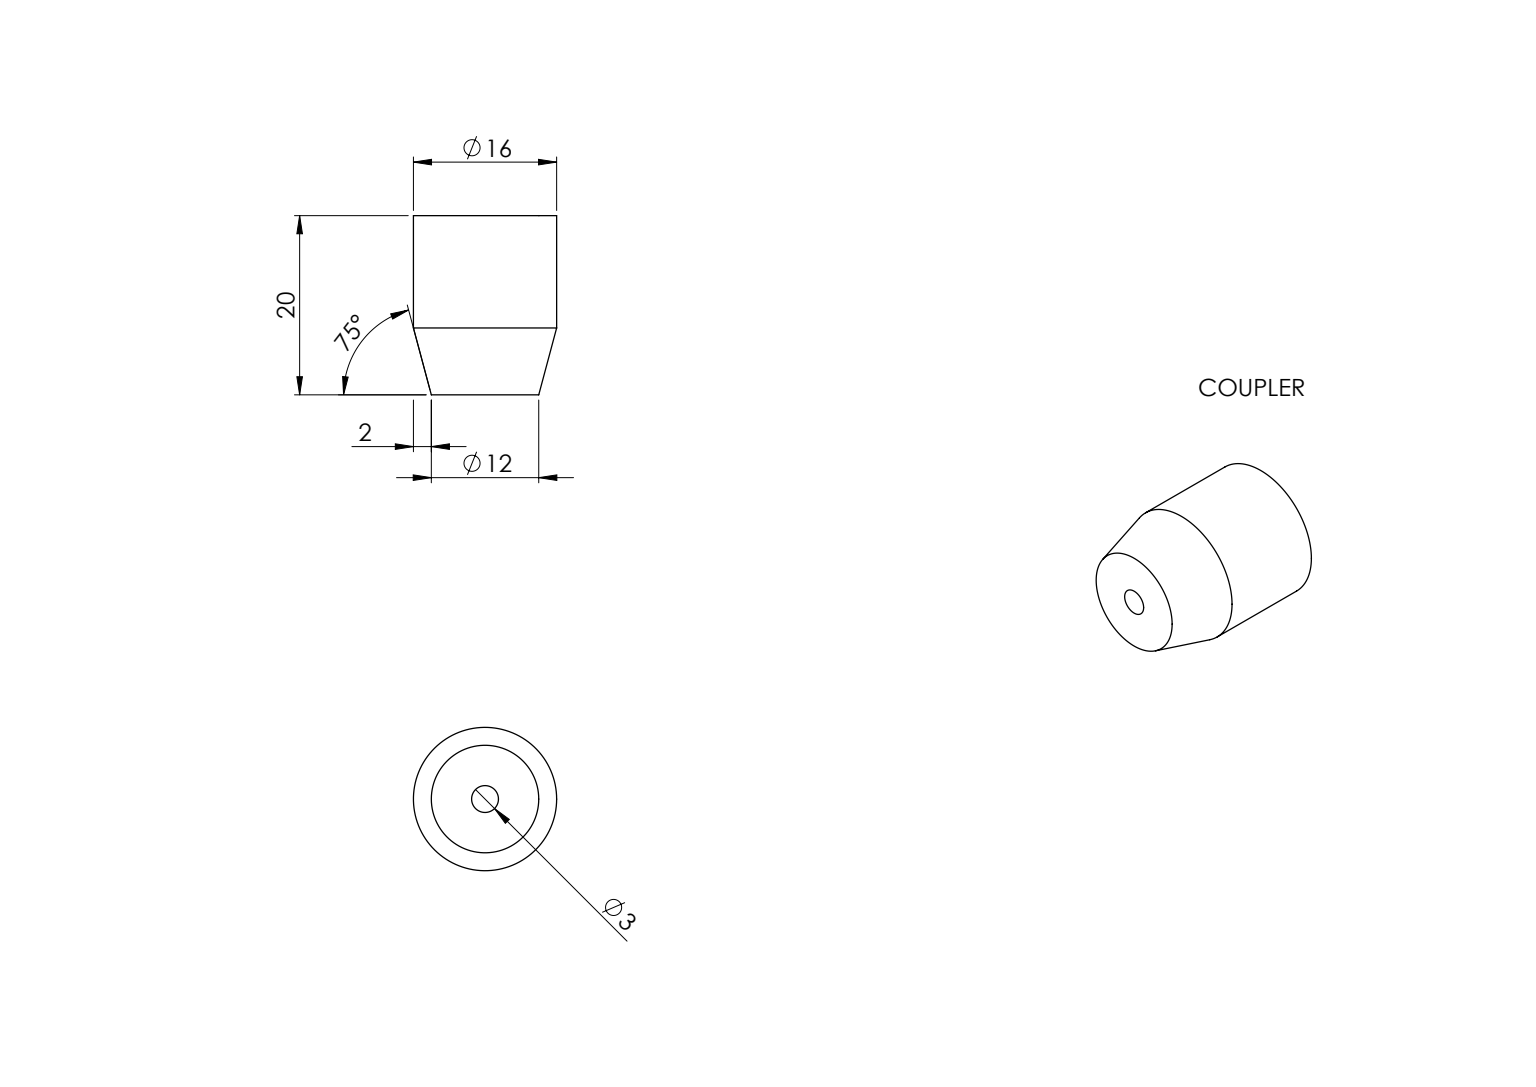
ISO-10303-21;
HEADER;
FILE_DESCRIPTION (('STEP AP214'),
    '1' );
FILE_NAME ('coupler.step',
    '2026-10-31T03:36:27',
    ( '' ),
    ( '' ),
    'SwSTEP 2.0',
    'SolidWorks 2026',
    '' );
FILE_SCHEMA (( 'AUTOMOTIVE_DESIGN' ));
ENDSEC;

DATA;
#7=CARTESIAN_POINT ( 'NONE',  ( 10.56230152254411081, 0.000000000000000000, -0.3374999987710014526 ) ) ;
#8=DIRECTION ( 'NONE',  ( -1.000000000000000000, 0.000000000000000000, 0.000000000000000000 ) ) ;
#18=CARTESIAN_POINT ( 'NONE',  ( 19.68408634441911786, -5.407089921784861808, -9.046874999385529748 ) ) ;
#22=CARTESIAN_POINT ( 'NONE',  ( 13.44051670066911619, -5.407089921784865361, -3.721874999385532679 ) ) ;
#34=CARTESIAN_POINT ( 'NONE',  ( 16.56230152254410726, 0.000000000000000000, -10.00000000000000000 ) ) ;
#40=CARTESIAN_POINT ( 'NONE',  ( 13.56230152254411792, -5.196152422706638241, -4.875000000000101252 ) ) ;
#43=LINE ( 'NONE', #12559, #36906 ) ;
#57=CARTESIAN_POINT ( 'NONE',  ( 13.44051670066911441, -5.407089921784865361, -1.021874999385524729 ) ) ;
#68=CARTESIAN_POINT ( 'NONE',  ( 10.56230152254517307, 3.464101615138364565, -6.224999998771024501 ) ) ;
#79=EDGE_CURVE ( 'NONE', #19909, #6556, #23186, .T. ) ;
#81=CARTESIAN_POINT ( 'NONE',  ( 10.56230152254410726, 0.000000000000000000, -4.387499998770999277 ) ) ;
#94=CARTESIAN_POINT ( 'NONE',  ( 10.31873187879411269, 0.000000000000000000, -10.04062499938554431 ) ) ;
#97=CARTESIAN_POINT ( 'NONE',  ( 11.28998163430637725, -3.344369132205555317, -9.999999999999998224 ) ) ;
#108=CARTESIAN_POINT ( 'NONE',  ( 22.80587116629411781, -3.604726614523235284, -3.553124999385526728 ) ) ;
#125=CARTESIAN_POINT ( 'NONE',  ( 16.56230152254410726, 0.000000000000000000, -10.00000000000000000 ) ) ;
#128=EDGE_CURVE ( 'NONE', #11418, #35635, #36670, .T. ) ;
#135=ADVANCED_FACE ( 'NONE', ( #36144 ), #26701, .T. ) ;
#136=EDGE_LOOP ( 'NONE', ( #21590, #33549, #31769, #19071 ) ) ;
#142=CARTESIAN_POINT ( 'NONE',  ( 13.44051670066910908, 5.407089921784862696, -9.721874999385510918 ) ) ;
#155=LINE ( 'NONE', #26123, #10199 ) ;
#162=ORIENTED_EDGE ( 'NONE', *, *, #30521, .T. ) ;
#172=CARTESIAN_POINT ( 'NONE',  ( 19.68408634441911076, 5.407089921784857367, -4.790624999385539873 ) ) ;
#179=CARTESIAN_POINT ( 'NONE',  ( 10.56230152254411259, 3.464101615137752166, -4.874999998771025744 ) ) ;
#195=EDGE_CURVE ( 'NONE', #23387, #15078, #25492, .T. ) ;
#201=SHAPE_REPRESENTATION ( 'coupler', ( #17215 ), #24466 ) ;
#205=VERTEX_POINT ( 'NONE', #8495 ) ;
#208=CARTESIAN_POINT ( 'NONE',  ( 16.56230152254411436, 7.209453229046482114, -8.859374999385529748 ) ) ;
#213=CARTESIAN_POINT ( 'NONE',  ( 19.68408634441912142, -5.407089921784861808, -3.646874999385540939 ) ) ;
#222=EDGE_LOOP ( 'NONE', ( #9327, #12339, #21719, #21080 ) ) ;
#231=CARTESIAN_POINT ( 'NONE',  ( 10.56230152254410726, 0.000000000000000000, -3.600000000000047606 ) ) ;
#247=CARTESIAN_POINT ( 'NONE',  ( 19.68408634441911076, 5.407089921784862696, -2.146874999385511629 ) ) ;
#279=CARTESIAN_POINT ( 'NONE',  ( 22.80587116629410716, 7.646167579472015790E-16, -9.365624999385563143 ) ) ;
#285=DIRECTION ( 'NONE',  ( 1.000000000000000000, 0.000000000000000000, 0.000000000000000000 ) ) ;
#292=CARTESIAN_POINT ( 'NONE',  ( 10.31873187879411269, 3.604726614523236616, -4.228124999385536320 ) ) ;
#313=AXIS2_PLACEMENT_3D ( 'NONE', #22514, #37081, #34061 ) ;
#319=EDGE_LOOP ( 'NONE', ( #2535, #440, #17456, #4187 ) ) ;
#326=CARTESIAN_POINT ( 'NONE',  ( 13.44051670066911264, -5.407089921784865361, -10.02187499938553294 ) ) ;
#328=CARTESIAN_POINT ( 'NONE',  ( 13.44051670066911441, 5.407089921784856479, -2.915624999385552307 ) ) ;
#342=CARTESIAN_POINT ( 'NONE',  ( 10.56230152254331323, 3.464101615137297419, -9.037500000000031619 ) ) ;
#359=CARTESIAN_POINT ( 'NONE',  ( 22.80587116629411071, 3.604726614523238837, -5.728124999385511451 ) ) ;
#364=CARTESIAN_POINT ( 'NONE',  ( 10.56230152254410726, 0.000000000000000000, -4.387499998770999277 ) ) ;
#383=CARTESIAN_POINT ( 'NONE',  ( 22.56230152254385501, 3.464101615137912926, -7.837500000000038547 ) ) ;
#386=CARTESIAN_POINT ( 'NONE',  ( 22.56230152254410370, 0.000000000000000000, -10.00000000000000000 ) ) ;
#389=ORIENTED_EDGE ( 'NONE', *, *, #10539, .F. ) ;
#395=ORIENTED_EDGE ( 'NONE', *, *, #6389, .F. ) ;
#396=CARTESIAN_POINT ( 'NONE',  ( 10.31873187879411269, 3.604726614523240613, -4.284374999385516247 ) ) ;
#415=CARTESIAN_POINT ( 'NONE',  ( 16.56230152254411081, 6.928203230275514990, -3.712500000000020339 ) ) ;
#418=CARTESIAN_POINT ( 'NONE',  ( 10.56230152254458865, 3.464101615138028389, -5.324999998771027698 ) ) ;
#434=CARTESIAN_POINT ( 'NONE',  ( 10.31873187879410736, 3.604726614523240613, -1.584374999385509630 ) ) ;
#440=ORIENTED_EDGE ( 'NONE', *, *, #16671, .T. ) ;
#453=LINE ( 'NONE', #37417, #32490 ) ;
#457=CARTESIAN_POINT ( 'NONE',  ( 10.56230152254384080, 3.464101615137603396, -9.937499999999992895 ) ) ;
#464=DIRECTION ( 'NONE',  ( 0.000000000000000000, 0.000000000000000000, 1.000000000000000000 ) ) ;
#465=CARTESIAN_POINT ( 'NONE',  ( 10.31873187879411091, -3.604726614523240613, -8.653124999385532590 ) ) ;
#478=CARTESIAN_POINT ( 'NONE',  ( 10.31873187879411091, -3.604726614523240613, -5.053124999385533833 ) ) ;
#495=DIRECTION ( 'NONE',  ( 1.000000000000000000, 0.000000000000000000, 0.000000000000000000 ) ) ;
#501=CARTESIAN_POINT ( 'NONE',  ( 22.56230152254543597, 3.464101615136989665, -4.574999998771033916 ) ) ;
#510=CARTESIAN_POINT ( 'NONE',  ( 13.44051670066911441, -5.407089921784859143, -1.865624999385528948 ) ) ;
#514=DIRECTION ( 'NONE',  ( 1.000000000000000000, 0.000000000000000000, -0.000000000000000000 ) ) ;
#524=FACE_OUTER_BOUND ( 'NONE', #7081, .T. ) ;
#537=( BOUNDED_CURVE ( )  B_SPLINE_CURVE ( 2, ( #9361, #68, #20936, #11634, #17898, #12007, #35307 ),
 .UNSPECIFIED., .F., .F. ) 
 B_SPLINE_CURVE_WITH_KNOTS ( ( 3, 2, 2, 3 ),
 ( 0.5652173913043500031, 0.5724637681159433500, 0.5797101449275368079, 0.5869565217391301548 ),
 .UNSPECIFIED. ) 
 CURVE ( )  GEOMETRIC_REPRESENTATION_ITEM ( )  RATIONAL_B_SPLINE_CURVE ( ( 0.9999999999999589217, 0.8660254037844797859, 1.000000000000000000, 0.8660254037844387076, 1.000000000000000000, 0.8660254037844448138, 0.9999999999999938938 ) ) 
 REPRESENTATION_ITEM ( '' )  );
#541=CARTESIAN_POINT ( 'NONE',  ( 10.31873187879411269, -3.604726614523240613, -4.603124999385506122 ) ) ;
#546=CARTESIAN_POINT ( 'NONE',  ( 13.56230152254410548, 5.196152422706630247, -5.812499998771008869 ) ) ;
#568=CARTESIAN_POINT ( 'NONE',  ( 22.80587116629411071, 3.604726614523238837, -0.7781249993855585689 ) ) ;
#571=ORIENTED_EDGE ( 'NONE', *, *, #36630, .T. ) ;
#578=CARTESIAN_POINT ( 'NONE',  ( 22.80587116629412492, 3.604726614523243278, -3.984374999385507987 ) ) ;
#579=EDGE_LOOP ( 'NONE', ( #18982, #34697, #20451, #16198 ) ) ;
#598=CARTESIAN_POINT ( 'NONE',  ( 13.56230152254411614, -5.196152422706638241, -5.775000000000085620 ) ) ;
#602=LINE ( 'NONE', #31703, #10891 ) ;
#606=CARTESIAN_POINT ( 'NONE',  ( 22.56625951594015689, -0.6522502533381772105, -10.00000000000000000 ) ) ;
#616=CARTESIAN_POINT ( 'NONE',  ( 19.68408634441911431, 5.407089921784862696, -0.7968749993855217539 ) ) ;
#639=CARTESIAN_POINT ( 'NONE',  ( 19.56230152254412147, 5.196152422706637353, -0.6000000000000171863 ) ) ;
#650=CARTESIAN_POINT ( 'NONE',  ( 10.31873187879411091, -3.604726614523240613, -9.553124999385522287 ) ) ;
#657=ORIENTED_EDGE ( 'NONE', *, *, #10356, .T. ) ;
#661=CARTESIAN_POINT ( 'NONE',  ( 13.44051670066911619, -5.407089921784859143, -5.015624999385570604 ) ) ;
#667=ORIENTED_EDGE ( 'NONE', *, *, #34152, .T. ) ;
#698=CARTESIAN_POINT ( 'NONE',  ( 19.68408634441910721, -5.407089921784855591, -1.790624999385564964 ) ) ;
#727=CARTESIAN_POINT ( 'NONE',  ( 22.80587116629410716, 7.646167579472015790E-16, -5.765624999385543958 ) ) ;
#735=CARTESIAN_POINT ( 'NONE',  ( 16.56230152254410726, -6.928203230275506996, -5.624999998770996434 ) ) ;
#740=CARTESIAN_POINT ( 'NONE',  ( 19.68408634441911786, -5.407089921784861808, -4.996874999385530813 ) ) ;
#742=CARTESIAN_POINT ( 'NONE',  ( 22.56230152254410015, 7.347880794884117764E-16, -7.312499998771010645 ) ) ;
#754=CARTESIAN_POINT ( 'NONE',  ( 16.56230152254411436, -6.928203230275514990, -4.837499999999994138 ) ) ;
#756=CARTESIAN_POINT ( 'NONE',  ( 22.56230152254500254, 3.464101615137234358, -5.924999998771016685 ) ) ;
#771=CARTESIAN_POINT ( 'NONE',  ( 10.31873187879410736, -3.604726614523244610, -3.309374999385498395 ) ) ;
#791=CARTESIAN_POINT ( 'NONE',  ( 13.56230152254410726, 5.196152422706636465, -6.375000000000019540 ) ) ;
#792=ORIENTED_EDGE ( 'NONE', *, *, #29984, .F. ) ;
#800=CARTESIAN_POINT ( 'NONE',  ( 10.56230152254594756, 3.464101615138813095, -1.274999998771018772 ) ) ;
#808=CARTESIAN_POINT ( 'NONE',  ( 22.80587116629411781, -3.604726614523238837, -4.509374999385530103 ) ) ;
#822=CARTESIAN_POINT ( 'NONE',  ( 19.68408634441910365, -5.407089921784855591, -0.8906249993855530622 ) ) ;
#831=CARTESIAN_POINT ( 'NONE',  ( 16.56230152254411436, 6.928203230275506996, -0.8999999987709939031 ) ) ;
#837=CARTESIAN_POINT ( 'NONE',  ( 21.95617849068234761, 3.814046910745170660, -9.967423460872726793 ) ) ;
#841=( BOUNDED_CURVE ( )  B_SPLINE_CURVE ( 2, ( #13122, #26953, #12745, #33021, #24313, #35856, #23936 ),
 .UNSPECIFIED., .F., .F. ) 
 B_SPLINE_CURVE_WITH_KNOTS ( ( 3, 2, 2, 3 ),
 ( 0.5434782608695670758, 0.5507246376811614219, 0.5579710144927557680, 0.5652173913043500031 ),
 .UNSPECIFIED. ) 
 CURVE ( )  GEOMETRIC_REPRESENTATION_ITEM ( )  RATIONAL_B_SPLINE_CURVE ( ( 0.9999999999999651390, 0.8660254037844735686, 1.000000000000000000, 0.8660254037844387076, 1.000000000000000000, 0.8660254037843976294, 1.000000000000041078 ) ) 
 REPRESENTATION_ITEM ( '' )  );
#853=DIRECTION ( 'NONE',  ( 0.000000000000000000, 0.000000000000000000, 1.000000000000000000 ) ) ;
#854=CARTESIAN_POINT ( 'NONE',  ( 13.44051670066911086, 5.407089921784856479, -6.965624999385521932 ) ) ;
#856=LINE ( 'NONE', #4264, #19603 ) ;
#861=ORIENTED_EDGE ( 'NONE', *, *, #9647, .T. ) ;
#863=DIRECTION ( 'NONE',  ( 0.000000000000000000, 0.000000000000000000, 1.000000000000000000 ) ) ;
#868=CARTESIAN_POINT ( 'NONE',  ( 10.56230152254410726, 0.000000000000000000, -5.850000000000049383 ) ) ;
#890=CARTESIAN_POINT ( 'NONE',  ( 13.44051670066911264, -5.407089921784859143, -2.765624999385540850 ) ) ;
#901=CARTESIAN_POINT ( 'NONE',  ( 10.56230152254374310, -3.464101615137546109, -6.712500000000007461 ) ) ;
#912=EDGE_LOOP ( 'NONE', ( #20316, #5565, #15559, #5000 ) ) ;
#923=CARTESIAN_POINT ( 'NONE',  ( 13.44051670066911086, 5.407089921784856479, -4.715624999385548577 ) ) ;
#929=CARTESIAN_POINT ( 'NONE',  ( 16.56230152254411081, -6.928203230275506996, -5.174999998771001586 ) ) ;
#932=AXIS2_PLACEMENT_3D ( 'NONE', #8550, #25977, #8 ) ;
#933=CARTESIAN_POINT ( 'NONE',  ( 16.56230152254411436, 7.209453229046482114, -4.809374999385505944 ) ) ;
#945=CARTESIAN_POINT ( 'NONE',  ( 10.56230152254410726, 0.000000000000000000, -7.650000000000045652 ) ) ;
#960=CARTESIAN_POINT ( 'NONE',  ( 22.80587116629411426, 7.646167579472024665E-16, -6.721874999385535787 ) ) ;
#968=CARTESIAN_POINT ( 'NONE',  ( 22.56230152254411792, 7.347880794884125653E-16, -5.625000000000018652 ) ) ;
#975=AXIS2_PLACEMENT_3D ( 'NONE', #33240, #22432, #7279 ) ;
#979=CARTESIAN_POINT ( 'NONE',  ( 22.56230152254412502, -3.464101615137755275, -7.012500000000041922 ) ) ;
#983=CARTESIAN_POINT ( 'NONE',  ( 22.56230152254410726, 7.347880794884117764E-16, -9.562499998771039955 ) ) ;
#988=CARTESIAN_POINT ( 'NONE',  ( 22.39561461052787195, -1.640876061562029031, -9.999999999999998224 ) ) ;
#990=DIRECTION ( 'NONE',  ( 1.000000000000000000, 0.000000000000000000, 0.000000000000000000 ) ) ;
#996=CARTESIAN_POINT ( 'NONE',  ( 19.68408634441912142, -5.407089921784861808, -2.746874999385529037 ) ) ;
#1037=ORIENTED_EDGE ( 'NONE', *, *, #23070, .T. ) ;
#1041=CARTESIAN_POINT ( 'NONE',  ( 22.80587116629411071, 3.604726614523238837, -6.178124999385540050 ) ) ;
#1049=CARTESIAN_POINT ( 'NONE',  ( 16.56230152254411436, -6.928203230275514990, -3.937500000000034639 ) ) ;
#1055=CARTESIAN_POINT ( 'NONE',  ( 13.56230152254410370, 5.196152422706630247, -4.912499998770996967 ) ) ;
#1079=CARTESIAN_POINT ( 'NONE',  ( 22.80587116629410716, 7.646167579472015790E-16, -3.965624999385547689 ) ) ;
#1088=ORIENTED_EDGE ( 'NONE', *, *, #15863, .T. ) ;
#1111=CARTESIAN_POINT ( 'NONE',  ( 19.68408634441910721, -5.407089921784855591, -8.090624999385564564 ) ) ;
#1118=CARTESIAN_POINT ( 'NONE',  ( 10.56230152254411614, -3.464101615137757051, -6.149999998770987020 ) ) ;
#1119=CARTESIAN_POINT ( 'NONE',  ( 10.56230152254410903, 7.347880794884117764E-16, -10.00000000000000000 ) ) ;
#1121=CARTESIAN_POINT ( 'NONE',  ( 10.31873187879410736, 0.000000000000000000, -3.346874999385518468 ) ) ;
#1134=CARTESIAN_POINT ( 'NONE',  ( 10.56230152254490484, 3.464101615138212242, -5.774999998771026988 ) ) ;
#1149=CARTESIAN_POINT ( 'NONE',  ( 16.56230152254411792, -7.209453229046482114, -5.484374999385515537 ) ) ;
#1154=EDGE_CURVE ( 'NONE', #28711, #31946, #29357, .T. ) ;
#1169=CARTESIAN_POINT ( 'NONE',  ( 22.56230152254411792, 7.347880794884125653E-16, -7.425000000000042455 ) ) ;
#1184=CARTESIAN_POINT ( 'NONE',  ( 19.68408634441910721, 5.407089921784862696, -3.046874999385523530 ) ) ;
#1201=CARTESIAN_POINT ( 'NONE',  ( 22.56230152254410370, 7.347880794884117764E-16, -1.012499998771038134 ) ) ;
#1213=CARTESIAN_POINT ( 'NONE',  ( 22.56230152254411792, 7.347880794884125653E-16, -2.475000000000060485 ) ) ;
#1225=CARTESIAN_POINT ( 'NONE',  ( 13.44051670066911619, -5.407089921784859143, -6.815624999385539340 ) ) ;
#1250=ADVANCED_FACE ( 'NONE', ( #23225 ), #9190, .F. ) ;
#1263=CARTESIAN_POINT ( 'NONE',  ( 22.80587116629410716, 7.646167579472015790E-16, -4.415624999385525662 ) ) ;
#1265=CARTESIAN_POINT ( 'NONE',  ( 16.56230152254410726, 0.000000000000000000, 10.00000000000000000 ) ) ;
#1272=CARTESIAN_POINT ( 'NONE',  ( 16.56230152254410726, 0.000000000000000000, 10.00000000000000000 ) ) ;
#1287=CARTESIAN_POINT ( 'NONE',  ( 22.56230152254410726, 7.347880794884117764E-16, -9.112499998771033560 ) ) ;
#1288=EDGE_CURVE ( 'NONE', #21775, #13344, #22888, .T. ) ;
#1296=CARTESIAN_POINT ( 'NONE',  ( 19.68408634441910721, 5.407089921784857367, -8.390624999385531524 ) ) ;
#1297=( BOUNDED_CURVE ( )  B_SPLINE_CURVE ( 2, ( #36397, #25222, #16702, #28423, #36212, #7793, #8169 ),
 .UNSPECIFIED., .F., .F. ) 
 B_SPLINE_CURVE_WITH_KNOTS ( ( 3, 2, 2, 3 ),
 ( 0.2173913043478289675, 0.2246376811594223422, 0.2318840579710157446, 0.2391304347826091192 ),
 .UNSPECIFIED. ) 
 CURVE ( )  GEOMETRIC_REPRESENTATION_ITEM ( )  RATIONAL_B_SPLINE_CURVE ( ( 0.9999999999999465983, 0.8660254037844921093, 1.000000000000000000, 0.8660254037844387076, 1.000000000000000000, 0.8660254037844310471, 1.000000000000007772 ) ) 
 REPRESENTATION_ITEM ( '' )  );
#1301=CIRCLE ( 'NONE', #23716, 5.999999999999998224 ) ;
#1303=CARTESIAN_POINT ( 'NONE',  ( 22.56230152254410015, 7.347880794884117764E-16, -7.762499998770988618 ) ) ;
#1308=CARTESIAN_POINT ( 'NONE',  ( 22.80587116629411781, -3.604726614523238837, -4.509374999385530103 ) ) ;
#1327=CARTESIAN_POINT ( 'NONE',  ( 16.56230152254410726, -7.209453229046475009, -3.178124999385525395 ) ) ;
#1339=CARTESIAN_POINT ( 'NONE',  ( 16.56230152254411081, 7.209453229046482114, -5.709374999385496530 ) ) ;
#1340=VERTEX_POINT ( 'NONE', #32484 ) ;
#1346=( NAMED_UNIT ( * ) SI_UNIT ( $, .STERADIAN. ) SOLID_ANGLE_UNIT ( ) );
#1361=CARTESIAN_POINT ( 'NONE',  ( 16.56230152254411436, -6.928203230275514990, -7.987500000000027356 ) ) ;
#1363=ORIENTED_EDGE ( 'NONE', *, *, #4409, .T. ) ;
#1378=CARTESIAN_POINT ( 'NONE',  ( 19.68408634441911431, 5.407089921784862696, -4.846874999385547333 ) ) ;
#1392=CARTESIAN_POINT ( 'NONE',  ( 16.56230152254410726, 0.000000000000000000, 0.000000000000000000 ) ) ;
#1399=CARTESIAN_POINT ( 'NONE',  ( 13.56230152254410903, 5.196152422706636465, -0.5250000000000532019 ) ) ;
#1404=CARTESIAN_POINT ( 'NONE',  ( 16.56230152254411081, 6.928203230275506996, -8.549999998770985599 ) ) ;
#1415=CARTESIAN_POINT ( 'NONE',  ( 10.31873187879411091, 0.000000000000000000, -7.340624999385508609 ) ) ;
#1455=CARTESIAN_POINT ( 'NONE',  ( 16.56230152254411081, 7.209453229046475009, -3.403124999385538807 ) ) ;
#1457=LINE ( 'NONE', #35951, #26756 ) ;
#1460=CARTESIAN_POINT ( 'NONE',  ( 15.26155779561005232, -6.106572496351636126, -10.00000000000000000 ) ) ;
#1486=CARTESIAN_POINT ( 'NONE',  ( 10.31873187879411091, 3.604726614523236616, -7.828124999385534188 ) ) ;
#1491=CARTESIAN_POINT ( 'NONE',  ( 22.56230152254410370, 7.347880794884117764E-16, -8.662499998771028942 ) ) ;
#1494=CARTESIAN_POINT ( 'NONE',  ( 22.80587116629412847, -3.604726614523238837, -5.409374999385520688 ) ) ;
#1522=ORIENTED_EDGE ( 'NONE', *, *, #16803, .T. ) ;
#1523=CARTESIAN_POINT ( 'NONE',  ( 13.44051670066910908, 5.407089921784862696, -7.021874999385530280 ) ) ;
#1527=CARTESIAN_POINT ( 'NONE',  ( 19.68408634441910721, 5.407089921784857367, -1.190624999385520022 ) ) ;
#1532=CARTESIAN_POINT ( 'NONE',  ( 19.56230152254411081, -5.196152422706629359, -9.637499998771032139 ) ) ;
#1536=CARTESIAN_POINT ( 'NONE',  ( 10.56230152254410903, 0.000000000000000000, -1.237499998771041110 ) ) ;
#1537=ORIENTED_EDGE ( 'NONE', *, *, #3843, .T. ) ;
#1546=CARTESIAN_POINT ( 'NONE',  ( 13.56230152254411792, -5.196152422706638241, -9.375000000000078160 ) ) ;
#1561=CARTESIAN_POINT ( 'NONE',  ( 10.31873187879410736, 0.000000000000000000, -5.596874999385520688 ) ) ;
#1588=CARTESIAN_POINT ( 'NONE',  ( 16.56230152254411436, 6.928203230275514990, -3.262500000000057021 ) ) ;
#1606=CARTESIAN_POINT ( 'NONE',  ( 10.31873187879410736, 0.000000000000000000, -6.890624999385530636 ) ) ;
#1608=CARTESIAN_POINT ( 'NONE',  ( 13.56230152254411259, -5.196152422706632912, -2.512499998771011711 ) ) ;
#1613=ORIENTED_EDGE ( 'NONE', *, *, #16584, .F. ) ;
#1625=DIRECTION ( 'NONE',  ( 0.000000000000000000, 0.000000000000000000, 1.000000000000000000 ) ) ;
#1645=CARTESIAN_POINT ( 'NONE',  ( 13.44051670066911086, 5.407089921784856479, -4.715624999385548577 ) ) ;
#1649=CARTESIAN_POINT ( 'NONE',  ( 19.68408634441911786, -5.407089921784861808, -9.496874999385534366 ) ) ;
#1654=CARTESIAN_POINT ( 'NONE',  ( 10.31873187879410381, 3.604726614523240613, -0.2343749993854903346 ) ) ;
#1656=ORIENTED_EDGE ( 'NONE', *, *, #14505, .T. ) ;
#1661=DIRECTION ( 'NONE',  ( 1.000000000000000000, 0.000000000000000000, 0.000000000000000000 ) ) ;
#1675=CARTESIAN_POINT ( 'NONE',  ( 19.68408634441910721, -5.407089921784855591, -8.990624999385548932 ) ) ;
#1680=CARTESIAN_POINT ( 'NONE',  ( 22.56230152254409660, 3.464101615137755275, -9.074999998770975296 ) ) ;
#1683=CARTESIAN_POINT ( 'NONE',  ( 13.44051670066911264, -5.407089921784865361, -5.521874999385528504 ) ) ;
#1696=CARTESIAN_POINT ( 'NONE',  ( 22.56230152254410726, 7.347880794884117764E-16, -9.112499998771033560 ) ) ;
#1708=CARTESIAN_POINT ( 'NONE',  ( 22.56230152254403265, -3.464101615137814338, -0.2625000000000441980 ) ) ;
#1712=CARTESIAN_POINT ( 'NONE',  ( 13.44051670066911086, 5.407089921784862696, -5.671874999385540406 ) ) ;
#1721=( NAMED_UNIT ( * ) PLANE_ANGLE_UNIT ( ) SI_UNIT ( $, .RADIAN. ) );
#1722=CARTESIAN_POINT ( 'NONE',  ( 22.56230152254410015, 7.347880794884117764E-16, -2.812499998771006204 ) ) ;
#1725=CARTESIAN_POINT ( 'NONE',  ( 22.56230152254410015, 3.464101615137755275, -0.5249999987710241012 ) ) ;
#1729=CARTESIAN_POINT ( 'NONE',  ( 10.56230152254411081, 0.000000000000000000, -4.837499998771033205 ) ) ;
#1733=CARTESIAN_POINT ( 'NONE',  ( 19.56230152254412147, -5.196152422706635576, -9.300000000000057554 ) ) ;
#1752=CARTESIAN_POINT ( 'NONE',  ( 13.44051670066910908, 5.407089921784862696, -7.021874999385530280 ) ) ;
#1756=EDGE_LOOP ( 'NONE', ( #2378, #1797, #29965, #24577 ) ) ;
#1775=CARTESIAN_POINT ( 'NONE',  ( 10.56230152254411614, -3.464101615137761048, -1.312500000000054401 ) ) ;
#1783=DIRECTION ( 'NONE',  ( 0.000000000000000000, 0.000000000000000000, 1.000000000000000000 ) ) ;
#1793=CARTESIAN_POINT ( 'NONE',  ( 19.68408634441910721, 5.407089921784857367, -8.390624999385531524 ) ) ;
#1797=ORIENTED_EDGE ( 'NONE', *, *, #17252, .T. ) ;
#1829=CARTESIAN_POINT ( 'NONE',  ( 10.31873187879411091, -3.604726614523240613, -5.053124999385533833 ) ) ;
#1839=CARTESIAN_POINT ( 'NONE',  ( 13.44051670066910908, 5.407089921784862696, -2.071874999385547866 ) ) ;
#1847=EDGE_CURVE ( 'NONE', #16024, #17042, #30597, .T. ) ;
#1860=CARTESIAN_POINT ( 'NONE',  ( 13.44051670066911264, 5.407089921784856479, -8.315624999385541116 ) ) ;
#1865=CARTESIAN_POINT ( 'NONE',  ( 22.56230152254410015, 7.347880794884117764E-16, -8.212499998771022547 ) ) ;
#1866=( BOUNDED_CURVE ( )  B_SPLINE_CURVE ( 2, ( #29614, #800, #33026, #3650, #4213, #18453, #15219 ),
 .UNSPECIFIED., .F., .F. ) 
 B_SPLINE_CURVE_WITH_KNOTS ( ( 3, 2, 2, 3 ),
 ( 0.08695652173913427652, 0.09420289855072766505, 0.1014492753623210397, 0.1086956521739144144 ),
 .UNSPECIFIED. ) 
 CURVE ( )  GEOMETRIC_REPRESENTATION_ITEM ( )  RATIONAL_B_SPLINE_CURVE ( ( 0.9999999999999289457, 0.8660254037845097619, 1.000000000000000000, 0.8660254037844387076, 1.000000000000000000, 0.8660254037844132835, 1.000000000000025313 ) ) 
 REPRESENTATION_ITEM ( '' )  );
#1870=CARTESIAN_POINT ( 'NONE',  ( 13.44051670066911264, -5.407089921784865361, -5.971874999385562433 ) ) ;
#1874=CYLINDRICAL_SURFACE ( 'NONE', #4361, 1.500000000000001332 ) ;
#1877=DIRECTION ( 'NONE',  ( 0.000000000000000000, 0.000000000000000000, 1.000000000000000000 ) ) ;
#1899=CARTESIAN_POINT ( 'NONE',  ( 22.80587116629412492, -3.604726614523238837, -7.659374999385499372 ) ) ;
#1900=ORIENTED_EDGE ( 'NONE', *, *, #29749, .F. ) ;
#1910=CARTESIAN_POINT ( 'NONE',  ( 16.56230152254411436, 6.928203230275506996, -0.4499999987709982219 ) ) ;
#1917=CARTESIAN_POINT ( 'NONE',  ( 22.56230152254412147, -3.464101615137755275, -9.712500000000016342 ) ) ;
#1924=CYLINDRICAL_SURFACE ( 'NONE', #15961, 5.999999999999998224 ) ;
#1934=CARTESIAN_POINT ( 'NONE',  ( 19.68408634441911431, -5.407089921784861808, -6.346874999385549110 ) ) ;
#1939=CARTESIAN_POINT ( 'NONE',  ( 19.68408634441911431, -5.407089921784861808, -0.4968749993855270386 ) ) ;
#1943=PRODUCT_CONTEXT ( 'NONE', #19027, 'mechanical' ) ;
#1958=CARTESIAN_POINT ( 'NONE',  ( 13.56230152254410726, 5.196152422706636465, -1.875000000000043299 ) ) ;
#1971=ORIENTED_EDGE ( 'NONE', *, *, #25981, .F. ) ;
#1972=CARTESIAN_POINT ( 'NONE',  ( 22.56230152254492438, -3.464101615137295642, -7.012500000000033040 ) ) ;
#1976=CARTESIAN_POINT ( 'NONE',  ( 13.44051670066911619, -5.407089921784859143, -9.515624999385547511 ) ) ;
#1986=DIRECTION ( 'NONE',  ( 0.000000000000000000, 0.000000000000000000, 1.000000000000000000 ) ) ;
#2009=DIRECTION ( 'NONE',  ( 0.000000000000000000, 0.000000000000000000, 1.000000000000000000 ) ) ;
#2014=CARTESIAN_POINT ( 'NONE',  ( 22.80587116629410360, 7.646167579472015790E-16, -7.115624999385533833 ) ) ;
#2020=CARTESIAN_POINT ( 'NONE',  ( 10.56230152254410548, 0.000000000000000000, -6.750000000000061284 ) ) ;
#2022=CARTESIAN_POINT ( 'NONE',  ( 22.80587116629411426, 7.646167579472024665E-16, -1.771874999385525395 ) ) ;
#2029=CARTESIAN_POINT ( 'NONE',  ( 19.68408634441910365, -5.407089921784855591, -0.8906249993855530622 ) ) ;
#2046=CARTESIAN_POINT ( 'NONE',  ( 16.56230152254411436, -7.209453229046475009, -9.928124999385525840 ) ) ;
#2053=CARTESIAN_POINT ( 'NONE',  ( 22.56230152254409660, 3.464101615137755275, -9.524999998771003007 ) ) ;
#2057=CARTESIAN_POINT ( 'NONE',  ( 10.31873187879411091, 3.604726614523240613, -9.684374999385527261 ) ) ;
#2058=CARTESIAN_POINT ( 'NONE',  ( 22.80587116629411781, -3.604726614523238837, -7.209374999385536498 ) ) ;
#2074=CARTESIAN_POINT ( 'NONE',  ( 10.56230152254410903, 0.000000000000000000, -2.250000000000057732 ) ) ;
#2083=CYLINDRICAL_SURFACE ( 'NONE', #16524, 5.999999999999998224 ) ;
#2089=CARTESIAN_POINT ( 'NONE',  ( 22.80587116629411781, -3.604726614523238837, -8.109374999385527971 ) ) ;
#2099=CARTESIAN_POINT ( 'NONE',  ( 13.56230152254410548, 5.196152422706630247, -1.312499998771005094 ) ) ;
#2102=CARTESIAN_POINT ( 'NONE',  ( 16.56230152254411081, -6.928203230275514990, -8.887500000000020606 ) ) ;
#2106=CARTESIAN_POINT ( 'NONE',  ( 13.56230152254410548, 5.196152422706636465, -9.975000000000012079 ) ) ;
#2121=CARTESIAN_POINT ( 'NONE',  ( 16.56230152254411436, 7.209453229046482114, -5.259374999385500793 ) ) ;
#2127=CARTESIAN_POINT ( 'NONE',  ( 22.80587116629411781, 7.646167579472024665E-16, -0.4218749993855352987 ) ) ;
#2128=CARTESIAN_POINT ( 'NONE',  ( 10.56230152254410903, 0.000000000000000000, -5.737499998771017573 ) ) ;
#2144=CARTESIAN_POINT ( 'NONE',  ( 10.56230152254410726, 0.000000000000000000, -1.350000000000045608 ) ) ;
#2161=CARTESIAN_POINT ( 'NONE',  ( 19.68408634441910721, -5.407089921784855591, -9.440624999385555327 ) ) ;
#2165=EDGE_CURVE ( 'NONE', #205, #18251, #37105, .T. ) ;
#2168=ORIENTED_EDGE ( 'NONE', *, *, #25401, .F. ) ;
#2171=CARTESIAN_POINT ( 'NONE',  ( 22.56230152254410726, 7.347880794884117764E-16, -3.262499998771012599 ) ) ;
#2198=CARTESIAN_POINT ( 'NONE',  ( 19.68408634441910721, 5.407089921784857367, -5.690624999385579308 ) ) ;
#2207=CARTESIAN_POINT ( 'NONE',  ( 10.31873187879410736, -3.604726614523244610, -1.509374999385515670 ) ) ;
#2209=VERTEX_POINT ( 'NONE', #32966 ) ;
#2213=CARTESIAN_POINT ( 'NONE',  ( 16.56230152254411436, 7.209453229046475009, -2.053124999385520066 ) ) ;
#2218=EDGE_LOOP ( 'NONE', ( #26929, #14715, #15035, #29987 ) ) ;
#2232=CARTESIAN_POINT ( 'NONE',  ( 22.80587116629410716, 7.646167579472015790E-16, -9.365624999385563143 ) ) ;
#2238=CARTESIAN_POINT ( 'NONE',  ( 10.56230152254411259, -3.464101615137757051, -10.19999999877101082 ) ) ;
#2241=CARTESIAN_POINT ( 'NONE',  ( 10.31873187879411091, -3.604726614523244610, -9.609374999385535077 ) ) ;
#2242=CARTESIAN_POINT ( 'NONE',  ( 16.56230152254411436, -7.209453229046482114, -5.934374999385510385 ) ) ;
#2248=CYLINDRICAL_SURFACE ( 'NONE', #20898, 8.000000000000000000 ) ;
#2272=CARTESIAN_POINT ( 'NONE',  ( 22.80587116629412137, 7.646167579472024665E-16, -8.521874999385502747 ) ) ;
#2276=CARTESIAN_POINT ( 'NONE',  ( 13.44051670066911264, -5.407089921784859143, -2.765624999385540850 ) ) ;
#2282=CARTESIAN_POINT ( 'NONE',  ( 10.56230152254410903, 3.464101615137752166, -1.274999998770995679 ) ) ;
#2292=CARTESIAN_POINT ( 'NONE',  ( 19.68408634441910721, 5.407089921784857367, -0.2906249993855358760 ) ) ;
#2293=CYLINDRICAL_SURFACE ( 'NONE', #36650, 5.999999999999998224 ) ;
#2303=CARTESIAN_POINT ( 'NONE',  ( 22.56230152254390475, 3.464101615137881840, -3.787500000000044942 ) ) ;
#2311=CARTESIAN_POINT ( 'NONE',  ( 16.56230152254411436, 7.209453229046482114, -7.059374999385483740 ) ) ;
#2315=( BOUNDED_CURVE ( )  B_SPLINE_CURVE ( 2, ( #26791, #15432, #23962, #30909, #22012, #33566, #6519, #33750, #10623, #36582, #13286, #10250, #36206, #3671, #7417, #18988, #13100, #16511, #26981, #4562, #822, #35505, #16137, #19368, #22202, #24842, #28058, #15241, #1527, #32665, #13473, #36393, #25025, #7790, #6706, #10439, #24655, #18278, #7603, #30727, #16323, #18094, #29635, #9552, #29822, #28420, #3017, #17250, #20096, #37499, #16884, #26139, #34488, #36950, #25584, #11551, #22568, #10812, #31825, #31097, #22384, #8348, #5306, #23124, #33934, #37320, #7975, #22942, #16698, #31278, #2276, #20285, #11370, #8530, #14586, #34668, #8713, #25957, #2641, #37137, #11182, #28791, #28976, #5119, #19740, #2460, #5860, #31642, #28246, #19549, #34115, #19920, #5670, #2828, #28604, #13853, #14400, #25400, #10997, #17438, #8166, #14034, #14218, #22755, #34304, #31459, #25768, #5482, #17066, #23873, #26893, #20657, #26510, #21226, #15339, #29731, #15147, #35604, #32389, #541, #11923, #14963, #923, #23490, #172, #32766, #20473, #11739, #12492, #6429, #35041, #24059, #18190, #3765, #9650, #35412, #35227, #32012, #12107, #6802, #3202, #18003, #29546, #32204, #18377, #29927, #3955, #15530, #23309, #359, #727, #14778, #21038, #9276, #34855, #8895, #23680, #20848, #6043, #3584, #17629, #26697, #12299, #9462, #29159, #26322, #32575, #9088, #6239, #6615, #17816, #29354, #3394, #24433, #24617, #7193, #7743, #24799, #7006, #13249, #7561, #19327, #36538, #30864, #27270, #16282, #21972, #36164, #19136, #30118, #10581, #15910, #18576, #22160, #33704, #33335, #18946, #36350, #21600, #10019, #21784, #10395, #10210, #4889, #27086, #1486, #13060, #12678, #7375, #24977, #21412, #33149, #1111, #4148, #24248, #33517, #18764, #4703, #1860, #35792, #1296, #30684, #35983, #30500, #30306, #9834, #27830, #15720, #13429, #32954, #4521, #12867, #4330, #27458, #16095, #27648, #1675, #25542, #28013, #5440, #31781, #8669, #28561, #36728, #25728, #17022, #2232, #19695, #2418, #28382, #37094, #37281, #13812, #13991, #2602, #22898, #34625, #10767, #25359, #34073, #11510, #2046, #22339, #13625, #36904 ),
 .UNSPECIFIED., .F., .F. ) 
 B_SPLINE_CURVE_WITH_KNOTS ( ( 3, 2, 2, 2, 2, 2, 2, 2, 2, 2, 2, 2, 2, 2, 2, 2, 2, 2, 2, 2, 2, 2, 2, 2, 2, 2, 2, 2, 2, 2, 2, 2, 2, 2, 2, 2, 2, 2, 2, 2, 2, 2, 2, 2, 2, 2, 2, 2, 2, 2, 2, 2, 2, 2, 2, 2, 2, 2, 2, 2, 2, 2, 2, 2, 2, 2, 2, 2, 2, 2, 2, 2, 2, 2, 2, 2, 2, 2, 2, 2, 2, 2, 2, 2, 2, 2, 2, 2, 2, 2, 2, 2, 2, 2, 2, 2, 2, 2, 2, 2, 2, 2, 2, 2, 2, 2, 2, 2, 2, 2, 2, 2, 2, 2, 2, 2, 2, 2, 2, 2, 2, 2, 2, 2, 2, 2, 2, 2, 2, 2, 2, 2, 3 ),
 ( 0.000000000000000000, 0.007499808116169960973, 0.01499961623233992195, 0.02249942434850988118, 0.02999923246467984389, 0.03749904058084980313, 0.04499884869701976237, 0.05249865681318972854, 0.05999846492935968778, 0.06749827304552964702, 0.07499808116169960626, 0.08249788927786955162, 0.08999769739403952473, 0.09749750551020949785, 0.1049973136263794571, 0.1124971217425494163, 0.1199969298587193756, 0.1274967379748893348, 0.1349965460910592940, 0.1424963542072292533, 0.1499961623233992125, 0.1574959704395691995, 0.1649957785557391032, 0.1724955866719090902, 0.1799953947880790495, 0.1874952029042490087, 0.1949950110204189957, 0.2024948191365889549, 0.2099946272527589142, 0.2174944353689288457, 0.2249942434850988326, 0.2324940516012687641, 0.2399938597174387511, 0.2474936678336087381, 0.2549934759497786696, 0.2624932840659486288, 0.2699930921821185881, 0.2774929002982886028, 0.2849927084144585065, 0.2924925165306284103, 0.2999923246467984250, 0.3074921327629683843, 0.3149919408791383990, 0.3224917489953083582, 0.3299915571114782065, 0.3374913652276482212, 0.3449911733438181805, 0.3524909814599881952, 0.3599907895761580989, 0.3674905976923280582, 0.3749904058084980174, 0.3824902139246679766, 0.3899900220408379914, 0.3974898301570078951, 0.4049896382731779099, 0.4124894463893478136, 0.4199892545055178283, 0.4274890626216877321, 0.4349888707378576913, 0.4424886788540277061, 0.4499884869701976653, 0.4574882950863676245, 0.4649881032025375283, 0.4724879113187074875, 0.4799877194348775022, 0.4874875275510474615, 0.4949873356672174762, 0.5024871437833873244, 0.5099869518995573392, 0.5174867600157272429, 0.5249865681318972577, 0.5324863762480671614, 0.5399861843642371761, 0.5474859924804070799, 0.5549858005965772056, 0.5624856087127469983, 0.5699854168289170131, 0.5774852249450870278, 0.5849850330612568206, 0.5924848411774269463, 0.5999846492935968501, 0.6074844574097668648, 0.6149842655259367685, 0.6224840736421066723, 0.6299838817582767980, 0.6374836898744465907, 0.6449834979906167165, 0.6524833061067866202, 0.6599831142229564129, 0.6674829223391265387, 0.6749827304552964424, 0.6824825385714665682, 0.6899823466876363609, 0.6974821548038062646, 0.7049819629199763904, 0.7124817710361461831, 0.7199815791523161979, 0.7274813872684862126, 0.7349811953846561163, 0.7424810035008261311, 0.7499808116169960348, 0.7574806197331660496, 0.7649804278493359533, 0.7724802359655059680, 0.7799800440816759828, 0.7874798521978458865, 0.7949796603140157902, 0.8024794684301858050, 0.8099792765463558197, 0.8174790846625257235, 0.8249788927786956272, 0.8324787008948656419, 0.8399785090110356567, 0.8474783171272055604, 0.8549781252433754641, 0.8624779333595454789, 0.8699777414757153826, 0.8774775495918853974, 0.8849773577080554121, 0.8924771658242253158, 0.8999769739403953306, 0.9074767820565652343, 0.9149765901727352491, 0.9224763982889051528, 0.9299762064050750565, 0.9374760145212451823, 0.9449758226374149750, 0.9524756307535849897, 0.9599754388697550045, 0.9674752469859249082, 0.9749750551020949230, 0.9824748632182648267, 0.9859330816693211430 ),
 .UNSPECIFIED. ) 
 CURVE ( )  GEOMETRIC_REPRESENTATION_ITEM ( )  RATIONAL_B_SPLINE_CURVE ( ( 1.000000000000000000, 0.8660254037844387076, 1.000000000000000000, 0.8660254037844387076, 1.000000000000000000, 0.8660254037844387076, 1.000000000000000000, 0.8660254037844387076, 1.000000000000000000, 0.8660254037844387076, 1.000000000000000000, 0.8660254037844387076, 1.000000000000000000, 0.8660254037844387076, 1.000000000000000000, 0.8660254037844387076, 1.000000000000000000, 0.8660254037844387076, 1.000000000000000000, 0.8660254037844387076, 1.000000000000000000, 0.8660254037844387076, 1.000000000000000000, 0.8660254037844387076, 1.000000000000000000, 0.8660254037844387076, 1.000000000000000000, 0.8660254037844387076, 1.000000000000000000, 0.8660254037844387076, 1.000000000000000000, 0.8660254037844387076, 1.000000000000000000, 0.8660254037844387076, 1.000000000000000000, 0.8660254037844387076, 1.000000000000000000, 0.8660254037844387076, 1.000000000000000000, 0.8660254037844387076, 1.000000000000000000, 0.8660254037844387076, 1.000000000000000000, 0.8660254037844387076, 1.000000000000000000, 0.8660254037844387076, 1.000000000000000000, 0.8660254037844387076, 1.000000000000000000, 0.8660254037844387076, 1.000000000000000000, 0.8660254037844387076, 1.000000000000000000, 0.8660254037844387076, 1.000000000000000000, 0.8660254037844387076, 1.000000000000000000, 0.8660254037844387076, 1.000000000000000000, 0.8660254037844387076, 1.000000000000000000, 0.8660254037844387076, 1.000000000000000000, 0.8660254037844387076, 1.000000000000000000, 0.8660254037844387076, 1.000000000000000000, 0.8660254037844387076, 1.000000000000000000, 0.8660254037844387076, 1.000000000000000000, 0.8660254037844387076, 1.000000000000000000, 0.8660254037844387076, 1.000000000000000000, 0.8660254037844387076, 1.000000000000000000, 0.8660254037844387076, 1.000000000000000000, 0.8660254037844387076, 1.000000000000000000, 0.8660254037844387076, 1.000000000000000000, 0.8660254037844387076, 1.000000000000000000, 0.8660254037844387076, 1.000000000000000000, 0.8660254037844387076, 1.000000000000000000, 0.8660254037844387076, 1.000000000000000000, 0.8660254037844387076, 1.000000000000000000, 0.8660254037844387076, 1.000000000000000000, 0.8660254037844387076, 1.000000000000000000, 0.8660254037844387076, 1.000000000000000000, 0.8660254037844387076, 1.000000000000000000, 0.8660254037844387076, 1.000000000000000000, 0.8660254037844387076, 1.000000000000000000, 0.8660254037844387076, 1.000000000000000000, 0.8660254037844387076, 1.000000000000000000, 0.8660254037844387076, 1.000000000000000000, 0.8660254037844387076, 1.000000000000000000, 0.8660254037844387076, 1.000000000000000000, 0.8660254037844387076, 1.000000000000000000, 0.8660254037844387076, 1.000000000000000000, 0.8660254037844387076, 1.000000000000000000, 0.8660254037844387076, 1.000000000000000000, 0.8660254037844387076, 1.000000000000000000, 0.8660254037844387076, 1.000000000000000000, 0.8660254037844387076, 1.000000000000000000, 0.8660254037844387076, 1.000000000000000000, 0.8660254037844387076, 1.000000000000000000, 0.8660254037844387076, 1.000000000000000000, 0.8660254037844387076, 1.000000000000000000, 0.8660254037844387076, 1.000000000000000000, 0.8660254037844387076, 1.000000000000000000, 0.8660254037844387076, 1.000000000000000000, 0.8660254037844387076, 1.000000000000000000, 0.8660254037844387076, 1.000000000000000000, 0.8660254037844387076, 1.000000000000000000, 0.8660254037844387076, 1.000000000000000000, 0.8660254037844387076, 1.000000000000000000, 0.8660254037844387076, 1.000000000000000000, 0.8660254037844387076, 1.000000000000000000, 0.8660254037844387076, 1.000000000000000000, 0.8660254037844387076, 1.000000000000000000, 0.8660254037844387076, 1.000000000000000000, 0.8660254037844387076, 1.000000000000000000, 0.8660254037844387076, 1.000000000000000000, 0.8660254037844387076, 1.000000000000000000, 0.8660254037844387076, 1.000000000000000000, 0.8660254037844387076, 1.000000000000000000, 0.8660254037844387076, 1.000000000000000000, 0.8660254037844387076, 1.000000000000000000, 0.8660254037844387076, 1.000000000000000000, 0.8660254037844387076, 1.000000000000000000, 0.8660254037844387076, 1.000000000000000000, 0.8660254037844387076, 1.000000000000000000, 0.8660254037844387076, 1.000000000000000000, 0.8660254037844387076, 1.000000000000000000, 0.8660254037844387076, 1.000000000000000000, 0.8660254037844387076, 1.000000000000000000, 0.8660254037844387076, 1.000000000000000000, 0.8660254037844387076, 1.000000000000000000, 0.8660254037844387076, 1.000000000000000000, 0.8660254037844387076, 1.000000000000000000, 0.8660254037844387076, 1.000000000000000000, 0.8660254037844387076, 1.000000000000000000, 0.8660254037844387076, 1.000000000000000000, 0.8660254037844387076, 1.000000000000000000, 0.8660254037844387076, 1.000000000000000000, 0.8660254037844387076, 1.000000000000000000, 0.8660254037844387076, 1.000000000000000000, 0.8660254037844387076, 1.000000000000000000, 0.8660254037844387076, 1.000000000000000000, 0.8660254037844387076, 1.000000000000000000, 0.8660254037844387076, 1.000000000000000000, 0.8660254037844387076, 1.000000000000000000, 0.8660254037844387076, 1.000000000000000000, 0.8660254037844387076, 1.000000000000000000, 0.8660254037844387076, 1.000000000000000000, 0.8660254037844387076, 1.000000000000000000, 0.8660254037844387076, 1.000000000000000000, 0.8660254037844387076, 1.000000000000000000, 0.8660254037844387076, 1.000000000000000000, 0.8660254037844387076, 1.000000000000000000, 0.8660254037844387076, 1.000000000000000000, 0.8660254037844387076, 1.000000000000000000, 0.8660254037844387076, 1.000000000000000000, 0.8660254037844387076, 1.000000000000000000, 0.8660254037844387076, 1.000000000000000000, 0.8660254037844387076, 1.000000000000000000, 0.8660254037844387076, 1.000000000000000000, 0.8660254037844387076, 1.000000000000000000, 0.8660254037844387076, 1.000000000000000000, 0.8660254037844387076, 1.000000000000000000, 0.8660254037844387076, 1.000000000000000000, 0.9382232967258800072, 0.9334180070662969619 ) ) 
 REPRESENTATION_ITEM ( '' )  );
#2318=CARTESIAN_POINT ( 'NONE',  ( 10.31873187879410914, 0.000000000000000000, -2.446874999385534544 ) ) ;
#2324=CYLINDRICAL_SURFACE ( 'NONE', #23074, 8.000000000000000000 ) ;
#2336=CARTESIAN_POINT ( 'NONE',  ( 19.56230152254411792, 5.196152422706637353, -1.950000000000035039 ) ) ;
#2344=FACE_OUTER_BOUND ( 'NONE', #9960, .T. ) ;
#2353=CARTESIAN_POINT ( 'NONE',  ( 10.31873187879411091, -3.604726614523240613, -10.00312499938551802 ) ) ;
#2362=CARTESIAN_POINT ( 'NONE',  ( 10.56230152254410726, 0.000000000000000000, -0.9000000000000396572 ) ) ;
#2378=ORIENTED_EDGE ( 'NONE', *, *, #13301, .T. ) ;
#2386=CARTESIAN_POINT ( 'NONE',  ( 16.56230152254411081, 7.209453229046475009, -6.553124999385508964 ) ) ;
#2388=FACE_OUTER_BOUND ( 'NONE', #26406, .T. ) ;
#2395=CARTESIAN_POINT ( 'NONE',  ( 22.80587116629411781, 7.646167579472024665E-16, -0.8718749993855412495 ) ) ;
#2400=CARTESIAN_POINT ( 'NONE',  ( 22.80587116629410360, 7.646167579472015790E-16, -2.615624999385557370 ) ) ;
#2418=CARTESIAN_POINT ( 'NONE',  ( 19.68408634441910721, -5.407089921784855591, -9.440624999385555327 ) ) ;
#2428=CARTESIAN_POINT ( 'NONE',  ( 22.80587116629411071, 3.604726614523243278, -9.384374999385521221 ) ) ;
#2435=CARTESIAN_POINT ( 'NONE',  ( 19.56230152254410370, 5.196152422706631135, -3.637499998771026810 ) ) ;
#2436=VERTEX_POINT ( 'NONE', #9755 ) ;
#2457=CARTESIAN_POINT ( 'NONE',  ( 22.80587116629411426, 7.646167579472024665E-16, -7.621874999385519267 ) ) ;
#2460=CARTESIAN_POINT ( 'NONE',  ( 10.31873187879411091, 3.604726614523236616, -3.328124999385545291 ) ) ;
#2467=CARTESIAN_POINT ( 'NONE',  ( 19.56230152254410370, 5.196152422706631135, -3.637499998771026810 ) ) ;
#2471=CARTESIAN_POINT ( 'NONE',  ( 22.56230152254412147, 7.347880794884125653E-16, -8.775000000000032330 ) ) ;
#2477=CARTESIAN_POINT ( 'NONE',  ( 16.56230152254411081, -7.209453229046475009, -2.278124999385533478 ) ) ;
#2492=CARTESIAN_POINT ( 'NONE',  ( 22.80587116629411781, -3.604726614523238837, -8.109374999385527971 ) ) ;
#2497=CARTESIAN_POINT ( 'NONE',  ( 10.31873187879410203, 3.604726614523240613, -1.134374999385481697 ) ) ;
#2510=ORIENTED_EDGE ( 'NONE', *, *, #29857, .F. ) ;
#2520=CARTESIAN_POINT ( 'NONE',  ( 22.56230152254412502, -3.464101615137755275, -5.662500000000022737 ) ) ;
#2522=ORIENTED_EDGE ( 'NONE', *, *, #21319, .F. ) ;
#2535=ORIENTED_EDGE ( 'NONE', *, *, #13434, .T. ) ;
#2540=CARTESIAN_POINT ( 'NONE',  ( 13.44051670066911086, 5.407089921784856479, -9.215624999385523708 ) ) ;
#2542=CARTESIAN_POINT ( 'NONE',  ( 22.56230152254410370, 0.000000000000000000, -10.00000000000000000 ) ) ;
#2545=ORIENTED_EDGE ( 'NONE', *, *, #19779, .F. ) ;
#2549=CARTESIAN_POINT ( 'NONE',  ( 19.56230152254412502, -5.196152422706635576, -4.350000000000076028 ) ) ;
#2561=CARTESIAN_POINT ( 'NONE',  ( 19.56230152254411436, -5.196152422706629359, -4.237499998771044218 ) ) ;
#2568=CARTESIAN_POINT ( 'NONE',  ( 16.56230152254410726, 0.000000000000000000, -10.00000000000000000 ) ) ;
#2572=CARTESIAN_POINT ( 'NONE',  ( 22.80587116629410360, 7.646167579472015790E-16, -6.665624999385527438 ) ) ;
#2582=ORIENTED_EDGE ( 'NONE', *, *, #17982, .F. ) ;
#2586=CARTESIAN_POINT ( 'NONE',  ( 13.44051670066911441, 5.407089921784856479, -2.915624999385552307 ) ) ;
#2599=DIRECTION ( 'NONE',  ( 0.000000000000000000, 0.000000000000000000, 1.000000000000000000 ) ) ;
#2602=CARTESIAN_POINT ( 'NONE',  ( 13.44051670066911086, 5.407089921784856479, -9.665624999385530103 ) ) ;
#2611=CARTESIAN_POINT ( 'NONE',  ( 24.19849202207515404, 7.686353184319911769, -10.30110366105550135 ) ) ;
#2612=CARTESIAN_POINT ( 'NONE',  ( 16.56230152254411436, 7.209453229046482114, -9.759374999385554972 ) ) ;
#2615=CARTESIAN_POINT ( 'NONE',  ( 22.56230152254410370, 7.347880794884117764E-16, -1.012499998771038134 ) ) ;
#2633=CARTESIAN_POINT ( 'NONE',  ( 19.56230152254412502, -5.196152422706635576, -2.100000000000074252 ) ) ;
#2641=CARTESIAN_POINT ( 'NONE',  ( 22.80587116629410716, 7.646167579472015790E-16, -3.065624999385535787 ) ) ;
#2647=CARTESIAN_POINT ( 'NONE',  ( 16.56230152254410726, 6.928203230275506996, -3.599999998771000520 ) ) ;
#2657=CARTESIAN_POINT ( 'NONE',  ( 16.56230152254411436, 7.209453229046475009, -2.503124999385547778 ) ) ;
#2661=MECHANICAL_DESIGN_GEOMETRIC_PRESENTATION_REPRESENTATION('',(#35945),#19635);
#2666=FACE_OUTER_BOUND ( 'NONE', #17186, .T. ) ;
#2677=CARTESIAN_POINT ( 'NONE',  ( 10.31873187879410736, 0.000000000000000000, -8.296874999385501326 ) ) ;
#2681=CARTESIAN_POINT ( 'NONE',  ( 10.31873187879410736, -3.604726614523244610, -1.509374999385515670 ) ) ;
#2693=CARTESIAN_POINT ( 'NONE',  ( 22.56230152254411792, 7.347880794884125653E-16, -4.725000000000035172 ) ) ;
#2699=CARTESIAN_POINT ( 'NONE',  ( 10.56230152254410548, 0.000000000000000000, -4.050000000000054001 ) ) ;
#2700=VERTEX_POINT ( 'NONE', #28299 ) ;
#2717=CARTESIAN_POINT ( 'NONE',  ( 22.80587116629411781, -3.604726614523238837, -0.9093749993854999270 ) ) ;
#2755=CARTESIAN_POINT ( 'NONE',  ( 19.68408634441910721, -5.407089921784855591, -9.440624999385555327 ) ) ;
#2764=ORIENTED_EDGE ( 'NONE', *, *, #13312, .F. ) ;
#2768=CARTESIAN_POINT ( 'NONE',  ( 13.44051670066911619, -5.407089921784859143, -5.465624999385548577 ) ) ;
#2780=ADVANCED_FACE ( 'NONE', ( #20488 ), #35241, .F. ) ;
#2800=CARTESIAN_POINT ( 'NONE',  ( 16.56230152254411436, 7.209453229046482114, -8.859374999385529748 ) ) ;
#2828=CARTESIAN_POINT ( 'NONE',  ( 16.56230152254411081, -7.209453229046475009, -3.628124999385553107 ) ) ;
#2834=CARTESIAN_POINT ( 'NONE',  ( 16.56230152254411081, -6.928203230275506996, -4.724999998771005849 ) ) ;
#2856=ORIENTED_EDGE ( 'NONE', *, *, #33700, .F. ) ;
#2860=CARTESIAN_POINT ( 'NONE',  ( 19.68408634441911786, -5.407089921784861808, -9.496874999385534366 ) ) ;
#2865=CARTESIAN_POINT ( 'NONE',  ( 22.80587116629411781, 3.604726614523243278, -3.084374999385516514 ) ) ;
#2868=EDGE_CURVE ( 'NONE', #19993, #12997, #5359, .T. ) ;
#2876=FACE_OUTER_BOUND ( 'NONE', #16775, .T. ) ;
#2883=CARTESIAN_POINT ( 'NONE',  ( 22.56230152254412147, 3.464101615137759271, -5.137500000000033928 ) ) ;
#2892=CARTESIAN_POINT ( 'NONE',  ( 16.56230152254410726, 0.000000000000000000, -10.00000000000000000 ) ) ;
#2904=CARTESIAN_POINT ( 'NONE',  ( 10.31873187879410914, 0.000000000000000000, -1.996874999385528371 ) ) ;
#2910=ORIENTED_EDGE ( 'NONE', *, *, #10356, .F. ) ;
#2940=CARTESIAN_POINT ( 'NONE',  ( 16.56230152254410726, -7.209453229046475009, -8.578124999385506655 ) ) ;
#2949=ORIENTED_EDGE ( 'NONE', *, *, #16877, .F. ) ;
#2953=CARTESIAN_POINT ( 'NONE',  ( 19.68408634441910721, -5.407089921784855591, -4.940624999385550886 ) ) ;
#2955=( BOUNDED_CURVE ( )  B_SPLINE_CURVE ( 2, ( #21166, #28596, #15279, #32514, #20981, #11545, #25761 ),
 .UNSPECIFIED., .F., .F. ) 
 B_SPLINE_CURVE_WITH_KNOTS ( ( 3, 2, 2, 3 ),
 ( 0.1521739130434802134, 0.1594202898550745040, 0.1666666666666688501, 0.1739130434782631685 ),
 .UNSPECIFIED. ) 
 CURVE ( )  GEOMETRIC_REPRESENTATION_ITEM ( )  RATIONAL_B_SPLINE_CURVE ( ( 0.9999999999999640288, 0.8660254037844746788, 1.000000000000000000, 0.8660254037844387076, 1.000000000000000000, 0.8660254037843960750, 1.000000000000042633 ) ) 
 REPRESENTATION_ITEM ( '' )  );
#2959=EDGE_LOOP ( 'NONE', ( #12802, #33780 ) ) ;
#2980=VERTEX_POINT ( 'NONE', #6817 ) ;
#2987=CARTESIAN_POINT ( 'NONE',  ( 16.56230152254411436, -7.209453229046482114, -9.534374999385541116 ) ) ;
#3017=CARTESIAN_POINT ( 'NONE',  ( 13.44051670066911441, -5.407089921784859143, -1.865624999385528948 ) ) ;
#3023=CARTESIAN_POINT ( 'NONE',  ( 19.56230152254411436, -5.196152422706629359, -4.687499998771022192 ) ) ;
#3035=ORIENTED_EDGE ( 'NONE', *, *, #24256, .T. ) ;
#3036=CARTESIAN_POINT ( 'NONE',  ( 22.56230152254278210, -3.464101615138517332, -4.649999998770996790 ) ) ;
#3044=ADVANCED_FACE ( 'NONE', ( #18589 ), #33162, .F. ) ;
#3049=VECTOR ( 'NONE', #10113, 1000.000000000000000 ) ;
#3051=CARTESIAN_POINT ( 'NONE',  ( 22.80587116629411781, -3.604726614523238837, -8.559374999385489957 ) ) ;
#3055=CARTESIAN_POINT ( 'NONE',  ( 22.80587116629412492, -3.604726614523238837, -3.159374999385510474 ) ) ;
#3073=CARTESIAN_POINT ( 'NONE',  ( 13.56230152254411969, -5.196152422706638241, -3.525000000000083844 ) ) ;
#3092=CARTESIAN_POINT ( 'NONE',  ( 19.68408634441911431, -5.407089921784861808, -0.9468749993855329894 ) ) ;
#3127=CARTESIAN_POINT ( 'NONE',  ( 16.56230152254411081, -7.209453229046475009, -8.128124999385510918 ) ) ;
#3128=CARTESIAN_POINT ( 'NONE',  ( 13.56230152254410726, 5.196152422706636465, -8.625000000000021316 ) ) ;
#3141=CARTESIAN_POINT ( 'NONE',  ( 19.68408634441910721, -5.407089921784855591, -4.490624999385572913 ) ) ;
#3157=DIRECTION ( 'NONE',  ( 0.000000000000000000, 0.000000000000000000, 1.000000000000000000 ) ) ;
#3171=CARTESIAN_POINT ( 'NONE',  ( 22.80587116629412847, 3.604726614523243278, -9.834374999385516958 ) ) ;
#3177=DIRECTION ( 'NONE',  ( 1.000000000000000000, 0.000000000000000000, 0.000000000000000000 ) ) ;
#3202=CARTESIAN_POINT ( 'NONE',  ( 19.68408634441910365, -5.407089921784855591, -5.390624999385557281 ) ) ;
#3203=EDGE_CURVE ( 'NONE', #9264, #35280, #34242, .T. ) ;
#3210=CARTESIAN_POINT ( 'NONE',  ( 19.56230152254410370, 5.196152422706631135, -4.087499998771032317 ) ) ;
#3217=DIRECTION ( 'NONE',  ( 1.000000000000000000, 0.000000000000000000, 0.000000000000000000 ) ) ;
#3219=DIRECTION ( 'NONE',  ( 1.000000000000000000, 0.000000000000000000, 0.000000000000000000 ) ) ;
#3223=ORIENTED_EDGE ( 'NONE', *, *, #14047, .F. ) ;
#3224=CARTESIAN_POINT ( 'NONE',  ( 16.56230152254411081, -6.928203230275506996, -4.724999998771005849 ) ) ;
#3238=CARTESIAN_POINT ( 'NONE',  ( 10.31873187879410558, 0.000000000000000000, -9.196874999385512339 ) ) ;
#3244=CARTESIAN_POINT ( 'NONE',  ( 13.44051670066911086, 5.407089921784862696, -3.871874999385516158 ) ) ;
#3263=CARTESIAN_POINT ( 'NONE',  ( 13.56230152254410548, 5.196152422706636465, -5.025000000000029665 ) ) ;
#3271=DIRECTION ( 'NONE',  ( 0.000000000000000000, 0.000000000000000000, 1.000000000000000000 ) ) ;
#3275=ORIENTED_EDGE ( 'NONE', *, *, #16803, .F. ) ;
#3279=CARTESIAN_POINT ( 'NONE',  ( 13.44051670066911086, -5.407089921784865361, -0.5718749993855187785 ) ) ;
#3286=ORIENTED_EDGE ( 'NONE', *, *, #8631, .F. ) ;
#3312=CARTESIAN_POINT ( 'NONE',  ( 22.80587116629410360, 7.646167579472015790E-16, -8.015624999385517313 ) ) ;
#3319=CARTESIAN_POINT ( 'NONE',  ( 16.56230152254410726, 0.000000000000000000, 2.535898384862258492 ) ) ;
#3326=CARTESIAN_POINT ( 'NONE',  ( 13.44051670066911619, -5.407089921784859143, -4.565624999385536675 ) ) ;
#3339=CARTESIAN_POINT ( 'NONE',  ( 16.56230152254410726, 0.000000000000000000, -10.00000000000000000 ) ) ;
#3341=CARTESIAN_POINT ( 'NONE',  ( 22.56230152254411792, 7.347880794884125653E-16, -0.2250000000000584865 ) ) ;
#3362=CARTESIAN_POINT ( 'NONE',  ( 22.80587116629410716, 7.646167579472015790E-16, -1.265624999385539518 ) ) ;
#3364=PLANE ( 'NONE',  #6170 ) ;
#3373=ADVANCED_FACE ( 'NONE', ( #22355 ), #1874, .F. ) ;
#3394=CARTESIAN_POINT ( 'NONE',  ( 19.68408634441910721, 5.407089921784857367, -6.590624999385563676 ) ) ;
#3399=CARTESIAN_POINT ( 'NONE',  ( 16.56230152254410726, 6.928203230275506996, -6.749999998770969789 ) ) ;
#3412=EDGE_LOOP ( 'NONE', ( #13119, #17010, #21267, #27489 ) ) ;
#3420=CARTESIAN_POINT ( 'NONE',  ( 19.68408634441910721, 5.407089921784857367, -0.2906249993855358760 ) ) ;
#3428=CARTESIAN_POINT ( 'NONE',  ( 19.56230152254412502, -5.196152422706635576, -1.200000000000062128 ) ) ;
#3430=CARTESIAN_POINT ( 'NONE',  ( 16.56230152254411436, -7.209453229046482114, -4.134374999385496352 ) ) ;
#3441=ORIENTED_EDGE ( 'NONE', *, *, #11948, .T. ) ;
#3448=CARTESIAN_POINT ( 'NONE',  ( 22.56230152254411436, 3.464101615137759271, -6.037500000000025402 ) ) ;
#3470=CARTESIAN_POINT ( 'NONE',  ( 19.68408634441912142, -5.407089921784861808, -1.396874999385538940 ) ) ;
#3498=VECTOR ( 'NONE', #5141, 1000.000000000000000 ) ;
#3501=CARTESIAN_POINT ( 'NONE',  ( 22.80587116629411071, -3.604726614523235284, -9.403124999385536142 ) ) ;
#3515=CARTESIAN_POINT ( 'NONE',  ( 22.80587116629411071, -3.604726614523235284, -5.353124999385542537 ) ) ;
#3521=ORIENTED_EDGE ( 'NONE', *, *, #18712, .T. ) ;
#3531=CARTESIAN_POINT ( 'NONE',  ( 16.56230152254410726, 0.000000000000000000, -10.00000000000000000 ) ) ;
#3555=CARTESIAN_POINT ( 'NONE',  ( 10.31873187879411091, 3.604726614523236616, -0.6281249993855065883 ) ) ;
#3567=UNCERTAINTY_MEASURE_WITH_UNIT (LENGTH_MEASURE( 1.000000000000000082E-05 ), #34263, 'distance_accuracy_value', 'NONE');
#3584=CARTESIAN_POINT ( 'NONE',  ( 16.56230152254411081, 7.209453229046475009, -6.103124999385545202 ) ) ;
#3591=CARTESIAN_POINT ( 'NONE',  ( 16.56230152254411081, 6.928203230275506996, -5.849999998771011178 ) ) ;
#3596=CARTESIAN_POINT ( 'NONE',  ( 22.80587116629412847, 3.604726614523243278, -4.884374999385531879 ) ) ;
#3616=ORIENTED_EDGE ( 'NONE', *, *, #4742, .F. ) ;
#3622=VERTEX_POINT ( 'NONE', #2615 ) ;
#3623=CARTESIAN_POINT ( 'NONE',  ( 13.44051670066910908, 5.407089921784862696, -4.321874999385522109 ) ) ;
#3634=ORIENTED_EDGE ( 'NONE', *, *, #27555, .T. ) ;
#3641=CARTESIAN_POINT ( 'NONE',  ( 10.56230152254410726, 0.000000000000000000, -5.850000000000049383 ) ) ;
#3642=ORIENTED_EDGE ( 'NONE', *, *, #9417, .T. ) ;
#3649=DIRECTION ( 'NONE',  ( 0.000000000000000000, 0.000000000000000000, 1.000000000000000000 ) ) ;
#3650=CARTESIAN_POINT ( 'NONE',  ( 16.56230152254411436, 6.928203230275506996, -1.349999998771021614 ) ) ;
#3654=ORIENTED_EDGE ( 'NONE', *, *, #12852, .T. ) ;
#3657=CARTESIAN_POINT ( 'NONE',  ( 16.56230152254411436, -7.209453229046482114, -4.134374999385496352 ) ) ;
#3669=EDGE_CURVE ( 'NONE', #3622, #7868, #13664, .T. ) ;
#3671=CARTESIAN_POINT ( 'NONE',  ( 10.31873187879411091, 3.604726614523236616, -0.6281249993855065883 ) ) ;
#3675=ADVANCED_FACE ( 'NONE', ( #17226, #34277 ), #3364, .T. ) ;
#3680=CARTESIAN_POINT ( 'NONE',  ( 22.56230152254322263, 3.464101615138280632, -0.6375000000000334843 ) ) ;
#3686=CYLINDRICAL_SURFACE ( 'NONE', #28947, 5.999999999999998224 ) ;
#3690=CARTESIAN_POINT ( 'NONE',  ( 16.56230152254410726, 0.000000000000000000, -10.00000000000000000 ) ) ;
#3702=CARTESIAN_POINT ( 'NONE',  ( 16.56230152254411081, 7.209453229046475009, -7.453124999385500438 ) ) ;
#3709=CARTESIAN_POINT ( 'NONE',  ( 22.56230152254411792, 7.347880794884125653E-16, -2.025000000000027001 ) ) ;
#3728=( BOUNDED_CURVE ( )  B_SPLINE_CURVE ( 2, ( #23495, #35044, #6244, #25587, #34307, #8351, #5484 ),
 .UNSPECIFIED., .F., .F. ) 
 B_SPLINE_CURVE_WITH_KNOTS ( ( 3, 2, 2, 3 ),
 ( 0.1086956521739144144, 0.1159420289855087466, 0.1231884057971030788, 0.1304347826086973972 ),
 .UNSPECIFIED. ) 
 CURVE ( )  GEOMETRIC_REPRESENTATION_ITEM ( )  RATIONAL_B_SPLINE_CURVE ( ( 0.9999999999999745759, 0.8660254037844641317, 1.000000000000000000, 0.8660254037844387076, 1.000000000000000000, 0.8660254037844064001, 1.000000000000032419 ) ) 
 REPRESENTATION_ITEM ( '' )  );
#3735=CARTESIAN_POINT ( 'NONE',  ( 19.68408634441910721, 5.407089921784857367, -2.090624999385559679 ) ) ;
#3738=DIRECTION ( 'NONE',  ( 0.000000000000000000, 0.000000000000000000, 1.000000000000000000 ) ) ;
#3751=( BOUNDED_CURVE ( )  B_SPLINE_CURVE ( 2, ( #28843, #8764, #5721, #34168, #14636, #17302, #19788 ),
 .UNSPECIFIED., .F., .F. ) 
 B_SPLINE_CURVE_WITH_KNOTS ( ( 3, 2, 2, 3 ),
 ( 0.1304347826086947326, 0.1376811594202889955, 0.1449275362318832860, 0.1521739130434775489 ),
 .UNSPECIFIED. ) 
 CURVE ( )  GEOMETRIC_REPRESENTATION_ITEM ( )  RATIONAL_B_SPLINE_CURVE ( ( 1.000000000000016875, 0.8660254037844218322, 1.000000000000000000, 0.8660254037844387076, 1.000000000000000000, 0.8660254037844520303, 0.9999999999999866773 ) ) 
 REPRESENTATION_ITEM ( '' )  );
#3765=CARTESIAN_POINT ( 'NONE',  ( 10.31873187879410736, 3.604726614523236616, -5.128124999385527794 ) ) ;
#3769=CYLINDRICAL_SURFACE ( 'NONE', #32755, 5.999999999999998224 ) ;
#3771=CARTESIAN_POINT ( 'NONE',  ( 22.56230152254411436, -3.464101615137751278, -5.099999998771006737 ) ) ;
#3776=CARTESIAN_POINT ( 'NONE',  ( 22.80587116629412847, 3.604726614523243278, -3.984374999385507987 ) ) ;
#3802=CARTESIAN_POINT ( 'NONE',  ( 13.56230152254410370, 5.196152422706630247, -8.062499998771011533 ) ) ;
#3803=ORIENTED_EDGE ( 'NONE', *, *, #2165, .T. ) ;
#3804=CARTESIAN_POINT ( 'NONE',  ( 22.80587116629411426, -3.604726614523238837, -6.309374999385513050 ) ) ;
#3824=CARTESIAN_POINT ( 'NONE',  ( 10.56230152254411081, 0.000000000000000000, -0.1687499993855146041 ) ) ;
#3826=CARTESIAN_POINT ( 'NONE',  ( 10.56230152254410726, 3.464101615137757051, -6.787500000000028955 ) ) ;
#3837=LINE ( 'NONE', #27341, #5454 ) ;
#3843=EDGE_CURVE ( 'NONE', #34832, #29417, #1457, .T. ) ;
#3844=CARTESIAN_POINT ( 'NONE',  ( 13.44051670066911619, -5.407089921784865361, -3.721874999385532679 ) ) ;
#3856=CARTESIAN_POINT ( 'NONE',  ( 22.56230152254410370, 0.000000000000000000, -10.00000000000000000 ) ) ;
#3869=DIRECTION ( 'NONE',  ( 0.000000000000000000, 0.000000000000000000, 1.000000000000000000 ) ) ;
#3872=CARTESIAN_POINT ( 'NONE',  ( 10.56230152254411259, -3.464101615137761048, -0.8625000000000265787 ) ) ;
#3886=STYLED_ITEM ( 'NONE', ( #27509 ), #20554 ) ;
#3888=ADVANCED_FACE ( 'NONE', ( #15880 ), #14352, .T. ) ;
#3890=CARTESIAN_POINT ( 'NONE',  ( 22.80587116629410716, 7.646167579472015790E-16, -5.765624999385543958 ) ) ;
#3899=CARTESIAN_POINT ( 'NONE',  ( 13.56230152254411792, -5.196152422706638241, -3.975000000000061817 ) ) ;
#3917=ORIENTED_EDGE ( 'NONE', *, *, #30423, .T. ) ;
#3924=CARTESIAN_POINT ( 'NONE',  ( 13.44051670066911264, 5.407089921784856479, -3.365624999385530280 ) ) ;
#3927=DIRECTION ( 'NONE',  ( -1.000000000000000000, 0.000000000000000000, 0.000000000000000000 ) ) ;
#3955=CARTESIAN_POINT ( 'NONE',  ( 13.44051670066911264, 5.407089921784856479, -5.615624999385532057 ) ) ;
#3962=CARTESIAN_POINT ( 'NONE',  ( 10.56230152254410726, 3.464101615137752166, -5.774999998771017218 ) ) ;
#3965=CARTESIAN_POINT ( 'NONE',  ( 22.80587116629412137, 7.646167579472024665E-16, -4.471874999385533123 ) ) ;
#3978=CARTESIAN_POINT ( 'NONE',  ( 16.56230152254411081, -6.928203230275506996, -5.174999998771001586 ) ) ;
#3994=CARTESIAN_POINT ( 'NONE',  ( 13.44051670066911441, -5.407089921784865361, -6.421874999385540406 ) ) ;
#4002=CARTESIAN_POINT ( 'NONE',  ( 16.56230152254411081, -6.928203230275506996, -9.674999998771022902 ) ) ;
#4016=CARTESIAN_POINT ( 'NONE',  ( 19.56230152254411792, -5.196152422706635576, -6.150000000000044764 ) ) ;
#4033=CARTESIAN_POINT ( 'NONE',  ( 19.68408634441910721, 5.407089921784862696, -4.396874999385541827 ) ) ;
#4054=VECTOR ( 'NONE', #6445, 999.9999999999998863 ) ;
#4059=DIRECTION ( 'NONE',  ( 0.000000000000000000, 0.000000000000000000, 1.000000000000000000 ) ) ;
#4079=CARTESIAN_POINT ( 'NONE',  ( 13.44051670066911264, 5.407089921784856479, -6.065624999385538452 ) ) ;
#4081=CARTESIAN_POINT ( 'NONE',  ( 22.56230152254410370, 7.347880794884117764E-16, -2.362499998771028231 ) ) ;
#4083=ORIENTED_EDGE ( 'NONE', *, *, #20736, .T. ) ;
#4086=ORIENTED_EDGE ( 'NONE', *, *, #8477, .T. ) ;
#4094=CARTESIAN_POINT ( 'NONE',  ( 10.56230152254427601, -3.464101615137852974, -5.812500000000041744 ) ) ;
#4095=ADVANCED_FACE ( 'NONE', ( #18348 ), #27242, .F. ) ;
#4116=CARTESIAN_POINT ( 'NONE',  ( 22.80587116629411781, -3.604726614523235284, -3.553124999385526728 ) ) ;
#4120=DIRECTION ( 'NONE',  ( 1.000000000000000000, 0.000000000000000000, 0.000000000000000000 ) ) ;
#4123=CARTESIAN_POINT ( 'NONE',  ( 22.56230152254469346, -3.464101615137414214, -7.799999998771006027 ) ) ;
#4148=CARTESIAN_POINT ( 'NONE',  ( 16.56230152254411081, -7.209453229046475009, -8.128124999385510918 ) ) ;
#4154=CARTESIAN_POINT ( 'NONE',  ( 13.56230152254410370, 5.196152422706630247, -4.912499998770996967 ) ) ;
#4155=EDGE_CURVE ( 'NONE', #28841, #4918, #31359, .T. ) ;
#4158=CARTESIAN_POINT ( 'NONE',  ( 13.44051670066911086, 5.407089921784862696, -3.871874999385516158 ) ) ;
#4186=CARTESIAN_POINT ( 'NONE',  ( 10.31873187879410558, 0.000000000000000000, -6.946874999385510563 ) ) ;
#4187=ORIENTED_EDGE ( 'NONE', *, *, #34152, .F. ) ;
#4204=CARTESIAN_POINT ( 'NONE',  ( 22.56230152254412147, -3.464101615137755275, -7.912500000000034284 ) ) ;
#4213=CARTESIAN_POINT ( 'NONE',  ( 19.56230152254410370, 5.196152422706631135, -1.387499998770996834 ) ) ;
#4219=CARTESIAN_POINT ( 'NONE',  ( 10.31873187879410914, 0.000000000000000000, -4.696874999385508787 ) ) ;
#4232=LINE ( 'NONE', #9554, #3049 ) ;
#4244=CARTESIAN_POINT ( 'NONE',  ( 10.56230152254411614, -3.464101615137761048, -0.4125000000000307865 ) ) ;
#4246=B_SPLINE_CURVE_WITH_KNOTS ( 'NONE', 1,
 ( #28767, #23658 ),
 .UNSPECIFIED., .F., .F.,
 ( 2, 2 ),
 ( 0.000000000000000000, 1.000000000000000000 ),
 .UNSPECIFIED. ) ;
#4250=CARTESIAN_POINT ( 'NONE',  ( 22.56230152254400423, -3.464101615137808565, -0.5999999987710193938 ) ) ;
#4262=CARTESIAN_POINT ( 'NONE',  ( 10.31873187879410914, 0.000000000000000000, -7.790624999385542537 ) ) ;
#4264=CARTESIAN_POINT ( 'NONE',  ( 22.56230152254410370, 0.000000000000000000, -10.00000000000000000 ) ) ;
#4267=ORIENTED_EDGE ( 'NONE', *, *, #20101, .F. ) ;
#4271=LINE ( 'NONE', #21353, #32148 ) ;
#4299=CARTESIAN_POINT ( 'NONE',  ( 13.44051670066911264, -5.407089921784859143, -3.215624999385519267 ) ) ;
#4301=DIRECTION ( 'NONE',  ( 1.000000000000000000, 0.000000000000000000, 0.000000000000000000 ) ) ;
#4308=EDGE_LOOP ( 'NONE', ( #16637, #26921, #22360, #2910 ) ) ;
#4330=CARTESIAN_POINT ( 'NONE',  ( 19.68408634441910721, 5.407089921784857367, -8.840624999385537919 ) ) ;
#4336=CARTESIAN_POINT ( 'NONE',  ( 13.56230152254410370, 5.196152422706630247, -8.062499998771011533 ) ) ;
#4339=CARTESIAN_POINT ( 'NONE',  ( 10.31873187879410914, 0.000000000000000000, -4.696874999385508787 ) ) ;
#4354=DIRECTION ( 'NONE',  ( 0.000000000000000000, 0.000000000000000000, 1.000000000000000000 ) ) ;
#4356=CARTESIAN_POINT ( 'NONE',  ( 10.31873187879410558, 3.604726614523236616, -2.878124999385517135 ) ) ;
#4360=ORIENTED_EDGE ( 'NONE', *, *, #36569, .F. ) ;
#4361=AXIS2_PLACEMENT_3D ( 'NONE', #4901, #13445, #30878 ) ;
#4370=CARTESIAN_POINT ( 'NONE',  ( 19.68408634441912142, -5.407089921784861808, -6.796874999385527083 ) ) ;
#4378=SURFACE_STYLE_USAGE ( .BOTH. , #30164 ) ;
#4382=CARTESIAN_POINT ( 'NONE',  ( 10.56230152254411614, -3.464101615137757051, -1.649999998770997678 ) ) ;
#4389=CARTESIAN_POINT ( 'NONE',  ( 10.31873187879410914, 0.000000000000000000, -0.5906249993855583469 ) ) ;
#4390=ORIENTED_EDGE ( 'NONE', *, *, #21678, .T. ) ;
#4391=CARTESIAN_POINT ( 'NONE',  ( 19.56230152254412502, -5.196152422706635576, -7.950000000000068567 ) ) ;
#4396=( BOUNDED_CURVE ( )  B_SPLINE_CURVE ( 2, ( #21436, #23706, #15363, #754, #21062, #15174, #12130 ),
 .UNSPECIFIED., .F., .F. ) 
 B_SPLINE_CURVE_WITH_KNOTS ( ( 3, 2, 2, 3 ),
 ( 0.4565217391304328132, 0.4637681159420271593, 0.4710144927536215054, 0.4782608695652158515 ),
 .UNSPECIFIED. ) 
 CURVE ( )  GEOMETRIC_REPRESENTATION_ITEM ( )  RATIONAL_B_SPLINE_CURVE ( ( 1.000000000000035749, 0.8660254037844027364, 1.000000000000000000, 0.8660254037844387076, 1.000000000000000000, 0.8660254037844674624, 0.9999999999999712452 ) ) 
 REPRESENTATION_ITEM ( '' )  );
#4405=CARTESIAN_POINT ( 'NONE',  ( 22.80587116629412137, 7.646167579472024665E-16, -3.121874999385543248 ) ) ;
#4409=EDGE_CURVE ( 'NONE', #31449, #11542, #36437, .T. ) ;
#4446=DIRECTION ( 'NONE',  ( 0.000000000000000000, 0.000000000000000000, 1.000000000000000000 ) ) ;
#4448=CARTESIAN_POINT ( 'NONE',  ( 22.80587116629410360, 7.646167579472015790E-16, -7.565624999385539340 ) ) ;
#4455=VERTEX_POINT ( 'NONE', #37430 ) ;
#4489=CARTESIAN_POINT ( 'NONE',  ( 13.44051670066911619, -5.407089921784859143, -4.565624999385536675 ) ) ;
#4493=CARTESIAN_POINT ( 'NONE',  ( 22.80587116629411781, -3.604726614523238837, -9.459374999385545379 ) ) ;
#4498=CARTESIAN_POINT ( 'NONE',  ( 22.80587116629411781, 3.604726614523243278, -0.8343749993855380520 ) ) ;
#4505=CARTESIAN_POINT ( 'NONE',  ( 16.56230152254410726, 0.000000000000000000, 2.535898384862258492 ) ) ;
#4521=CARTESIAN_POINT ( 'NONE',  ( 13.44051670066911264, 5.407089921784856479, -8.765624999385545735 ) ) ;
#4526=CARTESIAN_POINT ( 'NONE',  ( 10.56230152254411436, -3.464101615137757051, -8.399999998770997678 ) ) ;
#4530=CARTESIAN_POINT ( 'NONE',  ( 10.31873187879410736, 3.604726614523240613, -6.084374999385531169 ) ) ;
#4536=CARTESIAN_POINT ( 'NONE',  ( 13.56230152254410548, 5.196152422706636465, -4.575000000000050804 ) ) ;
#4558=CARTESIAN_POINT ( 'NONE',  ( 22.80587116629411781, 3.604726614523243278, -5.784374999385524241 ) ) ;
#4562=CARTESIAN_POINT ( 'NONE',  ( 22.80587116629410716, -3.604726614523235284, -0.8531249993855525293 ) ) ;
#4570=CARTESIAN_POINT ( 'NONE',  ( 13.56230152254410548, 5.196152422706630247, -1.762499998771011045 ) ) ;
#4574=CARTESIAN_POINT ( 'NONE',  ( 10.56230152254410903, 0.000000000000000000, -1.237499998771041110 ) ) ;
#4580=CARTESIAN_POINT ( 'NONE',  ( 19.56230152254412502, -5.196152422706635576, -8.850000000000052935 ) ) ;
#4590=CARTESIAN_POINT ( 'NONE',  ( 16.56230152254411081, 6.928203230275514990, -3.712500000000020339 ) ) ;
#4595=CARTESIAN_POINT ( 'NONE',  ( 16.56230152254411436, -7.209453229046482114, -6.384374999385507010 ) ) ;
#4604=CARTESIAN_POINT ( 'NONE',  ( 16.56230152254410726, 0.000000000000000000, -10.00000000000000000 ) ) ;
#4615=EDGE_CURVE ( 'NONE', #20931, #12997, #25698, .T. ) ;
#4618=CARTESIAN_POINT ( 'NONE',  ( 22.56230152254412857, -3.464101615137755275, -2.512500000000021494 ) ) ;
#4631=AXIS2_PLACEMENT_3D ( 'NONE', #8852, #2599, #6000 ) ;
#4634=CARTESIAN_POINT ( 'NONE',  ( 22.80587116629411426, -3.604726614523235284, -8.053124999385516958 ) ) ;
#4651=DIRECTION ( 'NONE',  ( 0.000000000000000000, 0.000000000000000000, 1.000000000000000000 ) ) ;
#4660=AXIS2_PLACEMENT_3D ( 'NONE', #10118, #16561, #4796 ) ;
#4669=CARTESIAN_POINT ( 'NONE',  ( 22.80587116629411071, -3.604726614523235284, -4.903124999385513938 ) ) ;
#4673=CARTESIAN_POINT ( 'NONE',  ( 13.44051670066911441, -5.407089921784865361, -9.571874999385554972 ) ) ;
#4679=CARTESIAN_POINT ( 'NONE',  ( 19.68408634441911076, 5.407089921784862696, -1.696874999385505900 ) ) ;
#4690=ORIENTED_EDGE ( 'NONE', *, *, #23960, .T. ) ;
#4699=ADVANCED_FACE ( 'NONE', ( #2388 ), #34416, .F. ) ;
#4703=CARTESIAN_POINT ( 'NONE',  ( 10.31873187879411091, 3.604726614523236616, -8.278124999385530813 ) ) ;
#4708=CARTESIAN_POINT ( 'NONE',  ( 10.56230152254411436, -3.464101615137757051, -8.849999998770995191 ) ) ;
#4712=CARTESIAN_POINT ( 'NONE',  ( 16.56230152254411436, 7.209453229046482114, -5.259374999385500793 ) ) ;
#4741=CARTESIAN_POINT ( 'NONE',  ( 13.34266913871822346, -5.365490278403956204, -9.999999999999996447 ) ) ;
#4742=EDGE_CURVE ( 'NONE', #18566, #29619, #20741, .T. ) ;
#4746=CARTESIAN_POINT ( 'NONE',  ( 10.31873187879410736, 3.604726614523240613, -7.434374999385486404 ) ) ;
#4747=ORIENTED_EDGE ( 'NONE', *, *, #26822, .F. ) ;
#4755=CARTESIAN_POINT ( 'NONE',  ( 10.56230152254411081, 0.000000000000000000, -7.537499998771012955 ) ) ;
#4757=CARTESIAN_POINT ( 'NONE',  ( 19.56230152254411792, -5.196152422706629359, -2.437499998771047949 ) ) ;
#4764=CARTESIAN_POINT ( 'NONE',  ( 16.56230152254411081, -6.928203230275514990, -8.887500000000020606 ) ) ;
#4769=CARTESIAN_POINT ( 'NONE',  ( 16.56230152254410726, 0.000000000000000000, -10.00000000000000000 ) ) ;
#4781=CARTESIAN_POINT ( 'NONE',  ( 10.31873187879411091, -3.604726614523244610, -7.359374999385524418 ) ) ;
#4787=CARTESIAN_POINT ( 'NONE',  ( 16.56230152254411792, 7.209453229046482114, -2.109374999385531080 ) ) ;
#4796=DIRECTION ( 'NONE',  ( 1.000000000000000000, 0.000000000000000000, 0.000000000000000000 ) ) ;
#4803=CARTESIAN_POINT ( 'NONE',  ( 16.56230152254411436, 6.928203230275514990, -1.912500000000037836 ) ) ;
#4819=CARTESIAN_POINT ( 'NONE',  ( 22.80587116629410716, 7.646167579472015790E-16, -9.815624999385569538 ) ) ;
#4858=CARTESIAN_POINT ( 'NONE',  ( 16.56230152254411081, -7.209453229046475009, -5.428124999385503635 ) ) ;
#4867=CARTESIAN_POINT ( 'NONE',  ( 22.80587116629412492, -3.604726614523238837, -0.4593749993855362757 ) ) ;
#4872=AXIS2_PLACEMENT_3D ( 'NONE', #3531, #26647, #12247 ) ;
#4889=CARTESIAN_POINT ( 'NONE',  ( 10.31873187879411091, -3.604726614523240613, -7.753124999385540228 ) ) ;
#4894=CARTESIAN_POINT ( 'NONE',  ( 16.56230152254411081, 6.928203230275506996, -9.449999998771041021 ) ) ;
#4898=CARTESIAN_POINT ( 'NONE',  ( 22.80587116629411781, -3.604726614523238837, -6.759374999385539873 ) ) ;
#4901=CARTESIAN_POINT ( 'NONE',  ( 16.56230152254410726, 0.000000000000000000, 10.00000000000000000 ) ) ;
#4918=VERTEX_POINT ( 'NONE', #23984 ) ;
#4925=CARTESIAN_POINT ( 'NONE',  ( 10.31873187879410736, 3.604726614523240613, -9.234374999385533300 ) ) ;
#4929=LINE ( 'NONE', #3856, #26261 ) ;
#4935=CARTESIAN_POINT ( 'NONE',  ( 22.56230152254410370, 7.347880794884117764E-16, -1.462499998771016330 ) ) ;
#4939=( BOUNDED_CURVE ( )  B_SPLINE_CURVE ( 2, ( #7204, #19337, #7755, #18777, #7384, #35993, #13442 ),
 .UNSPECIFIED., .F., .F. ) 
 B_SPLINE_CURVE_WITH_KNOTS ( ( 3, 2, 2, 3 ),
 ( 0.1521739130434775489, 0.1594202898550718672, 0.1666666666666661856, 0.1739130434782605317 ),
 .UNSPECIFIED. ) 
 CURVE ( )  GEOMETRIC_REPRESENTATION_ITEM ( )  RATIONAL_B_SPLINE_CURVE ( ( 1.000000000000013545, 0.8660254037844254960, 1.000000000000000000, 0.8660254037844387076, 1.000000000000000000, 0.8660254037844448138, 0.9999999999999938938 ) ) 
 REPRESENTATION_ITEM ( '' )  );
#4943=CARTESIAN_POINT ( 'NONE',  ( 10.56230152254410903, 3.464101615137757051, -9.487500000000068212 ) ) ;
#4952=CARTESIAN_POINT ( 'NONE',  ( 22.56230152254410370, 0.000000000000000000, -10.00000000000000000 ) ) ;
#4961=CARTESIAN_POINT ( 'NONE',  ( 22.80587116629411426, -3.604726614523238837, -6.309374999385513050 ) ) ;
#4967=ORIENTED_EDGE ( 'NONE', *, *, #15688, .F. ) ;
#4968=CARTESIAN_POINT ( 'NONE',  ( 19.68408634441911076, 5.407089921784862696, -1.696874999385505900 ) ) ;
#4974=CARTESIAN_POINT ( 'NONE',  ( 19.56230152254411792, 5.196152422706637353, -9.600000000000052935 ) ) ;
#4985=CARTESIAN_POINT ( 'NONE',  ( 22.56230152254412502, 7.347880794884125653E-16, -2.925000000000066436 ) ) ;
#5000=ORIENTED_EDGE ( 'NONE', *, *, #14751, .F. ) ;
#5006=CARTESIAN_POINT ( 'NONE',  ( 13.44051670066911441, -5.407089921784859143, -8.615624999385563143 ) ) ;
#5017=CARTESIAN_POINT ( 'NONE',  ( 22.56230152254534360, -3.464101615137050505, -4.312500000000021316 ) ) ;
#5025=CARTESIAN_POINT ( 'NONE',  ( 10.56230152254410903, 7.347880794884117764E-16, -10.00000000000000000 ) ) ;
#5035=ORIENTED_EDGE ( 'NONE', *, *, #3203, .T. ) ;
#5044=CARTESIAN_POINT ( 'NONE',  ( 16.56230152254411081, -7.209453229046475009, -7.678124999385515181 ) ) ;
#5052=CARTESIAN_POINT ( 'NONE',  ( 19.68408634441911431, -5.407089921784861808, -0.9468749993855329894 ) ) ;
#5059=CARTESIAN_POINT ( 'NONE',  ( 19.68408634441911076, -5.407089921784855591, -1.340624999385559013 ) ) ;
#5065=ORIENTED_EDGE ( 'NONE', *, *, #32048, .T. ) ;
#5082=ADVANCED_FACE ( 'NONE', ( #25279 ), #33436, .F. ) ;
#5084=CARTESIAN_POINT ( 'NONE',  ( 22.56230152254411436, -3.464101615137751278, -7.349999998771018284 ) ) ;
#5087=CARTESIAN_POINT ( 'NONE',  ( 22.80587116629412847, 3.604726614523243278, -9.834374999385516958 ) ) ;
#5088=CARTESIAN_POINT ( 'NONE',  ( 22.80587116629411426, 3.604726614523243278, -7.584374999385505411 ) ) ;
#5094=DIRECTION ( 'NONE',  ( 0.000000000000000000, 0.000000000000000000, 1.000000000000000000 ) ) ;
#5108=ORIENTED_EDGE ( 'NONE', *, *, #20736, .F. ) ;
#5116=CARTESIAN_POINT ( 'NONE',  ( 13.44051670066910731, 5.407089921784862696, -7.471874999385508254 ) ) ;
#5119=CARTESIAN_POINT ( 'NONE',  ( 10.31873187879411091, -3.604726614523240613, -3.253124999385519356 ) ) ;
#5122=CARTESIAN_POINT ( 'NONE',  ( 22.56230152254368804, -3.464101615137996415, -7.349999998771023613 ) ) ;
#5125=CARTESIAN_POINT ( 'NONE',  ( 19.56230152254410370, 5.196152422706631135, -1.387499998770996834 ) ) ;
#5132=CARTESIAN_POINT ( 'NONE',  ( 15.52041721667876573, 5.908847357411728396, -9.999476446176704059 ) ) ;
#5135=CARTESIAN_POINT ( 'NONE',  ( 16.56230152254411792, -6.928203230275514990, -3.487500000000039346 ) ) ;
#5141=DIRECTION ( 'NONE',  ( 0.000000000000000000, 0.000000000000000000, 1.000000000000000000 ) ) ;
#5148=CARTESIAN_POINT ( 'NONE',  ( 10.31873187879410736, 0.000000000000000000, -5.146874999385541827 ) ) ;
#5151=ORIENTED_EDGE ( 'NONE', *, *, #21319, .T. ) ;
#5152=CARTESIAN_POINT ( 'NONE',  ( 13.44051670066911264, 5.407089921784862696, -2.521874999385525840 ) ) ;
#5173=CARTESIAN_POINT ( 'NONE',  ( 22.56230152254411792, 7.347880794884125653E-16, -1.575000000000048583 ) ) ;
#5181=DIRECTION ( 'NONE',  ( 1.000000000000000000, 0.000000000000000000, 0.000000000000000000 ) ) ;
#5189=ORIENTED_EDGE ( 'NONE', *, *, #35777, .T. ) ;
#5194=CARTESIAN_POINT ( 'NONE',  ( 22.80587116629411071, -3.604726614523235284, -9.853124999385531879 ) ) ;
#5204=CARTESIAN_POINT ( 'NONE',  ( 13.56230152254411614, -5.196152422706638241, -1.275000000000053868 ) ) ;
#5232=CARTESIAN_POINT ( 'NONE',  ( 10.31873187879411269, -3.604726614523240613, -5.503124999385529570 ) ) ;
#5240=CARTESIAN_POINT ( 'NONE',  ( 22.80587116629411781, 3.604726614523243278, -0.3843749993855423153 ) ) ;
#5246=CARTESIAN_POINT ( 'NONE',  ( 19.68408634441910721, 5.407089921784857367, -1.190624999385520022 ) ) ;
#5270=CARTESIAN_POINT ( 'NONE',  ( 19.56230152254411081, -5.196152422706629359, -10.08749999877103853 ) ) ;
#5274=CARTESIAN_POINT ( 'NONE',  ( 22.80587116629411781, 3.604726614523243278, -5.334374999385495641 ) ) ;
#5301=CARTESIAN_POINT ( 'NONE',  ( 10.31873187879410558, 0.000000000000000000, -8.746874999385534366 ) ) ;
#5306=CARTESIAN_POINT ( 'NONE',  ( 13.44051670066911441, 5.407089921784856479, -2.465624999385545912 ) ) ;
#5307=EDGE_CURVE ( 'NONE', #18752, #33087, #9111, .T. ) ;
#5312=CARTESIAN_POINT ( 'NONE',  ( 16.56230152254411081, 6.928203230275506996, -3.149999998770972365 ) ) ;
#5316=AXIS2_PLACEMENT_3D ( 'NONE', #7585, #4354, #7957 ) ;
#5319=CARTESIAN_POINT ( 'NONE',  ( 10.56230152254410903, 0.000000000000000000, -1.687499998771019305 ) ) ;
#5321=CARTESIAN_POINT ( 'NONE',  ( 10.31873187879410558, 3.604726614523236616, -2.878124999385517135 ) ) ;
#5337=CARTESIAN_POINT ( 'NONE',  ( 16.56230152254411436, -7.209453229046482114, -7.284374999385498484 ) ) ;
#5342=CARTESIAN_POINT ( 'NONE',  ( 22.80587116629411781, -3.604726614523238837, -0.9093749993854999270 ) ) ;
#5358=CARTESIAN_POINT ( 'NONE',  ( 10.56230152254410193, 3.464101615137757051, -3.187499999999998668 ) ) ;
#5359=LINE ( 'NONE', #20866, #4054 ) ;
#5375=CARTESIAN_POINT ( 'NONE',  ( 16.56230152254411436, 7.209453229046482114, -0.3093749993854842950 ) ) ;
#5403=CYLINDRICAL_SURFACE ( 'NONE', #33800, 5.999999999999998224 ) ;
#5407=CARTESIAN_POINT ( 'NONE',  ( 10.31873187879411091, 0.000000000000000000, -7.340624999385508609 ) ) ;
#5416=CARTESIAN_POINT ( 'NONE',  ( 13.44051670066911264, 5.407089921784862696, -2.521874999385525840 ) ) ;
#5422=CARTESIAN_POINT ( 'NONE',  ( 16.56230152254411436, 7.209453229046475009, -2.503124999385547778 ) ) ;
#5436=EDGE_CURVE ( 'NONE', #11055, #31857, #18541, .T. ) ;
#5437=DIRECTION ( 'NONE',  ( 0.000000000000000000, 0.000000000000000000, 1.000000000000000000 ) ) ;
#5440=CARTESIAN_POINT ( 'NONE',  ( 10.31873187879411091, -3.604726614523240613, -9.103124999385528326 ) ) ;
#5441=VECTOR ( 'NONE', #18205, 1000.000000000000000 ) ;
#5442=CARTESIAN_POINT ( 'NONE',  ( 10.56230152254410903, 7.347880794884117764E-16, -10.00000000000000000 ) ) ;
#5448=CARTESIAN_POINT ( 'NONE',  ( 22.56230152254410370, 3.464101615137755275, -9.974999998770998744 ) ) ;
#5452=CARTESIAN_POINT ( 'NONE',  ( 10.31873187879411091, -3.604726614523244610, -9.609374999385535077 ) ) ;
#5453=CARTESIAN_POINT ( 'NONE',  ( 19.56230152254412502, 5.196152422706637353, -0.1500000000000112355 ) ) ;
#5454=VECTOR ( 'NONE', #10095, 1000.000000000000000 ) ;
#5459=CARTESIAN_POINT ( 'NONE',  ( 13.56230152254410548, 5.196152422706630247, -3.562499998771007093 ) ) ;
#5482=CARTESIAN_POINT ( 'NONE',  ( 10.31873187879411091, -3.604726614523240613, -4.153124999385542360 ) ) ;
#5484=CARTESIAN_POINT ( 'NONE',  ( 10.56230152254410903, 0.000000000000000000, -1.687499998771019305 ) ) ;
#5487=CARTESIAN_POINT ( 'NONE',  ( 13.56230152254411436, -5.196152422706632912, -3.412499998771051146 ) ) ;
#5498=CARTESIAN_POINT ( 'NONE',  ( 16.56230152254411436, -7.209453229046475009, -0.9281249993855145153 ) ) ;
#5508=CARTESIAN_POINT ( 'NONE',  ( 10.56230152254395627, -3.464101615137665124, -8.849999998770995191 ) ) ;
#5515=CARTESIAN_POINT ( 'NONE',  ( 22.80587116629411071, 3.604726614523243278, -8.934374999385493510 ) ) ;
#5520=CARTESIAN_POINT ( 'NONE',  ( 13.44051670066911264, 5.407089921784862696, -0.2718749993855240632 ) ) ;
#5535=CIRCLE ( 'NONE', #30965, 5.999999999999998224 ) ;
#5538=CARTESIAN_POINT ( 'NONE',  ( 16.56230152254411436, -6.928203230275514990, -3.937500000000034639 ) ) ;
#5544=CARTESIAN_POINT ( 'NONE',  ( 22.56230152254411792, 7.347880794884125653E-16, -6.525000000000058975 ) ) ;
#5558=CARTESIAN_POINT ( 'NONE',  ( 10.31873187879410736, -3.604726614523244610, -2.409374999385539340 ) ) ;
#5565=ORIENTED_EDGE ( 'NONE', *, *, #31874, .T. ) ;
#5580=CARTESIAN_POINT ( 'NONE',  ( 22.56230152254478583, -3.464101615137372470, -5.212500000000051870 ) ) ;
#5587=CARTESIAN_POINT ( 'NONE',  ( 13.56230152254410370, 5.196152422706630247, -9.862499998771006915 ) ) ;
#5590=CARTESIAN_POINT ( 'NONE',  ( 22.80587116629411071, 3.604726614523238837, -5.728124999385511451 ) ) ;
#5591=DIRECTION ( 'NONE',  ( 0.000000000000000000, 0.000000000000000000, 1.000000000000000000 ) ) ;
#5602=PRODUCT ( 'coupler', 'coupler', '', ( #1943 ) ) ;
#5605=CARTESIAN_POINT ( 'NONE',  ( 22.80587116629411426, -3.604726614523235284, -3.103124999385563410 ) ) ;
#5607=( BOUNDED_CURVE ( )  B_SPLINE_CURVE ( 2, ( #8836, #6550, #15081, #6173, #32321, #26444, #26631 ),
 .UNSPECIFIED., .F., .F. ) 
 B_SPLINE_CURVE_WITH_KNOTS ( ( 3, 2, 2, 3 ),
 ( 0.2826086956521748905, 0.2898550724637692366, 0.2971014492753635827, 0.3043478260869579288 ),
 .UNSPECIFIED. ) 
 CURVE ( )  GEOMETRIC_REPRESENTATION_ITEM ( )  RATIONAL_B_SPLINE_CURVE ( ( 0.9999999999999815703, 0.8660254037844571373, 1.000000000000000000, 0.8660254037844387076, 1.000000000000000000, 0.8660254037844130615, 1.000000000000025535 ) ) 
 REPRESENTATION_ITEM ( '' )  );
#5609=LINE ( 'NONE', #28368, #14857 ) ;
#5639=CARTESIAN_POINT ( 'NONE',  ( 19.68408634441910721, 5.407089921784862696, -8.896874999385516958 ) ) ;
#5642=CARTESIAN_POINT ( 'NONE',  ( 16.56230152254411081, -6.928203230275506996, -1.124999998771007759 ) ) ;
#5643=ADVANCED_FACE ( 'NONE', ( #23748 ), #15596, .F. ) ;
#5650=CARTESIAN_POINT ( 'NONE',  ( 15.06230152254410548, 0.000000000000000000, 0.000000000000000000 ) ) ;
#5656=EDGE_CURVE ( 'NONE', #23999, #27522, #28648, .T. ) ;
#5670=CARTESIAN_POINT ( 'NONE',  ( 19.68408634441910721, -5.407089921784855591, -3.590624999385533478 ) ) ;
#5676=CARTESIAN_POINT ( 'NONE',  ( 10.56230152254411259, 3.464101615137752166, -4.424999998771030008 ) ) ;
#5693=LINE ( 'NONE', #37339, #24704 ) ;
#5695=LINE ( 'NONE', #31121, #17912 ) ;
#5704=CARTESIAN_POINT ( 'NONE',  ( 22.80587116629411426, 7.646167579472024665E-16, -8.071874999385524774 ) ) ;
#5709=CARTESIAN_POINT ( 'NONE',  ( 10.31873187879410736, -3.604726614523244610, -4.659374999385518024 ) ) ;
#5713=CARTESIAN_POINT ( 'NONE',  ( 10.56230152254411081, 0.000000000000000000, -0.3374999987710014526 ) ) ;
#5721=CARTESIAN_POINT ( 'NONE',  ( 13.56230152254410726, 5.196152422706636465, -1.425000000000037348 ) ) ;
#5726=CARTESIAN_POINT ( 'NONE',  ( 22.56230152254412147, 3.464101615137759271, -4.687500000000039080 ) ) ;
#5746=CARTESIAN_POINT ( 'NONE',  ( 16.56230152254411436, -7.209453229046482114, -0.5343749993854981506 ) ) ;
#5753=AXIS2_PLACEMENT_3D ( 'NONE', #20449, #14938, #3177 ) ;
#5783=CARTESIAN_POINT ( 'NONE',  ( 19.68408634441910721, -5.407089921784855591, -9.890624999385533300 ) ) ;
#5796=CARTESIAN_POINT ( 'NONE',  ( 19.68408634441910721, 5.407089921784857367, -3.890624999385555505 ) ) ;
#5799=DIRECTION ( 'NONE',  ( 0.000000000000000000, 0.000000000000000000, 1.000000000000000000 ) ) ;
#5801=ORIENTED_EDGE ( 'NONE', *, *, #19380, .T. ) ;
#5813=DIRECTION ( 'NONE',  ( 0.000000000000000000, 0.000000000000000000, 1.000000000000000000 ) ) ;
#5825=CARTESIAN_POINT ( 'NONE',  ( 22.56230152254310894, -3.464101615138333923, -8.249999998771022192 ) ) ;
#5830=CARTESIAN_POINT ( 'NONE',  ( 19.68408634441911786, -5.407089921784861808, -8.596874999385523353 ) ) ;
#5832=( BOUNDED_CURVE ( )  B_SPLINE_CURVE ( 2, ( #18866, #12786, #35709, #1404, #36269, #33435, #7476 ),
 .UNSPECIFIED., .F., .F. ) 
 B_SPLINE_CURVE_WITH_KNOTS ( ( 3, 2, 2, 3 ),
 ( 0.7826086956521763893, 0.7898550724637706244, 0.7971014492753649705, 0.8043478260869593166 ),
 .UNSPECIFIED. ) 
 CURVE ( )  GEOMETRIC_REPRESENTATION_ITEM ( )  RATIONAL_B_SPLINE_CURVE ( ( 0.9999999999999548139, 0.8660254037844838937, 1.000000000000000000, 0.8660254037844387076, 1.000000000000000000, 0.8660254037843874153, 1.000000000000051292 ) ) 
 REPRESENTATION_ITEM ( '' )  );
#5860=CARTESIAN_POINT ( 'NONE',  ( 13.44051670066911264, 5.407089921784856479, -3.365624999385530280 ) ) ;
#5865=CARTESIAN_POINT ( 'NONE',  ( 10.56230152254410903, 3.464101615137752166, -3.524999998771006560 ) ) ;
#5882=DIRECTION ( 'NONE',  ( 0.000000000000000000, 0.000000000000000000, 1.000000000000000000 ) ) ;
#5894=CARTESIAN_POINT ( 'NONE',  ( 10.31873187879410558, 0.000000000000000000, -8.746874999385534366 ) ) ;
#5898=CARTESIAN_POINT ( 'NONE',  ( 10.31873187879410381, 3.604726614523240613, -4.734374999385511096 ) ) ;
#5909=CYLINDRICAL_SURFACE ( 'NONE', #25789, 5.999999999999998224 ) ;
#5915=CARTESIAN_POINT ( 'NONE',  ( 13.56230152254411792, -5.196152422706638241, -3.975000000000061817 ) ) ;
#5934=CARTESIAN_POINT ( 'NONE',  ( 22.80587116629411426, 7.646167579472024665E-16, -1.771874999385525395 ) ) ;
#5968=CARTESIAN_POINT ( 'NONE',  ( 22.56230152254410370, 0.000000000000000000, -10.00000000000000000 ) ) ;
#5969=CARTESIAN_POINT ( 'NONE',  ( 14.39393478667391690, 5.957546110389989380, -10.12707779971139210 ) ) ;
#5975=CARTESIAN_POINT ( 'NONE',  ( 15.52041717089296213, 5.908847349338256727, -9.999738233010948107 ) ) ;
#5978=EDGE_LOOP ( 'NONE', ( #17658, #1037, #2510, #14766 ) ) ;
#5983=CARTESIAN_POINT ( 'NONE',  ( 10.31873187879411091, -3.604726614523240613, -4.153124999385542360 ) ) ;
#5986=FACE_OUTER_BOUND ( 'NONE', #23300, .T. ) ;
#5991=CARTESIAN_POINT ( 'NONE',  ( 16.56230152254410726, 0.000000000000000000, -10.00000000000000000 ) ) ;
#6000=DIRECTION ( 'NONE',  ( 1.000000000000000000, 0.000000000000000000, 0.000000000000000000 ) ) ;
#6010=CARTESIAN_POINT ( 'NONE',  ( 19.56230152254410370, 5.196152422706631135, -9.937499998770999099 ) ) ;
#6014=CARTESIAN_POINT ( 'NONE',  ( 10.31873187879410736, -3.604726614523244610, -8.259374999385515892 ) ) ;
#6040=VECTOR ( 'NONE', #32491, 1000.000000000000000 ) ;
#6043=CARTESIAN_POINT ( 'NONE',  ( 13.44051670066911264, 5.407089921784856479, -6.065624999385538452 ) ) ;
#6048=CARTESIAN_POINT ( 'NONE',  ( 13.56230152254410548, 5.196152422706630247, -4.012499998771012599 ) ) ;
#6055=CARTESIAN_POINT ( 'NONE',  ( 10.56230152254410903, 7.347880794884117764E-16, -10.00000000000000000 ) ) ;
#6076=CARTESIAN_POINT ( 'NONE',  ( 10.31873187879411091, 3.604726614523240613, -8.784374999385505589 ) ) ;
#6079=CARTESIAN_POINT ( 'NONE',  ( 22.56230152254411792, 7.347880794884125653E-16, -1.125000000000042633 ) ) ;
#6081=CARTESIAN_POINT ( 'NONE',  ( 19.68408634441910721, 5.407089921784862696, -3.046874999385523530 ) ) ;
#6099=CARTESIAN_POINT ( 'NONE',  ( 19.56230152254412147, -5.196152422706635576, -4.800000000000082423 ) ) ;
#6100=ADVANCED_FACE ( 'NONE', ( #27894 ), #1924, .F. ) ;
#6101=ORIENTED_EDGE ( 'NONE', *, *, #79, .T. ) ;
#6121=CARTESIAN_POINT ( 'NONE',  ( 19.68408634441910721, 5.407089921784862696, -2.596874999385518024 ) ) ;
#6126=EDGE_CURVE ( 'NONE', #12454, #24665, #22407, .T. ) ;
#6130=CARTESIAN_POINT ( 'NONE',  ( 13.56230152254410726, 5.196152422706636465, -0.9750000000000591527 ) ) ;
#6158=CARTESIAN_POINT ( 'NONE',  ( 13.44051670066910908, 5.407089921784856479, -7.865624999385534721 ) ) ;
#6159=( BOUNDED_CURVE ( )  B_SPLINE_CURVE ( 2, ( #33491, #9810, #24954, #36324, #21388, #32929, #7166 ),
 .UNSPECIFIED., .F., .F. ) 
 B_SPLINE_CURVE_WITH_KNOTS ( ( 3, 2, 2, 3 ),
 ( 0.8043478260869539875, 0.8115942028985483336, 0.8188405797101425687, 0.8260869565217369148 ),
 .UNSPECIFIED. ) 
 CURVE ( )  GEOMETRIC_REPRESENTATION_ITEM ( )  RATIONAL_B_SPLINE_CURVE ( ( 1.000000000000047296, 0.8660254037843915231, 1.000000000000000000, 0.8660254037844387076, 1.000000000000000000, 0.8660254037844797859, 0.9999999999999589217 ) ) 
 REPRESENTATION_ITEM ( '' )  );
#6170=AXIS2_PLACEMENT_3D ( 'NONE', #17783, #23283, #25931 ) ;
#6173=CARTESIAN_POINT ( 'NONE',  ( 16.56230152254410370, -6.928203230275506996, -3.374999998770986664 ) ) ;
#6174=CARTESIAN_POINT ( 'NONE',  ( 10.31873187879410914, 0.000000000000000000, -3.740624999385516958 ) ) ;
#6182=FACE_OUTER_BOUND ( 'NONE', #36847, .T. ) ;
#6189=( BOUNDED_CURVE ( )  B_SPLINE_CURVE ( 2, ( #20385, #5580, #34583, #17351, #11832, #37236, #31926 ),
 .UNSPECIFIED., .F., .F. ) 
 B_SPLINE_CURVE_WITH_KNOTS ( ( 3, 2, 2, 3 ),
 ( 0.4999999999999986122, 0.5072463768115930138, 0.5144927536231872489, 0.5217391304347815950 ),
 .UNSPECIFIED. ) 
 CURVE ( )  GEOMETRIC_REPRESENTATION_ITEM ( )  RATIONAL_B_SPLINE_CURVE ( ( 1.000000000000025535, 0.8660254037844129504, 1.000000000000000000, 0.8660254037844387076, 1.000000000000000000, 0.8660254037844571373, 0.9999999999999815703 ) ) 
 REPRESENTATION_ITEM ( '' )  );
#6191=FACE_OUTER_BOUND ( 'NONE', #33107, .T. ) ;
#6196=CARTESIAN_POINT ( 'NONE',  ( 10.56230152254410726, 0.000000000000000000, -4.387499998770999277 ) ) ;
#6207=CARTESIAN_POINT ( 'NONE',  ( 22.80587116629412137, 7.646167579472024665E-16, -8.971874999385509142 ) ) ;
#6209=CARTESIAN_POINT ( 'NONE',  ( 16.56230152254411436, 7.209453229046475009, -2.053124999385520066 ) ) ;
#6212=FACE_OUTER_BOUND ( 'NONE', #22994, .T. ) ;
#6239=CARTESIAN_POINT ( 'NONE',  ( 10.31873187879410736, 0.000000000000000000, -6.440624999385525129 ) ) ;
#6240=ADVANCED_FACE ( 'NONE', ( #2666 ), #26361, .T. ) ;
#6243=EDGE_CURVE ( 'NONE', #35635, #20463, #5695, .T. ) ;
#6244=CARTESIAN_POINT ( 'NONE',  ( 19.56230152254411792, -5.196152422706629359, -1.537499998771035825 ) ) ;
#6246=CARTESIAN_POINT ( 'NONE',  ( 13.56230152254411614, -5.196152422706632912, -6.562499998771037291 ) ) ;
#6265=CARTESIAN_POINT ( 'NONE',  ( 13.56230152254410548, 5.196152422706636465, -7.725000000000036948 ) ) ;
#6267=DIRECTION ( 'NONE',  ( 0.000000000000000000, 0.000000000000000000, 1.000000000000000000 ) ) ;
#6268=CARTESIAN_POINT ( 'NONE',  ( 10.31873187879411091, 0.000000000000000000, -0.1406249993855246405 ) ) ;
#6279=CARTESIAN_POINT ( 'NONE',  ( 22.80587116629411426, 3.604726614523243278, -2.634374999385521221 ) ) ;
#6280=ORIENTED_EDGE ( 'NONE', *, *, #1154, .T. ) ;
#6294=PRODUCT_DEFINITION_FORMATION_WITH_SPECIFIED_SOURCE ( 'ANY', '', #5602, .NOT_KNOWN. ) ;
#6299=CARTESIAN_POINT ( 'NONE',  ( 22.56230152254412147, 3.464101615137759271, -5.587500000000029665 ) ) ;
#6317=CARTESIAN_POINT ( 'NONE',  ( 16.56230152254411436, 7.209453229046482114, -0.7593749993855121172 ) ) ;
#6327=FACE_OUTER_BOUND ( 'NONE', #15458, .T. ) ;
#6343=CARTESIAN_POINT ( 'NONE',  ( 15.52041717089296213, 5.908847349338256727, -9.999738233010948107 ) ) ;
#6351=CARTESIAN_POINT ( 'NONE',  ( 10.31873187879411091, 3.604726614523236616, -8.728124999385524774 ) ) ;
#6363=CARTESIAN_POINT ( 'NONE',  ( 13.44051670066911797, -5.407089921784859143, -4.115624999385558702 ) ) ;
#6389=EDGE_CURVE ( 'NONE', #4918, #21578, #30150, .T. ) ;
#6398=CARTESIAN_POINT ( 'NONE',  ( 13.44051670066911264, 5.407089921784856479, -1.565624999385561988 ) ) ;
#6418=EDGE_LOOP ( 'NONE', ( #27583, #31801, #3275, #29103 ) ) ;
#6429=CARTESIAN_POINT ( 'NONE',  ( 16.56230152254411436, -7.209453229046475009, -4.978124999385539873 ) ) ;
#6434=CARTESIAN_POINT ( 'NONE',  ( 22.56230152254410370, 7.347880794884117764E-16, -6.862499998771004250 ) ) ;
#6440=CARTESIAN_POINT ( 'NONE',  ( 10.31873187879411091, 3.604726614523240613, -3.834374999385520066 ) ) ;
#6445=DIRECTION ( 'NONE',  ( 0.8660254037844224984, 0.000000000000000000, -0.5000000000000278666 ) ) ;
#6451=( BOUNDED_CURVE ( )  B_SPLINE_CURVE ( 2, ( #2471, #10448, #18999, #2102, #30922, #30738, #30556 ),
 .UNSPECIFIED., .F., .F. ) 
 B_SPLINE_CURVE_WITH_KNOTS ( ( 3, 2, 2, 3 ),
 ( 0.8478260869565198421, 0.8550724637681141882, 0.8623188405797084233, 0.8695652173913026584 ),
 .UNSPECIFIED. ) 
 CURVE ( )  GEOMETRIC_REPRESENTATION_ITEM ( )  RATIONAL_B_SPLINE_CURVE ( ( 1.000000000000034861, 0.8660254037844038466, 1.000000000000000000, 0.8660254037844387076, 1.000000000000000000, 0.8660254037844694608, 0.9999999999999692468 ) ) 
 REPRESENTATION_ITEM ( '' )  );
#6473=CARTESIAN_POINT ( 'NONE',  ( 10.31873187879410736, 3.604726614523240613, -3.834374999385520955 ) ) ;
#6483=VERTEX_POINT ( 'NONE', #23518 ) ;
#6490=CARTESIAN_POINT ( 'NONE',  ( 19.56230152254412502, -5.196152422706635576, -6.600000000000050271 ) ) ;
#6498=CARTESIAN_POINT ( 'NONE',  ( 17.25050943477418031, -6.183923782582014361, -9.999999999999998224 ) ) ;
#6506=CARTESIAN_POINT ( 'NONE',  ( 13.44051670066911264, -5.407089921784865361, -3.271874999385554261 ) ) ;
#6519=CARTESIAN_POINT ( 'NONE',  ( 22.80587116629410716, 7.646167579472015790E-16, -0.3656249993855553715 ) ) ;
#6539=CARTESIAN_POINT ( 'NONE',  ( 16.56230152254411081, 7.209453229046475009, -7.903124999385497063 ) ) ;
#6550=CARTESIAN_POINT ( 'NONE',  ( 22.56230152254364185, -3.464101615138027057, -3.299999998771030008 ) ) ;
#6551=CARTESIAN_POINT ( 'NONE',  ( 10.31873187879411091, -3.604726614523240613, -7.303124999385512517 ) ) ;
#6556=VERTEX_POINT ( 'NONE', #9675 ) ;
#6559=CARTESIAN_POINT ( 'NONE',  ( 22.56230152254412502, 7.347880794884125653E-16, -2.925000000000066436 ) ) ;
#6585=CARTESIAN_POINT ( 'NONE',  ( 22.80587116629410716, 3.604726614523238837, -1.678124999385518068 ) ) ;
#6605=VERTEX_POINT ( 'NONE', #37076 ) ;
#6615=CARTESIAN_POINT ( 'NONE',  ( 10.31873187879411091, 3.604726614523236616, -6.478124999385515004 ) ) ;
#6616=( BOUNDED_CURVE ( )  B_SPLINE_CURVE ( 2, ( #1722, #33571, #30913, #19744, #22018, #7607, #16514 ),
 .UNSPECIFIED., .F., .F. ) 
 B_SPLINE_CURVE_WITH_KNOTS ( ( 3, 2, 2, 3 ),
 ( 0.2391304347826091192, 0.2463768115942034653, 0.2536231884057977837, 0.2608695652173921298 ),
 .UNSPECIFIED. ) 
 CURVE ( )  GEOMETRIC_REPRESENTATION_ITEM ( )  RATIONAL_B_SPLINE_CURVE ( ( 0.9999999999999923395, 0.8660254037844463681, 1.000000000000000000, 0.8660254037844387076, 1.000000000000000000, 0.8660254037844232755, 1.000000000000015321 ) ) 
 REPRESENTATION_ITEM ( '' )  );
#6622=CARTESIAN_POINT ( 'NONE',  ( 22.56230152254410370, 3.464101615137755275, -6.374999998771000875 ) ) ;
#6627=CARTESIAN_POINT ( 'NONE',  ( 10.31873187879411091, -3.604726614523244610, -2.859374999385534633 ) ) ;
#6635=FACE_OUTER_BOUND ( 'NONE', #13357, .T. ) ;
#6637=EDGE_LOOP ( 'NONE', ( #9950, #8508, #17913, #32330 ) ) ;
#6642=CARTESIAN_POINT ( 'NONE',  ( 19.56230152254411792, 5.196152422706637353, -7.800000000000029132 ) ) ;
#6654=CARTESIAN_POINT ( 'NONE',  ( 10.56230152254410903, 0.000000000000000000, -7.987499998771019349 ) ) ;
#6656=CARTESIAN_POINT ( 'NONE',  ( 22.80587116629411426, 7.646167579472024665E-16, -7.171874999385541294 ) ) ;
#6677=CARTESIAN_POINT ( 'NONE',  ( 22.56230152254412147, -3.464101615137755275, -6.112500000000051337 ) ) ;
#6689=FACE_OUTER_BOUND ( 'NONE', #35120, .T. ) ;
#6695=CARTESIAN_POINT ( 'NONE',  ( 16.56230152254411081, 7.209453229046482114, -3.909374999385482496 ) ) ;
#6706=CARTESIAN_POINT ( 'NONE',  ( 13.44051670066911619, -5.407089921784859143, -1.415624999385550753 ) ) ;
#6722=CARTESIAN_POINT ( 'NONE',  ( 19.56230152254412147, 5.196152422706637353, -0.6000000000000171863 ) ) ;
#6732=CARTESIAN_POINT ( 'NONE',  ( 22.56230152254410370, 0.000000000000000000, -10.00000000000000000 ) ) ;
#6738=CARTESIAN_POINT ( 'NONE',  ( 13.44051670066911086, 5.407089921784856479, -7.415624999385555860 ) ) ;
#6743=ORIENTED_EDGE ( 'NONE', *, *, #30770, .F. ) ;
#6744=EDGE_LOOP ( 'NONE', ( #31559, #31724, #15749, #3286 ) ) ;
#6771=CARTESIAN_POINT ( 'NONE',  ( 19.68408634441911076, 5.407089921784857367, -5.240624999385545379 ) ) ;
#6802=CARTESIAN_POINT ( 'NONE',  ( 22.80587116629411071, -3.604726614523235284, -5.353124999385542537 ) ) ;
#6808=CARTESIAN_POINT ( 'NONE',  ( 22.56230152254410370, -3.464101615137751278, -6.449999998771025922 ) ) ;
#6813=CARTESIAN_POINT ( 'NONE',  ( 16.56230152254411436, -7.209453229046482114, -5.034374999385487826 ) ) ;
#6817=CARTESIAN_POINT ( 'NONE',  ( 22.56230152254410015, 7.347880794884117764E-16, -7.762499998770988618 ) ) ;
#6828=CARTESIAN_POINT ( 'NONE',  ( 10.56230152254410903, 7.347880794884117764E-16, -10.00000000000000000 ) ) ;
#6842=CARTESIAN_POINT ( 'NONE',  ( 19.56230152254410370, 5.196152422706631135, -8.137499998771001941 ) ) ;
#6844=CARTESIAN_POINT ( 'NONE',  ( 16.56230152254411436, -7.209453229046482114, -5.034374999385487826 ) ) ;
#6868=CARTESIAN_POINT ( 'NONE',  ( 10.56230152254410726, -3.464101615137761048, -7.162500000000031619 ) ) ;
#6876=DIRECTION ( 'NONE',  ( 1.000000000000000000, 0.000000000000000000, 0.000000000000000000 ) ) ;
#6883=ORIENTED_EDGE ( 'NONE', *, *, #3843, .F. ) ;
#6886=CARTESIAN_POINT ( 'NONE',  ( 22.80587116629412847, -3.604726614523238837, -3.159374999385510474 ) ) ;
#6890=AXIS2_PLACEMENT_3D ( 'NONE', #32831, #9152, #6876 ) ;
#6906=AXIS2_PLACEMENT_3D ( 'NONE', #3319, #14890, #285 ) ;
#6916=CARTESIAN_POINT ( 'NONE',  ( 10.56230152254410903, 0.000000000000000000, -5.551115123125782702E-14 ) ) ;
#6936=CARTESIAN_POINT ( 'NONE',  ( 19.68408634441910365, -5.407089921784855591, -5.840624999385535254 ) ) ;
#6941=EDGE_LOOP ( 'NONE', ( #14617, #571, #29123, #37269 ) ) ;
#6956=PRODUCT_DEFINITION ( 'UNKNOWN', '', #6294, #26680 ) ;
#6974=CARTESIAN_POINT ( 'NONE',  ( 22.80587116629411071, -3.604726614523235284, -5.353124999385542537 ) ) ;
#6978=CARTESIAN_POINT ( 'NONE',  ( 22.80587116629411781, -3.604726614523238837, -9.909374999385510918 ) ) ;
#6984=CARTESIAN_POINT ( 'NONE',  ( 13.56230152254410726, 5.196152422706636465, -1.875000000000043299 ) ) ;
#7006=CARTESIAN_POINT ( 'NONE',  ( 13.44051670066911619, -5.407089921784859143, -6.815624999385539340 ) ) ;
#7012=CARTESIAN_POINT ( 'NONE',  ( 19.56230152254411081, -5.196152422706629359, -6.037499998771039600 ) ) ;
#7016=CARTESIAN_POINT ( 'NONE',  ( 13.44051670066911086, 5.407089921784862696, -2.971874999385532234 ) ) ;
#7017=CARTESIAN_POINT ( 'NONE',  ( 22.56230152254458687, 3.464101615137479495, -3.224999998771004961 ) ) ;
#7045=CARTESIAN_POINT ( 'NONE',  ( 22.56230152254410015, 7.347880794884117764E-16, -8.212499998771022547 ) ) ;
#7047=CARTESIAN_POINT ( 'NONE',  ( 13.44051670066910731, 5.407089921784862696, -5.221874999385534011 ) ) ;
#7059=CARTESIAN_POINT ( 'NONE',  ( 15.06230152254410548, 0.000000000000000000, 10.00000000000000000 ) ) ;
#7067=CARTESIAN_POINT ( 'NONE',  ( 13.56230152254411614, -5.196152422706638241, -7.575000000000054357 ) ) ;
#7081=EDGE_LOOP ( 'NONE', ( #31814, #20303, #7169, #36106 ) ) ;
#7084=CARTESIAN_POINT ( 'NONE',  ( 16.56230152254411436, 7.209453229046482114, -3.459374999385518290 ) ) ;
#7088=ORIENTED_EDGE ( 'NONE', *, *, #18149, .T. ) ;
#7107=CARTESIAN_POINT ( 'NONE',  ( 16.56230152254411436, -6.928203230275514990, -0.3375000000000368816 ) ) ;
#7123=CARTESIAN_POINT ( 'NONE',  ( 19.68408634441910721, 5.407089921784857367, -6.590624999385563676 ) ) ;
#7139=CARTESIAN_POINT ( 'NONE',  ( 10.56230152254410903, 0.000000000000000000, -3.937499998770993770 ) ) ;
#7159=CARTESIAN_POINT ( 'NONE',  ( 10.31873187879411091, -3.604726614523240613, -4.153124999385542360 ) ) ;
#7164=CARTESIAN_POINT ( 'NONE',  ( 16.56230152254410726, 0.000000000000000000, -10.00000000000000000 ) ) ;
#7166=CARTESIAN_POINT ( 'NONE',  ( 10.56230152254410726, 0.000000000000000000, -8.550000000000029132 ) ) ;
#7169=ORIENTED_EDGE ( 'NONE', *, *, #9103, .T. ) ;
#7193=CARTESIAN_POINT ( 'NONE',  ( 22.80587116629410716, -3.604726614523235284, -6.703124999385561722 ) ) ;
#7199=CARTESIAN_POINT ( 'NONE',  ( 10.56230152254410903, 0.000000000000000000, -8.437499998771025744 ) ) ;
#7203=CARTESIAN_POINT ( 'NONE',  ( 16.56230152254411436, 7.209453229046482114, -4.359374999385510208 ) ) ;
#7204=CARTESIAN_POINT ( 'NONE',  ( 22.56230152254411792, 7.347880794884125653E-16, -1.575000000000048583 ) ) ;
#7215=CARTESIAN_POINT ( 'NONE',  ( 22.56230152254410370, 7.347880794884115792E-16, 10.00000000000000000 ) ) ;
#7219=CARTESIAN_POINT ( 'NONE',  ( 19.68408634441910721, -5.407089921784855591, -1.790624999385564964 ) ) ;
#7230=CARTESIAN_POINT ( 'NONE',  ( 22.80587116629412492, -3.604726614523238837, -5.409374999385521576 ) ) ;
#7240=CARTESIAN_POINT ( 'NONE',  ( 16.56230152254411436, -6.928203230275506996, -2.024999998770999454 ) ) ;
#7248=CARTESIAN_POINT ( 'NONE',  ( 13.44051670066910908, -5.407089921784859143, -0.5156249993855110958 ) ) ;
#7257=CARTESIAN_POINT ( 'NONE',  ( 22.60184008074515916, 0.09462734519745615025, -10.00000000000000178 ) ) ;
#7263=CARTESIAN_POINT ( 'NONE',  ( 16.56230152254411436, -7.209453229046482114, -5.034374999385487826 ) ) ;
#7279=DIRECTION ( 'NONE',  ( 1.000000000000000000, 0.000000000000000000, 0.000000000000000000 ) ) ;
#7287=CARTESIAN_POINT ( 'NONE',  ( 16.56230152254412147, 6.928203230275514990, -0.5625000000000506262 ) ) ;
#7305=CARTESIAN_POINT ( 'NONE',  ( 22.80587116629410716, 3.604726614523238837, -7.978124999385491023 ) ) ;
#7323=CARTESIAN_POINT ( 'NONE',  ( 10.56230152254411081, 0.000000000000000000, -2.137499998771025034 ) ) ;
#7344=CARTESIAN_POINT ( 'NONE',  ( 22.80587116629410716, 7.646167579472015790E-16, -3.065624999385535787 ) ) ;
#7348=CARTESIAN_POINT ( 'NONE',  ( 22.80587116629411071, 3.604726614523243278, -9.384374999385521221 ) ) ;
#7353=CARTESIAN_POINT ( 'NONE',  ( 10.31873187879410736, 0.000000000000000000, -0.6468749993855105185 ) ) ;
#7360=CARTESIAN_POINT ( 'NONE',  ( 10.56230152254410903, 0.000000000000000000, -3.937499998770993770 ) ) ;
#7375=CARTESIAN_POINT ( 'NONE',  ( 19.68408634441910721, 5.407089921784857367, -7.940624999385553551 ) ) ;
#7381=CARTESIAN_POINT ( 'NONE',  ( 10.56230152254411081, 0.000000000000000000, -7.537499998771012955 ) ) ;
#7383=CARTESIAN_POINT ( 'NONE',  ( 19.68408634441911431, 5.407089921784862696, -5.296874999385526195 ) ) ;
#7384=CARTESIAN_POINT ( 'NONE',  ( 13.56230152254411614, -5.196152422706638241, -1.725000000000059819 ) ) ;
#7389=CARTESIAN_POINT ( 'NONE',  ( 10.56230152254410726, 0.000000000000000000, -3.150000000000041656 ) ) ;
#7409=CARTESIAN_POINT ( 'NONE',  ( 13.56230152254410903, 5.196152422706636465, -2.325000000000049027 ) ) ;
#7412=CARTESIAN_POINT ( 'NONE',  ( 16.56230152254411792, 7.209453229046482114, -7.059374999385484628 ) ) ;
#7417=CARTESIAN_POINT ( 'NONE',  ( 13.44051670066911441, 5.407089921784856479, -0.6656249993855500868 ) ) ;
#7427=CARTESIAN_POINT ( 'NONE',  ( 10.31873187879410736, 0.000000000000000000, -10.09687499938552513 ) ) ;
#7435=CARTESIAN_POINT ( 'NONE',  ( 22.56230152254412857, -3.464101615137755275, -8.812500000000058620 ) ) ;
#7448=CARTESIAN_POINT ( 'NONE',  ( 16.56230152254411436, -7.209453229046482114, -5.934374999385510385 ) ) ;
#7456=CARTESIAN_POINT ( 'NONE',  ( 19.56230152254410370, 5.196152422706631135, -9.487499998770992704 ) ) ;
#7462=EDGE_CURVE ( 'NONE', #11777, #8243, #28691, .T. ) ;
#7464=CARTESIAN_POINT ( 'NONE',  ( 13.56230152254411792, -5.196152422706638241, -6.225000000000063594 ) ) ;
#7471=CARTESIAN_POINT ( 'NONE',  ( 22.56230152254411792, 3.464101615137759271, -1.537500000000068257 ) ) ;
#7476=CARTESIAN_POINT ( 'NONE',  ( 22.56230152254410370, 7.347880794884117764E-16, -8.662499998771028942 ) ) ;
#7489=CARTESIAN_POINT ( 'NONE',  ( 10.31873187879410914, 0.000000000000000000, -8.690624999385526905 ) ) ;
#7505=CIRCLE ( 'NONE', #6906, 8.000000000000000000 ) ;
#7530=CARTESIAN_POINT ( 'NONE',  ( 19.68408634441910365, 5.407089921784857367, -4.340624999385561900 ) ) ;
#7540=CARTESIAN_POINT ( 'NONE',  ( 16.56230152254411436, 7.209453229046482114, -1.209374999385475657 ) ) ;
#7561=CARTESIAN_POINT ( 'NONE',  ( 10.31873187879410736, 0.000000000000000000, -6.890624999385530636 ) ) ;
#7566=CARTESIAN_POINT ( 'NONE',  ( 22.56230152254410370, 3.464101615137755275, -8.624999998771011533 ) ) ;
#7570=CARTESIAN_POINT ( 'NONE',  ( 16.56230152254411436, -7.209453229046482114, -6.384374999385507010 ) ) ;
#7574=CARTESIAN_POINT ( 'NONE',  ( 10.56230152254394916, 3.464101615137665124, -5.887500000000066791 ) ) ;
#7585=CARTESIAN_POINT ( 'NONE',  ( 16.56230152254410726, 0.000000000000000000, -10.00000000000000000 ) ) ;
#7591=ORIENTED_EDGE ( 'NONE', *, *, #12440, .T. ) ;
#7599=CARTESIAN_POINT ( 'NONE',  ( 10.31873187879410736, 0.000000000000000000, -7.396874999385516958 ) ) ;
#7603=CARTESIAN_POINT ( 'NONE',  ( 13.44051670066911264, 5.407089921784856479, -1.565624999385561988 ) ) ;
#7607=CARTESIAN_POINT ( 'NONE',  ( 10.56230152254371824, -3.464101615137527457, -2.999999998771021748 ) ) ;
#7610=CARTESIAN_POINT ( 'NONE',  ( 22.56230152254410370, 3.464101615137755275, -2.324999998771006826 ) ) ;
#7612=AXIS2_PLACEMENT_3D ( 'NONE', #15047, #31914, #17523 ) ;
#7619=CARTESIAN_POINT ( 'NONE',  ( 22.56230152254412857, -3.464101615137755275, -8.362500000000061107 ) ) ;
#7636=CARTESIAN_POINT ( 'NONE',  ( 10.31873187879410558, 0.000000000000000000, -6.496874999385504168 ) ) ;
#7641=( BOUNDED_CURVE ( )  B_SPLINE_CURVE ( 2, ( #21947, #4123, #27247, #18166, #33122, #33311, #26867 ),
 .UNSPECIFIED., .F., .F. ) 
 B_SPLINE_CURVE_WITH_KNOTS ( ( 3, 2, 2, 3 ),
 ( 0.7173913043478248319, 0.7246376811594200662, 0.7318840579710154115, 0.7391304347826105348 ),
 .UNSPECIFIED. ) 
 CURVE ( )  GEOMETRIC_REPRESENTATION_ITEM ( )  RATIONAL_B_SPLINE_CURVE ( ( 1.000000000000022649, 0.8660254037844161701, 1.000000000000000000, 0.8660254037844387076, 1.000000000000000000, 0.8660254037844038466, 1.000000000000034861 ) ) 
 REPRESENTATION_ITEM ( '' )  );
#7653=CYLINDRICAL_SURFACE ( 'NONE', #4660, 5.999999999999998224 ) ;
#7661=CARTESIAN_POINT ( 'NONE',  ( 13.56230152254410903, 5.196152422706636465, -2.325000000000049027 ) ) ;
#7667=DIRECTION ( 'NONE',  ( 1.000000000000000000, 0.000000000000000000, 0.000000000000000000 ) ) ;
#7677=CARTESIAN_POINT ( 'NONE',  ( 22.80587116629410716, 3.604726614523238837, -8.878124999385544669 ) ) ;
#7713=CARTESIAN_POINT ( 'NONE',  ( 10.31873187879411446, 3.604726614523236616, -6.928124999385510741 ) ) ;
#7720=CARTESIAN_POINT ( 'NONE',  ( 22.56230152254332921, 3.464101615138219348, -6.937500000000038192 ) ) ;
#7722=CARTESIAN_POINT ( 'NONE',  ( 16.56230152254411436, -7.209453229046482114, -1.434374999385489735 ) ) ;
#7743=CARTESIAN_POINT ( 'NONE',  ( 19.68408634441910721, -5.407089921784855591, -6.740624999385547156 ) ) ;
#7749=CARTESIAN_POINT ( 'NONE',  ( 10.56230152254411436, -3.464101615137757051, -9.299999998770987375 ) ) ;
#7754=CARTESIAN_POINT ( 'NONE',  ( 16.56230152254411436, -7.209453229046482114, -5.484374999385515537 ) ) ;
#7755=CARTESIAN_POINT ( 'NONE',  ( 19.56230152254412502, -5.196152422706635576, -1.650000000000068079 ) ) ;
#7786=CARTESIAN_POINT ( 'NONE',  ( 22.80587116629411781, 3.604726614523243278, -8.034374999385502036 ) ) ;
#7790=CARTESIAN_POINT ( 'NONE',  ( 16.56230152254411436, -7.209453229046475009, -1.378124999385542226 ) ) ;
#7793=CARTESIAN_POINT ( 'NONE',  ( 22.56230152254429555, 3.464101615137640255, -2.774999998771005227 ) ) ;
#7797=CARTESIAN_POINT ( 'NONE',  ( 16.56230152254411436, 6.928203230275506996, -1.349999998771021614 ) ) ;
#7804=EDGE_CURVE ( 'NONE', #11542, #28877, #6451, .T. ) ;
#7805=DIRECTION ( 'NONE',  ( -1.000000000000000000, 0.000000000000000000, 0.000000000000000000 ) ) ;
#7807=CARTESIAN_POINT ( 'NONE',  ( 19.56230152254411792, 5.196152422706637353, -8.700000000000041922 ) ) ;
#7808=VERTEX_POINT ( 'NONE', #1729 ) ;
#7809=CARTESIAN_POINT ( 'NONE',  ( 10.56230152254410726, 0.000000000000000000, -3.600000000000047606 ) ) ;
#7822=CARTESIAN_POINT ( 'NONE',  ( 22.80587116629411781, 7.646167579472024665E-16, -5.821874999385522997 ) ) ;
#7828=CARTESIAN_POINT ( 'NONE',  ( 22.80587116629412492, -3.604726614523238837, -2.259374999385487470 ) ) ;
#7830=CARTESIAN_POINT ( 'NONE',  ( 10.56230152254581078, 3.464101615138732715, -9.374999998771002652 ) ) ;
#7836=( BOUNDED_CURVE ( )  B_SPLINE_CURVE ( 2, ( #13330, #19225, #22056, #24888, #4974, #27914, #25072 ),
 .UNSPECIFIED., .F., .F. ) 
 B_SPLINE_CURVE_WITH_KNOTS ( ( 3, 2, 2, 3 ),
 ( 0.9130434782608684019, 0.9202898550724627480, 0.9275362318840569831, 0.9347826086956513292 ),
 .UNSPECIFIED. ) 
 CURVE ( )  GEOMETRIC_REPRESENTATION_ITEM ( )  RATIONAL_B_SPLINE_CURVE ( ( 1.000000000000020428, 0.8660254037844181685, 1.000000000000000000, 0.8660254037844387076, 1.000000000000000000, 0.8660254037844551389, 0.9999999999999835687 ) ) 
 REPRESENTATION_ITEM ( '' )  );
#7846=CARTESIAN_POINT ( 'NONE',  ( 19.56230152254411792, 5.196152422706637353, -2.850000000000019185 ) ) ;
#7856=( BOUNDED_CURVE ( )  B_SPLINE_CURVE ( 2, ( #4081, #15653, #15273, #9955, #1608, #23996, #35725 ),
 .UNSPECIFIED., .F., .F. ) 
 B_SPLINE_CURVE_WITH_KNOTS ( ( 3, 2, 2, 3 ),
 ( 0.1956521739130460125, 0.2028985507246403308, 0.2101449275362346492, 0.2173913043478289675 ),
 .UNSPECIFIED. ) 
 CURVE ( )  GEOMETRIC_REPRESENTATION_ITEM ( )  RATIONAL_B_SPLINE_CURVE ( ( 0.9999999999999533706, 0.8660254037844854480, 1.000000000000000000, 0.8660254037844387076, 1.000000000000000000, 0.8660254037843853059, 1.000000000000053291 ) ) 
 REPRESENTATION_ITEM ( '' )  );
#7864=CARTESIAN_POINT ( 'NONE',  ( 10.31873187879410914, 0.000000000000000000, -8.240624999385548932 ) ) ;
#7868=VERTEX_POINT ( 'NONE', #4574 ) ;
#7875=CARTESIAN_POINT ( 'NONE',  ( 22.56230152254412147, 7.347880794884125653E-16, -4.275000000000028777 ) ) ;
#7886=MANIFOLD_SOLID_BREP ( 'Cavity1', #13224 ) ;
#7902=CARTESIAN_POINT ( 'NONE',  ( 19.68408634441910365, -5.407089921784855591, -6.290624999385540761 ) ) ;
#7911=CARTESIAN_POINT ( 'NONE',  ( 16.56230152254411436, -7.209453229046482114, -1.884374999385517446 ) ) ;
#7917=CARTESIAN_POINT ( 'NONE',  ( 22.80587116629411071, 3.604726614523238837, -2.128124999385546001 ) ) ;
#7938=CARTESIAN_POINT ( 'NONE',  ( 13.56230152254411436, -5.196152422706632912, -8.362499998771033560 ) ) ;
#7942=CARTESIAN_POINT ( 'NONE',  ( 19.68408634441911431, -5.407089921784861808, -6.346874999385549110 ) ) ;
#7957=DIRECTION ( 'NONE',  ( 1.000000000000000000, 0.000000000000000000, 0.000000000000000000 ) ) ;
#7966=DIRECTION ( 'NONE',  ( 1.000000000000000000, 0.000000000000000000, 0.000000000000000000 ) ) ;
#7971=CARTESIAN_POINT ( 'NONE',  ( 13.44051670066911264, -5.407089921784865361, -8.221874999385537564 ) ) ;
#7975=CARTESIAN_POINT ( 'NONE',  ( 22.80587116629410360, 7.646167579472015790E-16, -2.615624999385557370 ) ) ;
#7982=CARTESIAN_POINT ( 'NONE',  ( 13.56230152254411436, -5.196152422706632912, -1.612499998771027565 ) ) ;
#7987=CARTESIAN_POINT ( 'NONE',  ( 16.56230152254410726, 0.000000000000000000, 10.00000000000000000 ) ) ;
#7989=CARTESIAN_POINT ( 'NONE',  ( 16.56230152254411081, 6.928203230275514990, -9.112500000000034461 ) ) ;
#8000=CARTESIAN_POINT ( 'NONE',  ( 10.56230152254379107, 3.464101615137573198, -3.637500000000023714 ) ) ;
#8003=ORIENTED_EDGE ( 'NONE', *, *, #9607, .F. ) ;
#8006=CARTESIAN_POINT ( 'NONE',  ( 19.68408634441911431, -5.407089921784861808, -5.896874999385542715 ) ) ;
#8010=CARTESIAN_POINT ( 'NONE',  ( 13.44051670066911264, -5.407089921784865361, -2.371874999385514826 ) ) ;
#8015=CARTESIAN_POINT ( 'NONE',  ( 19.56230152254410726, 5.196152422706631135, -0.4874999987710126881 ) ) ;
#8022=DIRECTION ( 'NONE',  ( 1.000000000000000000, 0.000000000000000000, 0.000000000000000000 ) ) ;
#8030=CARTESIAN_POINT ( 'NONE',  ( 10.56230152254411614, -3.464101615137761048, -2.662500000000041833 ) ) ;
#8046=CARTESIAN_POINT ( 'NONE',  ( 16.56230152254411436, -6.928203230275514990, -7.087500000000036771 ) ) ;
#8050=CARTESIAN_POINT ( 'NONE',  ( 19.68408634441910365, 5.407089921784857367, -9.740624999385548932 ) ) ;
#8089=CARTESIAN_POINT ( 'NONE',  ( 22.80587116629410716, -3.604726614523235284, -6.703124999385561722 ) ) ;
#8097=CARTESIAN_POINT ( 'NONE',  ( 10.56230152254410726, 0.000000000000000000, -6.637499998771001941 ) ) ;
#8104=CARTESIAN_POINT ( 'NONE',  ( 10.31873187879410914, 0.000000000000000000, -1.490624999385542493 ) ) ;
#8132=FACE_OUTER_BOUND ( 'NONE', #18180, .T. ) ;
#8135=CARTESIAN_POINT ( 'NONE',  ( 13.44051670066911441, -5.407089921784865361, -7.321874999385524774 ) ) ;
#8136=CARTESIAN_POINT ( 'NONE',  ( 16.56230152254410726, 0.000000000000000000, -10.00000000000000000 ) ) ;
#8137=CARTESIAN_POINT ( 'NONE',  ( 10.56230152254410903, 7.347880794884117764E-16, -10.00000000000000000 ) ) ;
#8143=ORIENTED_EDGE ( 'NONE', *, *, #26746, .T. ) ;
#8161=CARTESIAN_POINT ( 'NONE',  ( 13.70341545108635195, -5.565789069430963742, -9.999999999999987566 ) ) ;
#8163=CARTESIAN_POINT ( 'NONE',  ( 22.80587116629411781, -3.604726614523238837, -8.559374999385489957 ) ) ;
#8166=CARTESIAN_POINT ( 'NONE',  ( 19.68408634441910721, 5.407089921784857367, -3.890624999385555505 ) ) ;
#8169=CARTESIAN_POINT ( 'NONE',  ( 22.56230152254410015, 7.347880794884117764E-16, -2.812499998771006204 ) ) ;
#8172=CARTESIAN_POINT ( 'NONE',  ( 22.56230152254410370, 7.347880794884117764E-16, -4.612499998771030008 ) ) ;
#8180=CARTESIAN_POINT ( 'NONE',  ( 10.31873187879411091, 0.000000000000000000, -2.840624999385532590 ) ) ;
#8183=CARTESIAN_POINT ( 'NONE',  ( 22.56230152254411792, 7.347880794884125653E-16, -7.875000000000048850 ) ) ;
#8196=CARTESIAN_POINT ( 'NONE',  ( 16.56230152254411436, 7.209453229046482114, -6.609374999385519978 ) ) ;
#8200=CARTESIAN_POINT ( 'NONE',  ( 13.44051670066911264, -5.407089921784865361, -1.471874999385502925 ) ) ;
#8202=CARTESIAN_POINT ( 'NONE',  ( 13.56230152254410370, 5.196152422706630247, -9.412499998771028942 ) ) ;
#8207=DIRECTION ( 'NONE',  ( 1.000000000000000000, 0.000000000000000000, 0.000000000000000000 ) ) ;
#8219=CARTESIAN_POINT ( 'NONE',  ( 19.56230152254412147, 5.196152422706637353, -1.050000000000023137 ) ) ;
#8220=CARTESIAN_POINT ( 'NONE',  ( 16.56230152254410726, 0.000000000000000000, -10.00000000000000000 ) ) ;
#8221=ORIENTED_EDGE ( 'NONE', *, *, #32635, .T. ) ;
#8228=LINE ( 'NONE', #10875, #19489 ) ;
#8229=DIRECTION ( 'NONE',  ( 0.000000000000000000, 0.000000000000000000, 1.000000000000000000 ) ) ;
#8239=CARTESIAN_POINT ( 'NONE',  ( 15.47811703177229070, 6.148715791637009431, -10.14010138606053424 ) ) ;
#8243=VERTEX_POINT ( 'NONE', #13964 ) ;
#8245=VERTEX_POINT ( 'NONE', #37432 ) ;
#8272=CARTESIAN_POINT ( 'NONE',  ( 13.44051670066911619, -5.407089921784859143, -6.815624999385539340 ) ) ;
#8281=CARTESIAN_POINT ( 'NONE',  ( 22.80587116629411426, 7.646167579472024665E-16, -2.671874999385509319 ) ) ;
#8287=CARTESIAN_POINT ( 'NONE',  ( 13.44051670066911441, -5.407089921784859143, -1.865624999385528948 ) ) ;
#8317=CARTESIAN_POINT ( 'NONE',  ( 22.80587116629411071, 3.604726614523243278, -8.934374999385493510 ) ) ;
#8326=ORIENTED_EDGE ( 'NONE', *, *, #13190, .T. ) ;
#8348=CARTESIAN_POINT ( 'NONE',  ( 10.31873187879411091, 3.604726614523236616, -2.428124999385521843 ) ) ;
#8351=CARTESIAN_POINT ( 'NONE',  ( 10.56230152254328125, -3.464101615137274326, -1.649999998771008114 ) ) ;
#8354=CARTESIAN_POINT ( 'NONE',  ( 22.56230152254411436, -3.464101615137751278, -2.849999998770996967 ) ) ;
#8364=CARTESIAN_POINT ( 'NONE',  ( 13.44051670066911086, 5.407089921784856479, -2.015624999385540406 ) ) ;
#8380=CARTESIAN_POINT ( 'NONE',  ( 22.80587116629411781, 3.604726614523243278, -8.034374999385502036 ) ) ;
#8385=CARTESIAN_POINT ( 'NONE',  ( 22.80587116629412492, -3.604726614523238837, -0.4593749993855362757 ) ) ;
#8397=DIRECTION ( 'NONE',  ( 0.000000000000000000, 0.000000000000000000, 1.000000000000000000 ) ) ;
#8403=CARTESIAN_POINT ( 'NONE',  ( 22.56230152254412857, -3.464101615137755275, -3.412500000000044942 ) ) ;
#8405=ORIENTED_EDGE ( 'NONE', *, *, #15976, .T. ) ;
#8420=CARTESIAN_POINT ( 'NONE',  ( 22.80587116629412847, -3.604726614523238837, -2.259374999385487026 ) ) ;
#8426=ORIENTED_EDGE ( 'NONE', *, *, #9103, .F. ) ;
#8453=CARTESIAN_POINT ( 'NONE',  ( 13.44051670066911264, 5.407089921784856479, -5.615624999385532057 ) ) ;
#8459=LINE ( 'NONE', #34422, #29898 ) ;
#8466=CARTESIAN_POINT ( 'NONE',  ( 22.80587116629410716, 3.604726614523238837, -3.028124999385537475 ) ) ;
#8477=EDGE_CURVE ( 'NONE', #21699, #31946, #11872, .T. ) ;
#8495=CARTESIAN_POINT ( 'NONE',  ( 10.56230152254410726, 0.000000000000000000, -7.087499998771007448 ) ) ;
#8499=CARTESIAN_POINT ( 'NONE',  ( 22.80587116629412492, 3.604726614523243278, -8.484374999385497773 ) ) ;
#8501=AXIS2_PLACEMENT_3D ( 'NONE', #19783, #13896, #30589 ) ;
#8508=ORIENTED_EDGE ( 'NONE', *, *, #23537, .T. ) ;
#8530=CARTESIAN_POINT ( 'NONE',  ( 10.31873187879410381, 3.604726614523236616, -2.878124999385517135 ) ) ;
#8534=CARTESIAN_POINT ( 'NONE',  ( 22.56230152254410370, 3.464101615137755275, -4.124999998771022192 ) ) ;
#8544=CARTESIAN_POINT ( 'NONE',  ( 13.56230152254410548, 5.196152422706630247, -8.962499998770995902 ) ) ;
#8550=CARTESIAN_POINT ( 'NONE',  ( 16.56230152254410726, 0.000000000000000000, 10.00000000000000000 ) ) ;
#8553=CARTESIAN_POINT ( 'NONE',  ( 13.56230152254411436, -5.196152422706632912, -5.662499998771053811 ) ) ;
#8555=CARTESIAN_POINT ( 'NONE',  ( 22.56230152254410370, 7.347880794884117764E-16, -1.912499998771022280 ) ) ;
#8561=CARTESIAN_POINT ( 'NONE',  ( 16.56230152254411436, 7.209453229046482114, -9.309374999385527261 ) ) ;
#8566=CARTESIAN_POINT ( 'NONE',  ( 10.31873187879410736, 3.604726614523240613, -2.034374999385505145 ) ) ;
#8575=ORIENTED_EDGE ( 'NONE', *, *, #34130, .T. ) ;
#8582=CARTESIAN_POINT ( 'NONE',  ( 16.56230152254411436, 6.928203230275514990, -4.612500000000012257 ) ) ;
#8600=CARTESIAN_POINT ( 'NONE',  ( 13.44051670066911264, -5.407089921784865361, -1.921874999385508875 ) ) ;
#8631=EDGE_CURVE ( 'NONE', #9681, #2980, #21968, .T. ) ;
#8636=CARTESIAN_POINT ( 'NONE',  ( 10.31873187879410914, 0.000000000000000000, -9.590624999385537919 ) ) ;
#8650=CARTESIAN_POINT ( 'NONE',  ( 16.56230152254411081, -7.209453229046475009, -3.628124999385552663 ) ) ;
#8666=CARTESIAN_POINT ( 'NONE',  ( 22.56230152254411792, 7.347880794884125653E-16, -7.425000000000042455 ) ) ;
#8669=CARTESIAN_POINT ( 'NONE',  ( 10.31873187879411269, 3.604726614523236616, -9.178124999385522287 ) ) ;
#8682=CARTESIAN_POINT ( 'NONE',  ( 19.68408634441911431, -5.407089921784861808, -9.946874999385540761 ) ) ;
#8685=FACE_BOUND ( 'NONE', #9692, .T. ) ;
#8706=CARTESIAN_POINT ( 'NONE',  ( 16.56230152254411436, -6.928203230275514990, -3.037500000000043165 ) ) ;
#8713=CARTESIAN_POINT ( 'NONE',  ( 19.68408634441910365, 5.407089921784857367, -2.990624999385543603 ) ) ;
#8719=CARTESIAN_POINT ( 'NONE',  ( 16.56230152254410015, -6.928203230275506996, -3.374999998770986664 ) ) ;
#8725=CARTESIAN_POINT ( 'NONE',  ( 22.56230152254412147, 7.347880794884125653E-16, -8.325000000000027711 ) ) ;
#8728=CARTESIAN_POINT ( 'NONE',  ( 10.56230152254410726, 0.000000000000000000, -5.400000000000043876 ) ) ;
#8731=CARTESIAN_POINT ( 'NONE',  ( 13.56230152254411614, -5.196152422706632912, -4.762499998771041021 ) ) ;
#8741=CARTESIAN_POINT ( 'NONE',  ( 22.56230152254410370, 7.347880794884117764E-16, -5.512499998771014376 ) ) ;
#8748=CARTESIAN_POINT ( 'NONE',  ( 22.80587116629412137, 7.646167579472024665E-16, -8.521874999385502747 ) ) ;
#8752=CARTESIAN_POINT ( 'NONE',  ( 22.80587116629412492, -3.604726614523238837, -4.059374999385534366 ) ) ;
#8764=CARTESIAN_POINT ( 'NONE',  ( 10.56230152254366672, 3.464101615137503920, -1.387500000000010170 ) ) ;
#8771=CARTESIAN_POINT ( 'NONE',  ( 19.56230152254411792, 5.196152422706637353, -4.200000000000036593 ) ) ;
#8772=ORIENTED_EDGE ( 'NONE', *, *, #7462, .F. ) ;
#8790=CARTESIAN_POINT ( 'NONE',  ( 10.31873187879410736, 3.604726614523240613, -2.034374999385505145 ) ) ;
#8823=CARTESIAN_POINT ( 'NONE',  ( 13.44051670066910908, 5.407089921784856479, -10.11562499938553650 ) ) ;
#8825=CARTESIAN_POINT ( 'NONE',  ( 10.56230152254410726, 0.000000000000000000, -8.550000000000029132 ) ) ;
#8827=CARTESIAN_POINT ( 'NONE',  ( 10.82125134821038337, -2.451055655723595184, -9.999999999999994671 ) ) ;
#8836=CARTESIAN_POINT ( 'NONE',  ( 22.56230152254410726, 7.347880794884117764E-16, -3.262499998771012599 ) ) ;
#8837=CARTESIAN_POINT ( 'NONE',  ( 13.44051670066911264, 5.407089921784856479, -5.615624999385532057 ) ) ;
#8852=CARTESIAN_POINT ( 'NONE',  ( 16.56230152254410726, 0.000000000000000000, -10.00000000000000000 ) ) ;
#8862=CARTESIAN_POINT ( 'NONE',  ( 19.56230152254411436, -5.196152422706629359, -8.287499998771014731 ) ) ;
#8866=CARTESIAN_POINT ( 'NONE',  ( 16.56230152254411436, 7.209453229046482114, -9.309374999385527261 ) ) ;
#8879=CARTESIAN_POINT ( 'NONE',  ( 16.56230152254411436, 6.928203230275514990, -4.162500000000016520 ) ) ;
#8895=CARTESIAN_POINT ( 'NONE',  ( 10.31873187879410736, -3.604726614523240613, -5.953124999385525307 ) ) ;
#8901=CARTESIAN_POINT ( 'NONE',  ( 16.56230152254410726, -6.928203230275506996, -4.274999998770977250 ) ) ;
#8917=CARTESIAN_POINT ( 'NONE',  ( 18.06230152254410726, 1.836970198721029441E-16, 0.000000000000000000 ) ) ;
#8931=CARTESIAN_POINT ( 'NONE',  ( 13.44051670066911264, -5.407089921784865361, -8.671874999385515537 ) ) ;
#8934=CARTESIAN_POINT ( 'NONE',  ( 22.56230152254473253, -3.464101615137399115, -1.162500000000026512 ) ) ;
#8936=CARTESIAN_POINT ( 'NONE',  ( 22.80587116629412492, 3.604726614523243278, -4.884374999385530991 ) ) ;
#8937=EDGE_LOOP ( 'NONE', ( #6883, #162, #19240, #14606 ) ) ;
#8943=VECTOR ( 'NONE', #36979, 1000.000000000000000 ) ;
#8952=CARTESIAN_POINT ( 'NONE',  ( 10.56230152254410903, 0.000000000000000000, -7.987499998771019349 ) ) ;
#8958=CARTESIAN_POINT ( 'NONE',  ( 22.56230152254412147, 7.347880794884125653E-16, -3.825000000000050804 ) ) ;
#8975=CARTESIAN_POINT ( 'NONE',  ( 16.56230152254411436, 7.209453229046482114, -2.109374999385531080 ) ) ;
#8986=ADVANCED_FACE ( 'NONE', ( #2344 ), #19979, .F. ) ;
#9001=DIRECTION ( 'NONE',  ( 1.000000000000000000, 0.000000000000000000, 0.000000000000000000 ) ) ;
#9008=CARTESIAN_POINT ( 'NONE',  ( 13.44051670066911441, -5.407089921784859143, -8.615624999385563143 ) ) ;
#9011=CARTESIAN_POINT ( 'NONE',  ( 10.44739295067906681, -1.007476398167555631, -10.00000000000000000 ) ) ;
#9021=CARTESIAN_POINT ( 'NONE',  ( 10.31873187879411091, 3.604726614523236616, -5.128124999385527794 ) ) ;
#9027=ORIENTED_EDGE ( 'NONE', *, *, #33003, .T. ) ;
#9028=ORIENTED_EDGE ( 'NONE', *, *, #20849, .T. ) ;
#9056=CARTESIAN_POINT ( 'NONE',  ( 13.44051670066910908, 5.407089921784862696, -9.271874999385531169 ) ) ;
#9058=CARTESIAN_POINT ( 'NONE',  ( 22.80587116629411071, -3.604726614523235284, -2.653124999385503724 ) ) ;
#9084=VECTOR ( 'NONE', #26243, 1000.000000000000000 ) ;
#9088=CARTESIAN_POINT ( 'NONE',  ( 10.31873187879411269, -3.604726614523240613, -6.403124999385521043 ) ) ;
#9094=CARTESIAN_POINT ( 'NONE',  ( 19.56230152254411081, -5.196152422706629359, -5.137499998771027698 ) ) ;
#9103=EDGE_CURVE ( 'NONE', #36001, #33455, #8228, .T. ) ;
#9105=CARTESIAN_POINT ( 'NONE',  ( 16.56230152254410726, 0.000000000000000000, -10.00000000000000000 ) ) ;
#9111=( BOUNDED_CURVE ( )  B_SPLINE_CURVE ( 2, ( #28484, #11430, #26198, #22816, #19977, #14279, #5544 ),
 .UNSPECIFIED., .F., .F. ) 
 B_SPLINE_CURVE_WITH_KNOTS ( ( 3, 2, 2, 3 ),
 ( 0.6086956521739131931, 0.6159420289855074282, 0.6231884057971016633, 0.6304347826086960094 ),
 .UNSPECIFIED. ) 
 CURVE ( )  GEOMETRIC_REPRESENTATION_ITEM ( )  RATIONAL_B_SPLINE_CURVE ( ( 0.9999999999999980016, 0.8660254037844407060, 1.000000000000000000, 0.8660254037844387076, 1.000000000000000000, 0.8660254037844326014, 1.000000000000006217 ) ) 
 REPRESENTATION_ITEM ( '' )  );
#9115=DIRECTION ( 'NONE',  ( 0.000000000000000000, 0.000000000000000000, 1.000000000000000000 ) ) ;
#9117=CARTESIAN_POINT ( 'NONE',  ( 10.31873187879411091, 3.604726614523236616, -0.6281249993855065883 ) ) ;
#9128=CARTESIAN_POINT ( 'NONE',  ( 16.56230152254411436, 7.209453229046482114, -3.009374999385522553 ) ) ;
#9146=CARTESIAN_POINT ( 'NONE',  ( 13.56230152254410903, 5.196152422706636465, -5.475000000000035172 ) ) ;
#9149=CARTESIAN_POINT ( 'NONE',  ( 22.56230152254467924, 3.464101615137418211, -5.474999998770981868 ) ) ;
#9152=DIRECTION ( 'NONE',  ( 0.000000000000000000, 0.000000000000000000, 1.000000000000000000 ) ) ;
#9154=CARTESIAN_POINT ( 'NONE',  ( 10.56230152254410726, 0.000000000000000000, -5.850000000000049383 ) ) ;
#9164=CARTESIAN_POINT ( 'NONE',  ( 22.80587116629411781, -3.604726614523238837, -2.709374999385515181 ) ) ;
#9174=ADVANCED_FACE ( 'NONE', ( #14650 ), #11989, .F. ) ;
#9190=CYLINDRICAL_SURFACE ( 'NONE', #13197, 5.999999999999998224 ) ;
#9198=CARTESIAN_POINT ( 'NONE',  ( 22.80587116629410716, 3.604726614523238837, -8.878124999385544669 ) ) ;
#9201=CARTESIAN_POINT ( 'NONE',  ( 10.41621459261286198, -0.7567938363388677647, -9.999999999999998224 ) ) ;
#9209=CARTESIAN_POINT ( 'NONE',  ( 22.80587116629411426, 3.604726614523238837, -3.928124999385561367 ) ) ;
#9218=CARTESIAN_POINT ( 'NONE',  ( 24.56230152254410726, 0.000000000000000000, -10.00000000000000000 ) ) ;
#9230=DIRECTION ( 'NONE',  ( 0.000000000000000000, 0.000000000000000000, 1.000000000000000000 ) ) ;
#9244=CARTESIAN_POINT ( 'NONE',  ( 10.31873187879410914, 0.000000000000000000, -1.490624999385542493 ) ) ;
#9264=VERTEX_POINT ( 'NONE', #9154 ) ;
#9276=CARTESIAN_POINT ( 'NONE',  ( 16.56230152254411081, -7.209453229046475009, -5.878124999385531346 ) ) ;
#9282=CARTESIAN_POINT ( 'NONE',  ( 10.56230152254410726, 0.000000000000000000, -7.087499998771007448 ) ) ;
#9287=CARTESIAN_POINT ( 'NONE',  ( 10.31873187879410736, -3.604726614523244610, -3.309374999385498395 ) ) ;
#9317=CARTESIAN_POINT ( 'NONE',  ( 10.31873187879410381, 3.604726614523240613, -3.384374999385492799 ) ) ;
#9320=APPLICATION_CONTEXT ( 'automotive_design' ) ;
#9327=ORIENTED_EDGE ( 'NONE', *, *, #31021, .F. ) ;
#9332=MECHANICAL_DESIGN_GEOMETRIC_PRESENTATION_REPRESENTATION('',(#3886),#34137);
#9338=CARTESIAN_POINT ( 'NONE',  ( 22.56230152254411792, 3.464101615137759271, -6.487500000000020250 ) ) ;
#9345=CARTESIAN_POINT ( 'NONE',  ( 22.45414455245212793, -1.393728951354829659, -10.00000000000000533 ) ) ;
#9353=CARTESIAN_POINT ( 'NONE',  ( 22.80587116629412137, 7.646167579472024665E-16, -4.021874999385527616 ) ) ;
#9361=CARTESIAN_POINT ( 'NONE',  ( 10.56230152254410903, 0.000000000000000000, -6.187499998771023080 ) ) ;
#9374=CYLINDRICAL_SURFACE ( 'NONE', #27078, 5.999999999999998224 ) ;
#9385=CARTESIAN_POINT ( 'NONE',  ( 16.56230152254411436, -7.209453229046475009, -9.928124999385525840 ) ) ;
#9387=CARTESIAN_POINT ( 'NONE',  ( 13.56230152254411436, -5.196152422706638241, -2.625000000000043965 ) ) ;
#9398=CARTESIAN_POINT ( 'NONE',  ( 16.56230152254410015, -7.209453229046475009, -4.078124999385484450 ) ) ;
#9405=CARTESIAN_POINT ( 'NONE',  ( 22.56230152254411792, 7.347880794884125653E-16, -5.175000000000040679 ) ) ;
#9417=EDGE_CURVE ( 'NONE', #6556, #19909, #1301, .T. ) ;
#9427=LINE ( 'NONE', #32539, #11419 ) ;
#9431=CARTESIAN_POINT ( 'NONE',  ( 22.80587116629410716, -3.604726614523235284, -0.8531249993855525293 ) ) ;
#9438=DIRECTION ( 'NONE',  ( 1.000000000000000000, 0.000000000000000000, 0.000000000000000000 ) ) ;
#9462=CARTESIAN_POINT ( 'NONE',  ( 22.80587116629410360, -3.604726614523235284, -6.253124999385533123 ) ) ;
#9469=CARTESIAN_POINT ( 'NONE',  ( 10.56230152254411259, -3.464101615137757051, -5.249999998770995546 ) ) ;
#9474=CARTESIAN_POINT ( 'NONE',  ( 22.80587116629412137, 7.646167579472024665E-16, -4.021874999385527616 ) ) ;
#9476=CARTESIAN_POINT ( 'NONE',  ( 10.56230152254410726, 0.000000000000000000, -7.087499998771007448 ) ) ;
#9505=CARTESIAN_POINT ( 'NONE',  ( 19.68408634441911431, 5.407089921784862696, -7.096874999385549998 ) ) ;
#9513=CARTESIAN_POINT ( 'NONE',  ( 22.56230152254225274, -3.464101615138824197, -9.599999998771053811 ) ) ;
#9525=CARTESIAN_POINT ( 'NONE',  ( 22.56230152254412147, 3.464101615137759271, -6.937500000000048850 ) ) ;
#9526=ORIENTED_EDGE ( 'NONE', *, *, #26140, .T. ) ;
#9532=CARTESIAN_POINT ( 'NONE',  ( 18.71316448956201839, -5.789678881962990076, -10.00000000000000355 ) ) ;
#9541=CARTESIAN_POINT ( 'NONE',  ( 10.31873187879411269, 3.604726614523240613, -4.284374999385515359 ) ) ;
#9552=CARTESIAN_POINT ( 'NONE',  ( 22.80587116629410360, -3.604726614523235284, -1.753124999385512028 ) ) ;
#9554=CARTESIAN_POINT ( 'NONE',  ( 8.562301522544109034, 9.797174393178823685E-16, -10.00000000000000000 ) ) ;
#9559=CARTESIAN_POINT ( 'NONE',  ( 13.56230152254410903, 5.196152422706636465, -0.5250000000000532019 ) ) ;
#9566=CARTESIAN_POINT ( 'NONE',  ( 13.56230152254410903, 5.196152422706636465, -0.07500000000004725109 ) ) ;
#9571=CARTESIAN_POINT ( 'NONE',  ( 13.56230152254411259, -5.196152422706632912, -0.7124999987710434191 ) ) ;
#9584=CARTESIAN_POINT ( 'NONE',  ( 19.68408634441910721, 5.407089921784857367, -5.690624999385579308 ) ) ;
#9593=CARTESIAN_POINT ( 'NONE',  ( 10.56230152254416765, -3.464101615137792134, -4.012500000000060574 ) ) ;
#9607=EDGE_CURVE ( 'NONE', #25759, #26216, #5607, .T. ) ;
#9609=DIRECTION ( 'NONE',  ( 1.000000000000000000, 0.000000000000000000, 0.000000000000000000 ) ) ;
#9619=CARTESIAN_POINT ( 'NONE',  ( 10.31873187879411091, 3.604726614523236616, -5.128124999385527794 ) ) ;
#9639=ORIENTED_EDGE ( 'NONE', *, *, #17982, .T. ) ;
#9647=EDGE_CURVE ( 'NONE', #6483, #31946, #5535, .T. ) ;
#9650=CARTESIAN_POINT ( 'NONE',  ( 13.44051670066911086, 5.407089921784856479, -5.165624999385554084 ) ) ;
#9656=CARTESIAN_POINT ( 'NONE',  ( 19.56230152254411081, 5.196152422706631135, -4.987499998771016685 ) ) ;
#9661=CARTESIAN_POINT ( 'NONE',  ( 10.31873187879411091, -3.604726614523244610, -5.109374999385544847 ) ) ;
#9674=CARTESIAN_POINT ( 'NONE',  ( 10.56230152254363652, -3.464101615137481716, -5.249999998771001763 ) ) ;
#9675=CARTESIAN_POINT ( 'NONE',  ( 10.56230152254410903, 0.000000000000000000, 10.00000000000000000 ) ) ;
#9676=CYLINDRICAL_SURFACE ( 'NONE', #31811, 5.999999999999998224 ) ;
#9678=DIRECTION ( 'NONE',  ( 0.000000000000000000, 0.000000000000000000, 1.000000000000000000 ) ) ;
#9681=VERTEX_POINT ( 'NONE', #12044 ) ;
#9690=CARTESIAN_POINT ( 'NONE',  ( 10.31873187879411091, 3.604726614523240613, -6.534374999385494043 ) ) ;
#9692=EDGE_LOOP ( 'NONE', ( #35454, #20087 ) ) ;
#9713=CARTESIAN_POINT ( 'NONE',  ( 19.56230152254412147, 5.196152422706637353, -7.350000000000022737 ) ) ;
#9717=DIRECTION ( 'NONE',  ( 0.000000000000000000, 0.000000000000000000, 1.000000000000000000 ) ) ;
#9724=CARTESIAN_POINT ( 'NONE',  ( 19.39205759080449809, -5.473655403650819373, -10.00000000000000000 ) ) ;
#9733=CARTESIAN_POINT ( 'NONE',  ( 16.56230152254411436, -7.209453229046482114, -3.234374999385536853 ) ) ;
#9749=CARTESIAN_POINT ( 'NONE',  ( 16.56230152254410726, 0.000000000000000000, -10.00000000000000000 ) ) ;
#9754=CARTESIAN_POINT ( 'NONE',  ( 16.56230152254411436, -6.928203230275514990, -0.7875000000000326184 ) ) ;
#9755=CARTESIAN_POINT ( 'NONE',  ( 10.56230152254411081, 0.000000000000000000, -5.287499998771011178 ) ) ;
#9769=CARTESIAN_POINT ( 'NONE',  ( 13.44051670066911797, -5.407089921784859143, -6.365624999385560479 ) ) ;
#9778=CYLINDRICAL_SURFACE ( 'NONE', #21556, 5.999999999999998224 ) ;
#9804=CARTESIAN_POINT ( 'NONE',  ( 22.80587116629410716, 3.604726614523238837, -5.278124999385515714 ) ) ;
#9810=CARTESIAN_POINT ( 'NONE',  ( 22.56230152254534715, -3.464101615137050505, -8.362500000000045119 ) ) ;
#9834=CARTESIAN_POINT ( 'NONE',  ( 16.56230152254410726, -7.209453229046475009, -8.578124999385506655 ) ) ;
#9841=CARTESIAN_POINT ( 'NONE',  ( 13.56230152254411436, -5.196152422706632912, -5.662499998771053811 ) ) ;
#9845=CARTESIAN_POINT ( 'NONE',  ( 22.80587116629411781, 3.604726614523243278, -4.434374999385503280 ) ) ;
#9846=CARTESIAN_POINT ( 'NONE',  ( 10.56230152254450338, 3.464101615137982204, -3.074999998770982845 ) ) ;
#9861=CARTESIAN_POINT ( 'NONE',  ( 16.56230152254411436, -7.209453229046475009, -0.4781249993855187230 ) ) ;
#9873=CARTESIAN_POINT ( 'NONE',  ( 19.68408634441911431, 5.407089921784862696, -6.196874999385537208 ) ) ;
#9893=CARTESIAN_POINT ( 'NONE',  ( 10.56230152254410548, 0.000000000000000000, -6.750000000000061284 ) ) ;
#9902=CARTESIAN_POINT ( 'NONE',  ( 21.58663455327491221, -3.463016004891044552, -9.999999999999998224 ) ) ;
#9905=CYLINDRICAL_SURFACE ( 'NONE', #10903, 5.999999999999998224 ) ;
#9910=CARTESIAN_POINT ( 'NONE',  ( 13.44051670066911086, -5.407089921784865361, -2.821874999385520777 ) ) ;
#9950=ORIENTED_EDGE ( 'NONE', *, *, #23070, .F. ) ;
#9953=CARTESIAN_POINT ( 'NONE',  ( 10.31873187879411269, 3.604726614523236616, -6.028124999385552130 ) ) ;
#9955=CARTESIAN_POINT ( 'NONE',  ( 16.56230152254411081, -6.928203230275506996, -2.474999998771027165 ) ) ;
#9960=EDGE_LOOP ( 'NONE', ( #24513, #3917, #5801, #30736 ) ) ;
#9968=CARTESIAN_POINT ( 'NONE',  ( 13.56230152254411792, -5.196152422706632912, -3.862499998771057541 ) ) ;
#9988=CARTESIAN_POINT ( 'NONE',  ( 19.68408634441910721, -5.407089921784855591, -4.940624999385550886 ) ) ;
#9990=DIRECTION ( 'NONE',  ( 0.000000000000000000, 0.000000000000000000, 1.000000000000000000 ) ) ;
#9995=CARTESIAN_POINT ( 'NONE',  ( 10.56230152254410726, 0.000000000000000000, -8.550000000000029132 ) ) ;
#10011=CARTESIAN_POINT ( 'NONE',  ( 16.56230152254411081, -6.928203230275506996, -9.224999998771027165 ) ) ;
#10019=CARTESIAN_POINT ( 'NONE',  ( 22.80587116629411071, -3.604726614523235284, -7.603124999385553195 ) ) ;
#10024=CARTESIAN_POINT ( 'NONE',  ( 16.56230152254410726, 6.928203230275506996, -8.099999998770989862 ) ) ;
#10028=CARTESIAN_POINT ( 'NONE',  ( 10.31873187879410736, 0.000000000000000000, -3.796874999385524418 ) ) ;
#10048=CARTESIAN_POINT ( 'NONE',  ( 22.80587116629410360, 7.646167579472015790E-16, -2.165624999385551419 ) ) ;
#10060=CARTESIAN_POINT ( 'NONE',  ( 19.68408634441911786, -5.407089921784861808, -4.996874999385530813 ) ) ;
#10081=VECTOR ( 'NONE', #16333, 1000.000000000000000 ) ;
#10085=CARTESIAN_POINT ( 'NONE',  ( 10.56230152254411259, -3.464101615137761048, -6.712500000000003020 ) ) ;
#10086=ORIENTED_EDGE ( 'NONE', *, *, #16832, .F. ) ;
#10094=CARTESIAN_POINT ( 'NONE',  ( 21.44299373557924682, -3.671490946209025719, -9.999999999999996447 ) ) ;
#10095=DIRECTION ( 'NONE',  ( 0.000000000000000000, 0.000000000000000000, 1.000000000000000000 ) ) ;
#10100=ADVANCED_FACE ( 'NONE', ( #18976 ), #2083, .F. ) ;
#10101=CARTESIAN_POINT ( 'NONE',  ( 19.68408634441911786, -5.407089921784861808, -4.996874999385530813 ) ) ;
#10112=EDGE_CURVE ( 'NONE', #20463, #29417, #2955, .T. ) ;
#10113=DIRECTION ( 'NONE',  ( 0.000000000000000000, 0.000000000000000000, 1.000000000000000000 ) ) ;
#10117=CARTESIAN_POINT ( 'NONE',  ( 22.56230152254503452, 3.464101615137219259, -1.874999998771022636 ) ) ;
#10118=CARTESIAN_POINT ( 'NONE',  ( 16.56230152254410726, 0.000000000000000000, -10.00000000000000000 ) ) ;
#10124=CARTESIAN_POINT ( 'NONE',  ( 22.46128102716605923, 1.096376214649937619, -10.00000000000000000 ) ) ;
#10140=EDGE_CURVE ( 'NONE', #20388, #12454, #35382, .T. ) ;
#10142=CARTESIAN_POINT ( 'NONE',  ( 13.44051670066911619, -5.407089921784859143, -7.265624999385544847 ) ) ;
#10157=CARTESIAN_POINT ( 'NONE',  ( 22.56230152254444832, 3.464101615137555878, -5.024999998771018106 ) ) ;
#10177=CARTESIAN_POINT ( 'NONE',  ( 13.44051670066911086, 5.407089921784856479, -4.265624999385542182 ) ) ;
#10179=EDGE_CURVE ( 'NONE', #35635, #34832, #23778, .T. ) ;
#10181=CARTESIAN_POINT ( 'NONE',  ( 22.80587116629412492, 3.604726614523243278, -9.834374999385516958 ) ) ;
#10186=CARTESIAN_POINT ( 'NONE',  ( 13.44051670066911264, -5.407089921784865361, -1.921874999385508875 ) ) ;
#10195=EDGE_CURVE ( 'NONE', #36001, #29181, #36822, .T. ) ;
#10199=VECTOR ( 'NONE', #31261, 1000.000000000000000 ) ;
#10200=ORIENTED_EDGE ( 'NONE', *, *, #30521, .F. ) ;
#10210=CARTESIAN_POINT ( 'NONE',  ( 13.44051670066911619, -5.407089921784859143, -7.715624999385550353 ) ) ;
#10216=CARTESIAN_POINT ( 'NONE',  ( 13.56230152254410548, 5.196152422706630247, -8.512499998770989507 ) ) ;
#10219=CARTESIAN_POINT ( 'NONE',  ( 19.68408634441911431, -5.407089921784861808, -5.896874999385542715 ) ) ;
#10224=CARTESIAN_POINT ( 'NONE',  ( 16.56230152254410726, 0.000000000000000000, -10.00000000000000000 ) ) ;
#10246=CARTESIAN_POINT ( 'NONE',  ( 22.80587116629412492, 3.604726614523243278, -6.234374999385519089 ) ) ;
#10250=CARTESIAN_POINT ( 'NONE',  ( 10.31873187879410736, -3.604726614523240613, -0.5531249993855127389 ) ) ;
#10258=CARTESIAN_POINT ( 'NONE',  ( 16.56230152254411436, 6.928203230275506996, -0.8999999987709939031 ) ) ;
#10265=DIRECTION ( 'NONE',  ( -0.000000000000000000, -0.000000000000000000, -1.000000000000000000 ) ) ;
#10267=CARTESIAN_POINT ( 'NONE',  ( 13.56230152254410726, 5.196152422706636465, -8.175000000000043343 ) ) ;
#10280=ORIENTED_EDGE ( 'NONE', *, *, #28353, .F. ) ;
#10283=CARTESIAN_POINT ( 'NONE',  ( 16.56230152254411436, 7.209453229046482114, -7.509374999385480365 ) ) ;
#10289=EDGE_LOOP ( 'NONE', ( #3035, #23545, #21906, #28663 ) ) ;
#10308=CARTESIAN_POINT ( 'NONE',  ( 10.56230152254410903, 3.464101615137757051, -1.837500000000043876 ) ) ;
#10316=CARTESIAN_POINT ( 'NONE',  ( 13.56230152254410370, 5.196152422706630247, -7.612499998771005139 ) ) ;
#10324=CARTESIAN_POINT ( 'NONE',  ( 13.56230152254411792, -5.196152422706638241, -7.125000000000075495 ) ) ;
#10328=CARTESIAN_POINT ( 'NONE',  ( 16.56230152254410726, -7.209453229046475009, -6.778124999385522820 ) ) ;
#10334=VERTEX_POINT ( 'NONE', #19266 ) ;
#10356=EDGE_CURVE ( 'NONE', #17848, #28808, #27394, .T. ) ;
#10365=CARTESIAN_POINT ( 'NONE',  ( 10.31873187879411269, 3.604726614523236616, -4.228124999385536320 ) ) ;
#10374=CARTESIAN_POINT ( 'NONE',  ( 19.68408634441912142, -5.407089921784861808, -1.396874999385538940 ) ) ;
#10395=CARTESIAN_POINT ( 'NONE',  ( 16.56230152254411081, -7.209453229046475009, -7.678124999385514293 ) ) ;
#10403=CARTESIAN_POINT ( 'NONE',  ( 19.56230152254411436, -5.196152422706629359, -9.187499998771025744 ) ) ;
#10407=CARTESIAN_POINT ( 'NONE',  ( 16.56230152254411436, 7.209453229046482114, -9.759374999385554972 ) ) ;
#10409=CARTESIAN_POINT ( 'NONE',  ( 22.80587116629411781, -3.604726614523238837, -5.859374999385517313 ) ) ;
#10435=CARTESIAN_POINT ( 'NONE',  ( 13.44051670066911441, -5.407089921784865361, -9.121874999385520155 ) ) ;
#10439=CARTESIAN_POINT ( 'NONE',  ( 10.31873187879410736, -3.604726614523240613, -1.453124999385536187 ) ) ;
#10445=CARTESIAN_POINT ( 'NONE',  ( 16.56230152254411081, 6.928203230275506996, -2.249999998771013310 ) ) ;
#10447=LINE ( 'NONE', #36592, #10081 ) ;
#10448=CARTESIAN_POINT ( 'NONE',  ( 22.56230152254502741, -3.464101615137234358, -8.812500000000046185 ) ) ;
#10451=VECTOR ( 'NONE', #1986, 1000.000000000000000 ) ;
#10452=CARTESIAN_POINT ( 'NONE',  ( 19.56230152254412502, -5.196152422706635576, -8.400000000000073186 ) ) ;
#10468=CARTESIAN_POINT ( 'NONE',  ( 19.68408634441912142, -5.407089921784861808, -7.246874999385532590 ) ) ;
#10490=CARTESIAN_POINT ( 'NONE',  ( 10.56230152254410548, 3.464101615137757051, -1.387500000000016165 ) ) ;
#10508=CARTESIAN_POINT ( 'NONE',  ( 10.31873187879411091, -3.604726614523240613, -9.553124999385522287 ) ) ;
#10525=VECTOR ( 'NONE', #33268, 1000.000000000000000 ) ;
#10539=EDGE_CURVE ( 'NONE', #19993, #28398, #30083, .T. ) ;
#10551=CARTESIAN_POINT ( 'NONE',  ( 22.80587116629410716, 7.646167579472015790E-16, -5.765624999385543958 ) ) ;
#10559=CARTESIAN_POINT ( 'NONE',  ( 19.68408634441911076, 5.407089921784862696, -1.246874999385527705 ) ) ;
#10573=ADVANCED_FACE ( 'NONE', ( #18548 ), #21758, .F. ) ;
#10581=CARTESIAN_POINT ( 'NONE',  ( 13.44051670066911619, -5.407089921784859143, -7.265624999385544847 ) ) ;
#10586=CARTESIAN_POINT ( 'NONE',  ( 10.56230152254410903, 0.000000000000000000, -7.987499998771019349 ) ) ;
#10590=CARTESIAN_POINT ( 'NONE',  ( 10.31873187879410736, -3.604726614523244610, -6.909374999385495819 ) ) ;
#10593=CARTESIAN_POINT ( 'NONE',  ( 22.56230152254395094, 3.464101615137851642, -6.037500000000023626 ) ) ;
#10597=ORIENTED_EDGE ( 'NONE', *, *, #25981, .T. ) ;
#10619=CARTESIAN_POINT ( 'NONE',  ( 13.44051670066911086, 5.407089921784862696, -8.371874999385548577 ) ) ;
#10623=CARTESIAN_POINT ( 'NONE',  ( 19.68408634441910721, -5.407089921784855591, -0.4406249993855471114 ) ) ;
#10629=CARTESIAN_POINT ( 'NONE',  ( 10.56230152254410903, 0.000000000000000000, -0.7874999987710074034 ) ) ;
#10637=CARTESIAN_POINT ( 'NONE',  ( 10.31873187879411091, 0.000000000000000000, -0.1406249993855246405 ) ) ;
#10654=CARTESIAN_POINT ( 'NONE',  ( 22.80587116629411781, -3.604726614523238837, -6.759374999385539873 ) ) ;
#10661=CARTESIAN_POINT ( 'NONE',  ( 13.44051670066911086, 5.407089921784862696, -1.621874999385541916 ) ) ;
#10678=CARTESIAN_POINT ( 'NONE',  ( 10.56230152254410903, 0.000000000000000000, -1.800000000000051559 ) ) ;
#10691=ORIENTED_EDGE ( 'NONE', *, *, #5436, .T. ) ;
#10697=CARTESIAN_POINT ( 'NONE',  ( 16.56230152254411081, -7.209453229046475009, -9.028124999385500615 ) ) ;
#10703=VERTEX_POINT ( 'NONE', #19107 ) ;
#10735=CARTESIAN_POINT ( 'NONE',  ( 13.44051670066911086, 5.407089921784856479, -7.415624999385555860 ) ) ;
#10744=CARTESIAN_POINT ( 'NONE',  ( 16.56230152254411436, 7.209453229046482114, -0.7593749993855121172 ) ) ;
#10746=ORIENTED_EDGE ( 'NONE', *, *, #30201, .F. ) ;
#10750=CARTESIAN_POINT ( 'NONE',  ( 10.31873187879411091, 3.604726614523236616, -2.428124999385521399 ) ) ;
#10767=CARTESIAN_POINT ( 'NONE',  ( 22.80587116629411071, 3.604726614523238837, -9.778124999385536142 ) ) ;
#10773=CARTESIAN_POINT ( 'NONE',  ( 16.56230152254411081, -6.928203230275506996, -9.674999998771022902 ) ) ;
#10776=CARTESIAN_POINT ( 'NONE',  ( 10.31873187879410736, 0.000000000000000000, -10.09687499938552513 ) ) ;
#10777=CARTESIAN_POINT ( 'NONE',  ( 16.56230152254411436, 7.209453229046482114, -7.059374999385483740 ) ) ;
#10784=DIRECTION ( 'NONE',  ( 1.000000000000000000, 0.000000000000000000, 0.000000000000000000 ) ) ;
#10785=CARTESIAN_POINT ( 'NONE',  ( 10.56230152254410903, 0.000000000000000000, -0.4500000000000614619 ) ) ;
#10786=ORIENTED_EDGE ( 'NONE', *, *, #15018, .T. ) ;
#10788=CIRCLE ( 'NONE', #17447, 8.000000000000000000 ) ;
#10809=CARTESIAN_POINT ( 'NONE',  ( 10.31873187879410381, -3.604726614523244610, -9.159374999385505589 ) ) ;
#10812=CARTESIAN_POINT ( 'NONE',  ( 16.56230152254411081, -7.209453229046475009, -2.278124999385533922 ) ) ;
#10819=CARTESIAN_POINT ( 'NONE',  ( 10.56230152254411081, 0.000000000000000000, -0.3374999987710014526 ) ) ;
#10827=CARTESIAN_POINT ( 'NONE',  ( 22.56230152254411436, 3.464101615137759271, -8.737500000000032685 ) ) ;
#10835=CARTESIAN_POINT ( 'NONE',  ( 10.56230152254411436, 3.464101615137752610, -6.674999998771008691 ) ) ;
#10840=EDGE_CURVE ( 'NONE', #8243, #205, #24257, .T. ) ;
#10843=CARTESIAN_POINT ( 'NONE',  ( 19.68408634441911431, 5.407089921784862696, -5.746874999385531702 ) ) ;
#10848=CARTESIAN_POINT ( 'NONE',  ( 13.44051670066910908, 5.407089921784862696, -2.071874999385547866 ) ) ;
#10854=CARTESIAN_POINT ( 'NONE',  ( 19.56230152254411792, 5.196152422706637353, -2.850000000000019185 ) ) ;
#10859=CYLINDRICAL_SURFACE ( 'NONE', #975, 5.999999999999998224 ) ;
#10867=CARTESIAN_POINT ( 'NONE',  ( 16.56230152254411436, -6.928203230275514990, -2.587500000000015454 ) ) ;
#10875=CARTESIAN_POINT ( 'NONE',  ( 22.56230152254410370, 0.000000000000000000, -10.00000000000000000 ) ) ;
#10885=CARTESIAN_POINT ( 'NONE',  ( 16.56230152254411081, 7.209453229046475009, -9.703124999385542182 ) ) ;
#10891=VECTOR ( 'NONE', #20532, 1000.000000000000000 ) ;
#10895=CARTESIAN_POINT ( 'NONE',  ( 10.56230152254410903, 0.000000000000000000, -4.500000000000031974 ) ) ;
#10896=CARTESIAN_POINT ( 'NONE',  ( 10.56230152254455490, -3.464101615138013734, -1.312500000000048850 ) ) ;
#10903=AXIS2_PLACEMENT_3D ( 'NONE', #23942, #35863, #990 ) ;
#10912=ORIENTED_EDGE ( 'NONE', *, *, #12928, .T. ) ;
#10921=CARTESIAN_POINT ( 'NONE',  ( 22.80587116629411071, -3.604726614523235284, -7.153124999385556571 ) ) ;
#10930=CARTESIAN_POINT ( 'NONE',  ( 22.56230152254411792, 7.347880794884125653E-16, -2.025000000000027001 ) ) ;
#10937=CARTESIAN_POINT ( 'NONE',  ( 10.31873187879411091, 0.000000000000000000, -2.390624999385526639 ) ) ;
#10959=CARTESIAN_POINT ( 'NONE',  ( 10.56230152254410903, 0.000000000000000000, -8.437499998771025744 ) ) ;
#10962=CARTESIAN_POINT ( 'NONE',  ( 13.44051670066910908, 5.407089921784862696, -9.721874999385510918 ) ) ;
#10963=CARTESIAN_POINT ( 'NONE',  ( 13.44051670066911441, -5.407089921784865361, -6.871874999385546801 ) ) ;
#10990=CARTESIAN_POINT ( 'NONE',  ( 14.85533981743163245, -6.020045154339302762, -9.999999999999998224 ) ) ;
#10993=CARTESIAN_POINT ( 'NONE',  ( 22.80587116629411071, 3.604726614523243278, -8.934374999385493510 ) ) ;
#10997=CARTESIAN_POINT ( 'NONE',  ( 13.44051670066911264, 5.407089921784856479, -3.815624999385564209 ) ) ;
#11004=CARTESIAN_POINT ( 'NONE',  ( 19.56230152254411792, -5.196152422706629359, -1.987499998771014020 ) ) ;
#11012=CARTESIAN_POINT ( 'NONE',  ( 19.68408634441910721, -5.407089921784855591, -0.4406249993855471114 ) ) ;
#11018=CARTESIAN_POINT ( 'NONE',  ( 16.56230152254411081, 6.928203230275506996, -2.249999998771013310 ) ) ;
#11029=CARTESIAN_POINT ( 'NONE',  ( 13.44051670066910908, 5.407089921784862696, -6.571874999385523886 ) ) ;
#11033=ORIENTED_EDGE ( 'NONE', *, *, #24687, .F. ) ;
#11034=CARTESIAN_POINT ( 'NONE',  ( 10.31873187879410736, -3.604726614523244610, -1.059374999385519933 ) ) ;
#11043=ORIENTED_EDGE ( 'NONE', *, *, #1288, .F. ) ;
#11052=CARTESIAN_POINT ( 'NONE',  ( 22.56230152254411792, 7.347880794884125653E-16, -2.475000000000060485 ) ) ;
#11055=VERTEX_POINT ( 'NONE', #35990 ) ;
#11072=CARTESIAN_POINT ( 'NONE',  ( 19.68408634441910721, -5.407089921784855591, -9.890624999385533300 ) ) ;
#11078=VERTEX_POINT ( 'NONE', #12873 ) ;
#11102=ORIENTED_EDGE ( 'NONE', *, *, #16190, .F. ) ;
#11106=CARTESIAN_POINT ( 'NONE',  ( 22.56230152254500965, -3.464101615137234358, -0.7124999999999952482 ) ) ;
#11109=CARTESIAN_POINT ( 'NONE',  ( 16.56230152254411081, -7.209453229046475009, -5.878124999385531346 ) ) ;
#11117=CARTESIAN_POINT ( 'NONE',  ( 19.68408634441910721, 5.407089921784862696, -2.596874999385518024 ) ) ;
#11124=CARTESIAN_POINT ( 'NONE',  ( 10.31873187879411091, 3.604726614523236616, -1.078124999385534410 ) ) ;
#11128=VECTOR ( 'NONE', #12791, 1000.000000000000000 ) ;
#11147=VECTOR ( 'NONE', #22284, 1000.000000000000000 ) ;
#11149=CARTESIAN_POINT ( 'NONE',  ( 10.56230152254410903, 0.000000000000000000, -9.787499998771043153 ) ) ;
#11151=DIRECTION ( 'NONE',  ( 1.000000000000000000, 0.000000000000000000, 0.000000000000000000 ) ) ;
#11154=CARTESIAN_POINT ( 'NONE',  ( 13.44051670066911264, -5.407089921784865361, -8.221874999385537564 ) ) ;
#11161=ORIENTED_EDGE ( 'NONE', *, *, #34486, .F. ) ;
#11167=CARTESIAN_POINT ( 'NONE',  ( 10.56230152254405574, 3.464101615137725521, -4.087500000000053646 ) ) ;
#11179=CARTESIAN_POINT ( 'NONE',  ( 22.80587116629412137, 7.646167579472024665E-16, -8.971874999385509142 ) ) ;
#11182=CARTESIAN_POINT ( 'NONE',  ( 19.68408634441910721, -5.407089921784855591, -3.140624999385555061 ) ) ;
#11187=CARTESIAN_POINT ( 'NONE',  ( 10.56230152254411436, -3.464101615137757051, -3.449999998771012599 ) ) ;
#11196=ADVANCED_FACE ( 'NONE', ( #8132 ), #37102, .F. ) ;
#11197=CARTESIAN_POINT ( 'NONE',  ( 19.68408634441911076, -5.407089921784855591, -1.340624999385559013 ) ) ;
#11214=CARTESIAN_POINT ( 'NONE',  ( 10.31873187879410736, -3.604726614523244610, -8.259374999385515892 ) ) ;
#11219=CARTESIAN_POINT ( 'NONE',  ( 22.80587116629411781, 7.646167579472024665E-16, -1.321874999385519445 ) ) ;
#11225=CARTESIAN_POINT ( 'NONE',  ( 10.56230152254410903, 3.464101615137752610, -0.3749999987710042615 ) ) ;
#11237=CARTESIAN_POINT ( 'NONE',  ( 16.56230152254411436, -6.928203230275514990, -5.737500000000049560 ) ) ;
#11239=EDGE_LOOP ( 'NONE', ( #3223, #33454, #26638, #2949 ) ) ;
#11260=CARTESIAN_POINT ( 'NONE',  ( 19.68408634441910721, -5.407089921784855591, -8.540624999385542537 ) ) ;
#11297=CARTESIAN_POINT ( 'NONE',  ( 16.56230152254411081, 7.209453229046475009, -7.453124999385500438 ) ) ;
#11310=CARTESIAN_POINT ( 'NONE',  ( 19.68408634441910721, -5.407089921784855591, -2.690624999385549110 ) ) ;
#11340=CARTESIAN_POINT ( 'NONE',  ( 10.31873187879411091, 3.604726614523240613, -8.784374999385505589 ) ) ;
#11343=CARTESIAN_POINT ( 'NONE',  ( 19.56230152254411081, -5.196152422706629359, -1.087499998771029874 ) ) ;
#11347=CYLINDRICAL_SURFACE ( 'NONE', #25872, 5.999999999999998224 ) ;
#11364=CARTESIAN_POINT ( 'NONE',  ( 10.56230152254410726, 0.000000000000000000, -3.150000000000041656 ) ) ;
#11370=CARTESIAN_POINT ( 'NONE',  ( 10.31873187879411091, 0.000000000000000000, -2.840624999385532590 ) ) ;
#11375=CARTESIAN_POINT ( 'NONE',  ( 10.56230152254411436, -3.464101615137757051, -3.899999998771008336 ) ) ;
#11402=CARTESIAN_POINT ( 'NONE',  ( 13.44051670066911264, -5.407089921784865361, -8.221874999385537564 ) ) ;
#11407=CARTESIAN_POINT ( 'NONE',  ( 19.68408634441912142, -5.407089921784861808, -1.846874999385544891 ) ) ;
#11418=VERTEX_POINT ( 'NONE', #20250 ) ;
#11419=VECTOR ( 'NONE', #17967, 1000.000000000000000 ) ;
#11426=CARTESIAN_POINT ( 'NONE',  ( 10.56230152254410903, -3.464101615137761048, -4.462500000000024336 ) ) ;
#11427=ORIENTED_EDGE ( 'NONE', *, *, #19120, .F. ) ;
#11430=CARTESIAN_POINT ( 'NONE',  ( 10.56230152254416588, 3.464101615137787693, -6.337500000000034106 ) ) ;
#11433=EDGE_CURVE ( 'NONE', #26085, #2436, #9427, .T. ) ;
#11444=CARTESIAN_POINT ( 'NONE',  ( 16.56230152254411436, -7.209453229046482114, -1.434374999385489735 ) ) ;
#11451=ORIENTED_EDGE ( 'NONE', *, *, #3669, .T. ) ;
#11467=CARTESIAN_POINT ( 'NONE',  ( 22.56230152254434529, -3.464101615137613610, -4.199999998771044574 ) ) ;
#11478=CARTESIAN_POINT ( 'NONE',  ( 22.80587116629411071, 7.646167579472015790E-16, -8.915624999385585170 ) ) ;
#11482=CARTESIAN_POINT ( 'NONE',  ( 14.54431717697174875, 5.695505633664034839, -9.999999999999998224 ) ) ;
#11492=CARTESIAN_POINT ( 'NONE',  ( 19.68408634441910365, 5.407089921784857367, -3.440624999385522020 ) ) ;
#11510=CARTESIAN_POINT ( 'NONE',  ( 19.68408634441910721, -5.407089921784855591, -9.890624999385533300 ) ) ;
#11522=CARTESIAN_POINT ( 'NONE',  ( 10.31873187879411091, 3.604726614523240613, -9.234374999385533300 ) ) ;
#11526=CARTESIAN_POINT ( 'NONE',  ( 10.56230152254410903, 0.000000000000000000, -1.237499998771041110 ) ) ;
#11542=VERTEX_POINT ( 'NONE', #11888 ) ;
#11545=CARTESIAN_POINT ( 'NONE',  ( 10.56230152254300947, -3.464101615137121115, -2.099999998771007181 ) ) ;
#11551=CARTESIAN_POINT ( 'NONE',  ( 22.80587116629410716, -3.604726614523235284, -2.203124999385539962 ) ) ;
#11555=DIRECTION ( 'NONE',  ( 1.000000000000000000, 0.000000000000000000, 0.000000000000000000 ) ) ;
#11557=CARTESIAN_POINT ( 'NONE',  ( 13.56230152254411259, -5.196152422706632912, -2.962499998771017662 ) ) ;
#11566=DIRECTION ( 'NONE',  ( 0.000000000000000000, 0.000000000000000000, 1.000000000000000000 ) ) ;
#11580=VERTEX_POINT ( 'NONE', #15113 ) ;
#11584=CARTESIAN_POINT ( 'NONE',  ( 22.80587116629412492, -3.604726614523238837, -7.659374999385500260 ) ) ;
#11588=CARTESIAN_POINT ( 'NONE',  ( 19.68408634441911786, -5.407089921784861808, -4.096874999385518912 ) ) ;
#11605=CARTESIAN_POINT ( 'NONE',  ( 22.56230152254411792, 7.347880794884125653E-16, -5.175000000000040679 ) ) ;
#11624=CARTESIAN_POINT ( 'NONE',  ( 22.80587116629411781, 7.646167579472024665E-16, -1.321874999385519445 ) ) ;
#11631=VERTEX_POINT ( 'NONE', #28758 ) ;
#11634=CARTESIAN_POINT ( 'NONE',  ( 16.56230152254411081, 6.928203230275506996, -6.299999998771006915 ) ) ;
#11656=CARTESIAN_POINT ( 'NONE',  ( 16.56230152254411081, 7.209453229046475009, -8.353124999385522997 ) ) ;
#11661=CARTESIAN_POINT ( 'NONE',  ( 10.36878992021261148, -0.004136371210273081730, -9.999999999999998224 ) ) ;
#11672=CARTESIAN_POINT ( 'NONE',  ( 10.31873187879410914, 0.000000000000000000, -5.540624999385540761 ) ) ;
#11699=( BOUNDED_CURVE ( )  B_SPLINE_CURVE ( 2, ( #35840, #9513, #1532, #4002, #21276, #18431, #15198 ),
 .UNSPECIFIED., .F., .F. ) 
 B_SPLINE_CURVE_WITH_KNOTS ( ( 3, 2, 2, 3 ),
 ( 0.8913043478260908037, 0.8985507246376851498, 0.9057971014492794959, 0.9130434782608737310 ),
 .UNSPECIFIED. ) 
 CURVE ( )  GEOMETRIC_REPRESENTATION_ITEM ( )  RATIONAL_B_SPLINE_CURVE ( ( 0.9999999999999281686, 0.8660254037845105390, 1.000000000000000000, 0.8660254037844387076, 1.000000000000000000, 0.8660254037843606589, 1.000000000000077938 ) ) 
 REPRESENTATION_ITEM ( '' )  );
#11705=CARTESIAN_POINT ( 'NONE',  ( 22.80587116629411781, -3.604726614523238837, -8.109374999385527971 ) ) ;
#11708=CARTESIAN_POINT ( 'NONE',  ( 13.56230152254411614, -5.196152422706632912, -1.162499998771021614 ) ) ;
#11728=EDGE_LOOP ( 'NONE', ( #25389, #12386, #17332, #36940 ) ) ;
#11739=CARTESIAN_POINT ( 'NONE',  ( 22.80587116629411071, -3.604726614523235284, -4.903124999385514826 ) ) ;
#11745=CARTESIAN_POINT ( 'NONE',  ( 19.56230152254411792, -5.196152422706629359, -3.337499998771031873 ) ) ;
#11752=CYLINDRICAL_SURFACE ( 'NONE', #33891, 5.999999999999998224 ) ;
#11774=CARTESIAN_POINT ( 'NONE',  ( 16.56230152254411436, -7.209453229046482114, -7.734374999385493332 ) ) ;
#11777=VERTEX_POINT ( 'NONE', #30077 ) ;
#11778=CARTESIAN_POINT ( 'NONE',  ( 19.68408634441910721, 5.407089921784862696, -4.396874999385541827 ) ) ;
#11794=CARTESIAN_POINT ( 'NONE',  ( 22.56230152254411436, 3.464101615137759271, -3.787500000000046718 ) ) ;
#11811=CARTESIAN_POINT ( 'NONE',  ( 22.80587116629412492, 3.604726614523243278, -1.284374999385501814 ) ) ;
#11832=CARTESIAN_POINT ( 'NONE',  ( 13.56230152254411614, -5.196152422706638241, -5.325000000000079226 ) ) ;
#11844=FACE_OUTER_BOUND ( 'NONE', #22783, .T. ) ;
#11845=CARTESIAN_POINT ( 'NONE',  ( 22.80587116629411071, 3.604726614523238837, -9.328124999385510208 ) ) ;
#11848=CARTESIAN_POINT ( 'NONE',  ( 12.03223749450566160, 4.087220715173740082, -9.999999999999998224 ) ) ;
#11858=CARTESIAN_POINT ( 'NONE',  ( 10.31873187879411091, 3.604726614523236616, -3.328124999385545291 ) ) ;
#11872=B_SPLINE_CURVE_WITH_KNOTS ( 'NONE', 3,
 ( #97, #12036, #8827, #35149, #23235, #9011, #9201, #11661, #17552, #20399, #20769, #23794, #34597, #20581, #20207, #11848, #14698, #32313, #26069, #11482, #34783, #28907 ),
 .UNSPECIFIED., .F., .F.,
 ( 4, 2, 2, 2, 2, 2, 2, 2, 2, 2, 4 ),
 ( 0.000000000000000000, 0.001510400339957781394, 0.002265600509936672741, 0.003020800679915564089, 0.004531201019873346350, 0.005286401189852237698, 0.006041601359831129912, 0.007552001699788915209, 0.009062402039746699639, 0.01057280237970448580, 0.01208320271966227023 ),
 .UNSPECIFIED. ) ;
#11881=CARTESIAN_POINT ( 'NONE',  ( 10.56230152254403443, 3.464101615137706425, -4.424999998771029119 ) ) ;
#11885=ORIENTED_EDGE ( 'NONE', *, *, #128, .T. ) ;
#11888=CARTESIAN_POINT ( 'NONE',  ( 22.56230152254412147, 7.347880794884125653E-16, -8.775000000000032330 ) ) ;
#11891=CARTESIAN_POINT ( 'NONE',  ( 19.68408634441912142, -5.407089921784861808, -8.146874999385516958 ) ) ;
#11893=CARTESIAN_POINT ( 'NONE',  ( 22.80587116629411071, -3.604726614523235284, -1.303124999385484095 ) ) ;
#11910=ADVANCED_FACE ( 'NONE', ( #31017 ), #5403, .F. ) ;
#11913=EDGE_LOOP ( 'NONE', ( #17620, #33273, #10086, #35719 ) ) ;
#11923=CARTESIAN_POINT ( 'NONE',  ( 10.31873187879411091, 0.000000000000000000, -4.640624999385528859 ) ) ;
#11924=( BOUNDED_SURFACE ( )  B_SPLINE_SURFACE ( 1, 2, ( 
 ( #6916, #36081, #9566, #33062, #12595, #35704, #18487, #26995, #32679, #7107, #18676, #4244, #27369, #24531, #1399, #7287, #6722, #18860, #29836, #12215, #23787, #9754, #35326, #3872, #15445, #24160, #13342, #25084, #8219, #24899, #19419, #36450, #28298, #33430, #27746, #1775, #2144, #10490, #25273, #22069, #33620, #7471, #5173, #16381, #16196, #22628, #16750, #36825, #10678, #10308, #1958, #4803, #2336, #25457, #19049, #30601, #22257, #28114, #19605, #13724, #13907, #22440, #7661, #19238, #36639, #30780, #11052, #4618, #16568, #10867, #37009, #8030, #21879, #13529, #27927, #33809, #7846, #30968, #4985, #24712, #33987, #31153, #34175, #19794, #31330, #5358, #16936, #1588, #13157, #36264, #31514, #8403, #25826, #23180, #3073, #29220, #231, #34913, #19971, #415, #25640, #11794, #8958, #14455, #31885, #5538, #5915, #22809, #2699, #26011, #35097, #14275, #8771, #37374, #17683, #34358, #17125, #28662, #29029, #11426, #14643, #22993, #34543, #8582, #32071, #5726, #20152, #11980, #6099, #26193, #40, #37194, #28849, #31700, #3263, #14835, #17308, #2883, #11605, #17494, #20529, #23363, #26380, #23553, #34727, #20343, #9146, #20713, #32256, #6299, #28479, #2520, #14088, #11237, #598, #29794, #3641, #12362, #29605, #26569, #18062, #3448, #15589, #6677, #4016, #23932, #12167, #26760, #15405, #35279, #791, #15211, #20906, #9338, #35474, #29985, #6490, #15781, #32446, #10085, #9893, #3826, #23741, #27142, #24494, #9525, #26949, #979, #21097, #32637, #24121, #6868, #12555, #18250, #35664, #21477, #9713, #21288, #1169, #24309, #36041, #18636, #7067, #17871, #18443, #30176, #15019, #32823, #12741, #35852, #33016, #4204, #27331, #1361, #12932, #21655, #33208, #29416, #10267, #30926, #13685, #16338, #15969, #7619, #10452, #22399, #31112, #24672, #13118, #27887, #33767, #25233, #7807, #10827, #28072, #7435, #4580, #4764, #30562, #16713, #36225, #22216, #19383, #7989, #36782, #27521, #19195, #16156, #1733, #19004, #1546, #27705, #30366, #4943, #33581, #16525, #13302, #21842, #24860, #1917, #33395, #36408, #22028, #30743, #13485, #25041, #2106, #36597, #5132 ),
 ( #10637, #33948, #19563, #28260, #2292, #13867, #25416, #36969, #11012, #22586, #7248, #18822, #4389, #3555, #15308, #35381, #23842, #34131, #23652, #9431, #19754, #5498, #14932, #23461, #29324, #21009, #37155, #17971, #35015, #20629, #3362, #11893, #11197, #20817, #15117, #26479, #9244, #32543, #6398, #26668, #25600, #6585, #31293, #29514, #698, #32172, #510, #22770, #12078, #28436, #8364, #6209, #3735, #19934, #35195, #31474, #18160, #2477, #34318, #17081, #32359, #28620, #12270, #2657, #14234, #14050, #29701, #9058, #26292, #26860, #890, #12461, #8180, #5321, #328, #16897, #17781, #27421, #7344, #21569, #21753, #18917, #4299, #36136, #30274, #18346, #3924, #1455, #35759, #15878, #30082, #4116, #21940, #29894, #36318, #13028, #15498, #27053, #33114, #30468, #24584, #15689, #1079, #35575, #27240, #33485, #27614, #7159, #18732, #10365, #10177, #12649, #7530, #30654, #1263, #12834, #33304, #27802, #4489, #19103, #16066, #13217, #1645, #24401, #21196, #24766, #35949, #4669, #9988, #32922, #16252, #1829, #24030, #9619, #32734, #24214, #6771, #9804, #21382, #6974, #18543, #4858, #13960, #5232, #22125, #31568, #8453, #25509, #2198, #5590, #10551, #37062, #30834, #11109, #13778, #22496, #25326, #22685, #28718, #17177, #31387, #34229, #19295, #16989, #7902, #34043, #13399, #36875, #36695, #22865, #16437, #2386, #28529, #24948, #2572, #8089, #34415, #37248, #8272, #20022, #16626, #7713, #36506, #27984, #19475, #14142, #2014, #10921, #13591, #25696, #33673, #19845, #5407, #25141, #10735, #11297, #22308, #19663, #33860, #31204, #31022, #5044, #28168, #16807, #28349, #20396, #6158, #6539, #32122, #15070, #3312, #29466, #12033, #3127, #37429, #26431, #29085, #34965, #31937, #11656, #23601, #14884, #17732, #20960, #29273, #2940, #9008, #465, #28904, #6351, #23049, #31753, #35146, #9198, #11478, #32492, #35330, #20766, #14694, #18112, #34593, #32310, #20204, #17921, #26244, #11845, #279, #3501, #2755, #14327, #26620, #650, #8636, #12220, #34780, #23415, #25881, #20578, #26066, #23791, #5783, #9385, #17363, #14510, #94, #23232, #8823, #5969, #17549 ) ),
 .UNSPECIFIED., .F., .F., .F. ) 
 B_SPLINE_SURFACE_WITH_KNOTS ( ( 2, 2 ),
 ( 3, 2, 2, 2, 2, 2, 2, 2, 2, 2, 2, 2, 2, 2, 2, 2, 2, 2, 2, 2, 2, 2, 2, 2, 2, 2, 2, 2, 2, 2, 2, 2, 2, 2, 2, 2, 2, 2, 2, 2, 2, 2, 2, 2, 2, 2, 2, 2, 2, 2, 2, 2, 2, 2, 2, 2, 2, 2, 2, 2, 2, 2, 2, 2, 2, 2, 2, 2, 2, 2, 2, 2, 2, 2, 2, 2, 2, 2, 2, 2, 2, 2, 2, 2, 2, 2, 2, 2, 2, 2, 2, 2, 2, 2, 2, 2, 2, 2, 2, 2, 2, 2, 2, 2, 2, 2, 2, 2, 2, 2, 2, 2, 2, 2, 2, 2, 2, 2, 2, 2, 2, 2, 2, 2, 2, 2, 2, 2, 2, 2, 2, 2, 2, 2, 3 ),
 ( 0.000000000000000000, 1.000000000000000000 ),
 ( 0.000000000000000000, 0.007246376811594202987, 0.01449275362318840597, 0.02173913043478260809, 0.02898550724637681195, 0.03623188405797101580, 0.04347826086956521618, 0.05072463768115942351, 0.05797101449275362389, 0.06521739130434782428, 0.07246376811594203160, 0.07971014492753622505, 0.08695652173913043237, 0.09420289855072463969, 0.1014492753623188470, 0.1086956521739130405, 0.1159420289855072478, 0.1231884057971014551, 0.1304347826086956486, 0.1376811594202898559, 0.1449275362318840632, 0.1521739130434782705, 0.1594202898550724501, 0.1666666666666666574, 0.1739130434782608647, 0.1811594202898550721, 0.1884057971014492794, 0.1956521739130434867, 0.2028985507246376940, 0.2101449275362318736, 0.2173913043478260809, 0.2246376811594202882, 0.2318840579710144956, 0.2391304347826087029, 0.2463768115942029102, 0.2536231884057971175, 0.2608695652173912971, 0.2681159420289855322, 0.2753623188405797118, 0.2826086956521738913, 0.2898550724637681264, 0.2971014492753623060, 0.3043478260869565410, 0.3115942028985507206, 0.3188405797101449002, 0.3260869565217391353, 0.3333333333333333148, 0.3405797101449275499, 0.3478260869565217295, 0.3550724637681159646, 0.3623188405797101441, 0.3695652173913043237, 0.3768115942028985588, 0.3840579710144927383, 0.3913043478260869734, 0.3985507246376811530, 0.4057971014492753881, 0.4130434782608695676, 0.4202898550724637472, 0.4275362318840579823, 0.4347826086956521618, 0.4420289855072463969, 0.4492753623188405765, 0.4565217391304347561, 0.4637681159420289911, 0.4710144927536231707, 0.4782608695652174058, 0.4855072463768115854, 0.4927536231884058204, 0.5000000000000000000, 0.5072463768115942351, 0.5144927536231883591, 0.5217391304347825942, 0.5289855072463768293, 0.5362318840579710644, 0.5434782608695651884, 0.5507246376811594235, 0.5579710144927536586, 0.5652173913043477826, 0.5724637681159420177, 0.5797101449275362528, 0.5869565217391304879, 0.5942028985507246119, 0.6014492753623188470, 0.6086956521739130821, 0.6159420289855072062, 0.6231884057971014412, 0.6304347826086956763, 0.6376811594202898004, 0.6449275362318840354, 0.6521739130434782705, 0.6594202898550725056, 0.6666666666666666297, 0.6739130434782608647, 0.6811594202898550998, 0.6884057971014492239, 0.6956521739130434590, 0.7028985507246376940, 0.7101449275362319291, 0.7173913043478260532, 0.7246376811594202882, 0.7318840579710145233, 0.7391304347826086474, 0.7463768115942028825, 0.7536231884057971175, 0.7608695652173913526, 0.7681159420289854767, 0.7753623188405797118, 0.7826086956521739468, 0.7898550724637680709, 0.7971014492753623060, 0.8043478260869565410, 0.8115942028985507761, 0.8188405797101449002, 0.8260869565217391353, 0.8333333333333333703, 0.8405797101449274944, 0.8478260869565217295, 0.8550724637681159646, 0.8623188405797101996, 0.8695652173913043237, 0.8768115942028985588, 0.8840579710144927938, 0.8913043478260869179, 0.8985507246376811530, 0.9057971014492753881, 0.9130434782608695121, 0.9202898550724637472, 0.9275362318840579823, 0.9347826086956522174, 0.9420289855072463414, 0.9492753623188405765, 0.9565217391304348116, 0.9637681159420289356, 0.9662082948456578446 ),
 .UNSPECIFIED. ) 
 GEOMETRIC_REPRESENTATION_ITEM ( )  RATIONAL_B_SPLINE_SURFACE ( (
 ( 1.000000000000000000, 0.8660254037844387076, 1.000000000000000000, 0.8660254037844387076, 1.000000000000000000, 0.8660254037844387076, 1.000000000000000000, 0.8660254037844387076, 1.000000000000000000, 0.8660254037844387076, 1.000000000000000000, 0.8660254037844387076, 1.000000000000000000, 0.8660254037844387076, 1.000000000000000000, 0.8660254037844387076, 1.000000000000000000, 0.8660254037844387076, 1.000000000000000000, 0.8660254037844387076, 1.000000000000000000, 0.8660254037844387076, 1.000000000000000000, 0.8660254037844387076, 1.000000000000000000, 0.8660254037844387076, 1.000000000000000000, 0.8660254037844387076, 1.000000000000000000, 0.8660254037844387076, 1.000000000000000000, 0.8660254037844387076, 1.000000000000000000, 0.8660254037844387076, 1.000000000000000000, 0.8660254037844387076, 1.000000000000000000, 0.8660254037844387076, 1.000000000000000000, 0.8660254037844387076, 1.000000000000000000, 0.8660254037844387076, 1.000000000000000000, 0.8660254037844387076, 1.000000000000000000, 0.8660254037844387076, 1.000000000000000000, 0.8660254037844387076, 1.000000000000000000, 0.8660254037844387076, 1.000000000000000000, 0.8660254037844387076, 1.000000000000000000, 0.8660254037844387076, 1.000000000000000000, 0.8660254037844387076, 1.000000000000000000, 0.8660254037844387076, 1.000000000000000000, 0.8660254037844387076, 1.000000000000000000, 0.8660254037844387076, 1.000000000000000000, 0.8660254037844387076, 1.000000000000000000, 0.8660254037844387076, 1.000000000000000000, 0.8660254037844387076, 1.000000000000000000, 0.8660254037844387076, 1.000000000000000000, 0.8660254037844387076, 1.000000000000000000, 0.8660254037844387076, 1.000000000000000000, 0.8660254037844387076, 1.000000000000000000, 0.8660254037844387076, 1.000000000000000000, 0.8660254037844387076, 1.000000000000000000, 0.8660254037844387076, 1.000000000000000000, 0.8660254037844387076, 1.000000000000000000, 0.8660254037844387076, 1.000000000000000000, 0.8660254037844387076, 1.000000000000000000, 0.8660254037844387076, 1.000000000000000000, 0.8660254037844387076, 1.000000000000000000, 0.8660254037844387076, 1.000000000000000000, 0.8660254037844387076, 1.000000000000000000, 0.8660254037844387076, 1.000000000000000000, 0.8660254037844387076, 1.000000000000000000, 0.8660254037844387076, 1.000000000000000000, 0.8660254037844387076, 1.000000000000000000, 0.8660254037844387076, 1.000000000000000000, 0.8660254037844387076, 1.000000000000000000, 0.8660254037844387076, 1.000000000000000000, 0.8660254037844387076, 1.000000000000000000, 0.8660254037844387076, 1.000000000000000000, 0.8660254037844387076, 1.000000000000000000, 0.8660254037844387076, 1.000000000000000000, 0.8660254037844387076, 1.000000000000000000, 0.8660254037844387076, 1.000000000000000000, 0.8660254037844387076, 1.000000000000000000, 0.8660254037844387076, 1.000000000000000000, 0.8660254037844387076, 1.000000000000000000, 0.8660254037844387076, 1.000000000000000000, 0.8660254037844387076, 1.000000000000000000, 0.8660254037844387076, 1.000000000000000000, 0.8660254037844387076, 1.000000000000000000, 0.8660254037844387076, 1.000000000000000000, 0.8660254037844387076, 1.000000000000000000, 0.8660254037844387076, 1.000000000000000000, 0.8660254037844387076, 1.000000000000000000, 0.8660254037844387076, 1.000000000000000000, 0.8660254037844387076, 1.000000000000000000, 0.8660254037844387076, 1.000000000000000000, 0.8660254037844387076, 1.000000000000000000, 0.8660254037844387076, 1.000000000000000000, 0.8660254037844387076, 1.000000000000000000, 0.8660254037844387076, 1.000000000000000000, 0.8660254037844387076, 1.000000000000000000, 0.8660254037844387076, 1.000000000000000000, 0.8660254037844387076, 1.000000000000000000, 0.8660254037844387076, 1.000000000000000000, 0.8660254037844387076, 1.000000000000000000, 0.8660254037844387076, 1.000000000000000000, 0.8660254037844387076, 1.000000000000000000, 0.8660254037844387076, 1.000000000000000000, 0.8660254037844387076, 1.000000000000000000, 0.8660254037844387076, 1.000000000000000000, 0.8660254037844387076, 1.000000000000000000, 0.8660254037844387076, 1.000000000000000000, 0.8660254037844387076, 1.000000000000000000, 0.8660254037844387076, 1.000000000000000000, 0.8660254037844387076, 1.000000000000000000, 0.8660254037844387076, 1.000000000000000000, 0.8660254037844387076, 1.000000000000000000, 0.8660254037844387076, 1.000000000000000000, 0.8660254037844387076, 1.000000000000000000, 0.8660254037844387076, 1.000000000000000000, 0.8660254037844387076, 1.000000000000000000, 0.8660254037844387076, 1.000000000000000000, 0.8660254037844387076, 1.000000000000000000, 0.8660254037844387076, 1.000000000000000000, 0.8660254037844387076, 1.000000000000000000, 0.8660254037844387076, 1.000000000000000000, 0.8660254037844387076, 1.000000000000000000, 0.8660254037844387076, 1.000000000000000000, 0.8660254037844387076, 1.000000000000000000, 0.8660254037844387076, 1.000000000000000000, 0.8660254037844387076, 1.000000000000000000, 0.8660254037844387076, 1.000000000000000000, 0.8660254037844387076, 1.000000000000000000, 0.8660254037844387076, 1.000000000000000000, 0.8660254037844387076, 1.000000000000000000, 0.8660254037844387076, 1.000000000000000000, 0.8660254037844387076, 1.000000000000000000, 0.8660254037844387076, 1.000000000000000000, 0.8660254037844387076, 1.000000000000000000, 0.8660254037844387076, 1.000000000000000000, 0.8660254037844387076, 1.000000000000000000, 0.8660254037844387076, 1.000000000000000000, 0.8660254037844387076, 1.000000000000000000, 0.8660254037844387076, 1.000000000000000000, 0.8660254037844387076, 1.000000000000000000, 0.8660254037844387076, 1.000000000000000000, 0.8660254037844387076, 1.000000000000000000, 0.8660254037844387076, 1.000000000000000000, 0.8660254037844387076, 1.000000000000000000, 0.8660254037844387076, 1.000000000000000000, 0.8660254037844387076, 1.000000000000000000, 0.8660254037844387076, 1.000000000000000000, 0.8660254037844387076, 1.000000000000000000, 0.8660254037844387076, 1.000000000000000000, 0.9548847663035771038, 0.9401541632606846832),
 ( 1.000000000000000000, 0.8660254037844387076, 1.000000000000000000, 0.8660254037844387076, 1.000000000000000000, 0.8660254037844387076, 1.000000000000000000, 0.8660254037844387076, 1.000000000000000000, 0.8660254037844387076, 1.000000000000000000, 0.8660254037844387076, 1.000000000000000000, 0.8660254037844387076, 1.000000000000000000, 0.8660254037844387076, 1.000000000000000000, 0.8660254037844387076, 1.000000000000000000, 0.8660254037844387076, 1.000000000000000000, 0.8660254037844387076, 1.000000000000000000, 0.8660254037844387076, 1.000000000000000000, 0.8660254037844387076, 1.000000000000000000, 0.8660254037844387076, 1.000000000000000000, 0.8660254037844387076, 1.000000000000000000, 0.8660254037844387076, 1.000000000000000000, 0.8660254037844387076, 1.000000000000000000, 0.8660254037844387076, 1.000000000000000000, 0.8660254037844387076, 1.000000000000000000, 0.8660254037844387076, 1.000000000000000000, 0.8660254037844387076, 1.000000000000000000, 0.8660254037844387076, 1.000000000000000000, 0.8660254037844387076, 1.000000000000000000, 0.8660254037844387076, 1.000000000000000000, 0.8660254037844387076, 1.000000000000000000, 0.8660254037844387076, 1.000000000000000000, 0.8660254037844387076, 1.000000000000000000, 0.8660254037844387076, 1.000000000000000000, 0.8660254037844387076, 1.000000000000000000, 0.8660254037844387076, 1.000000000000000000, 0.8660254037844387076, 1.000000000000000000, 0.8660254037844387076, 1.000000000000000000, 0.8660254037844387076, 1.000000000000000000, 0.8660254037844387076, 1.000000000000000000, 0.8660254037844387076, 1.000000000000000000, 0.8660254037844387076, 1.000000000000000000, 0.8660254037844387076, 1.000000000000000000, 0.8660254037844387076, 1.000000000000000000, 0.8660254037844387076, 1.000000000000000000, 0.8660254037844387076, 1.000000000000000000, 0.8660254037844387076, 1.000000000000000000, 0.8660254037844387076, 1.000000000000000000, 0.8660254037844387076, 1.000000000000000000, 0.8660254037844387076, 1.000000000000000000, 0.8660254037844387076, 1.000000000000000000, 0.8660254037844387076, 1.000000000000000000, 0.8660254037844387076, 1.000000000000000000, 0.8660254037844387076, 1.000000000000000000, 0.8660254037844387076, 1.000000000000000000, 0.8660254037844387076, 1.000000000000000000, 0.8660254037844387076, 1.000000000000000000, 0.8660254037844387076, 1.000000000000000000, 0.8660254037844387076, 1.000000000000000000, 0.8660254037844387076, 1.000000000000000000, 0.8660254037844387076, 1.000000000000000000, 0.8660254037844387076, 1.000000000000000000, 0.8660254037844387076, 1.000000000000000000, 0.8660254037844387076, 1.000000000000000000, 0.8660254037844387076, 1.000000000000000000, 0.8660254037844387076, 1.000000000000000000, 0.8660254037844387076, 1.000000000000000000, 0.8660254037844387076, 1.000000000000000000, 0.8660254037844387076, 1.000000000000000000, 0.8660254037844387076, 1.000000000000000000, 0.8660254037844387076, 1.000000000000000000, 0.8660254037844387076, 1.000000000000000000, 0.8660254037844387076, 1.000000000000000000, 0.8660254037844387076, 1.000000000000000000, 0.8660254037844387076, 1.000000000000000000, 0.8660254037844387076, 1.000000000000000000, 0.8660254037844387076, 1.000000000000000000, 0.8660254037844387076, 1.000000000000000000, 0.8660254037844387076, 1.000000000000000000, 0.8660254037844387076, 1.000000000000000000, 0.8660254037844387076, 1.000000000000000000, 0.8660254037844387076, 1.000000000000000000, 0.8660254037844387076, 1.000000000000000000, 0.8660254037844387076, 1.000000000000000000, 0.8660254037844387076, 1.000000000000000000, 0.8660254037844387076, 1.000000000000000000, 0.8660254037844387076, 1.000000000000000000, 0.8660254037844387076, 1.000000000000000000, 0.8660254037844387076, 1.000000000000000000, 0.8660254037844387076, 1.000000000000000000, 0.8660254037844387076, 1.000000000000000000, 0.8660254037844387076, 1.000000000000000000, 0.8660254037844387076, 1.000000000000000000, 0.8660254037844387076, 1.000000000000000000, 0.8660254037844387076, 1.000000000000000000, 0.8660254037844387076, 1.000000000000000000, 0.8660254037844387076, 1.000000000000000000, 0.8660254037844387076, 1.000000000000000000, 0.8660254037844387076, 1.000000000000000000, 0.8660254037844387076, 1.000000000000000000, 0.8660254037844387076, 1.000000000000000000, 0.8660254037844387076, 1.000000000000000000, 0.8660254037844387076, 1.000000000000000000, 0.8660254037844387076, 1.000000000000000000, 0.8660254037844387076, 1.000000000000000000, 0.8660254037844387076, 1.000000000000000000, 0.8660254037844387076, 1.000000000000000000, 0.8660254037844387076, 1.000000000000000000, 0.8660254037844387076, 1.000000000000000000, 0.8660254037844387076, 1.000000000000000000, 0.8660254037844387076, 1.000000000000000000, 0.8660254037844387076, 1.000000000000000000, 0.8660254037844387076, 1.000000000000000000, 0.8660254037844387076, 1.000000000000000000, 0.8660254037844387076, 1.000000000000000000, 0.8660254037844387076, 1.000000000000000000, 0.8660254037844387076, 1.000000000000000000, 0.8660254037844387076, 1.000000000000000000, 0.8660254037844387076, 1.000000000000000000, 0.8660254037844387076, 1.000000000000000000, 0.8660254037844387076, 1.000000000000000000, 0.8660254037844387076, 1.000000000000000000, 0.8660254037844387076, 1.000000000000000000, 0.8660254037844387076, 1.000000000000000000, 0.8660254037844387076, 1.000000000000000000, 0.8660254037844387076, 1.000000000000000000, 0.8660254037844387076, 1.000000000000000000, 0.8660254037844387076, 1.000000000000000000, 0.8660254037844387076, 1.000000000000000000, 0.8660254037844387076, 1.000000000000000000, 0.8660254037844387076, 1.000000000000000000, 0.8660254037844387076, 1.000000000000000000, 0.8660254037844387076, 1.000000000000000000, 0.8660254037844387076, 1.000000000000000000, 0.8660254037844387076, 1.000000000000000000, 0.8660254037844387076, 1.000000000000000000, 0.8660254037844387076, 1.000000000000000000, 0.8660254037844387076, 1.000000000000000000, 0.8660254037844387076, 1.000000000000000000, 0.9548847663035771038, 0.9401541632606846832) ) ) 
 REPRESENTATION_ITEM ( '' )  SURFACE ( )  );
#11928=CARTESIAN_POINT ( 'NONE',  ( 13.56230152254410370, 5.196152422706630247, -7.162499998770998744 ) ) ;
#11935=CARTESIAN_POINT ( 'NONE',  ( 10.56230152254410726, 0.000000000000000000, -8.100000000000024514 ) ) ;
#11948=EDGE_CURVE ( 'NONE', #25619, #19865, #17251, .T. ) ;
#11952=CARTESIAN_POINT ( 'NONE',  ( 10.31873187879410914, 0.000000000000000000, -0.5906249993855583469 ) ) ;
#11962=ORIENTED_EDGE ( 'NONE', *, *, #12882, .F. ) ;
#11963=CARTESIAN_POINT ( 'NONE',  ( 22.80587116629412137, 7.646167579472024665E-16, -4.471874999385533123 ) ) ;
#11980=CARTESIAN_POINT ( 'NONE',  ( 22.56230152254412857, -3.464101615137755275, -4.762500000000064126 ) ) ;
#11988=CARTESIAN_POINT ( 'NONE',  ( 22.56230152254410370, 7.347880794884117764E-16, -3.712499998771018106 ) ) ;
#11989=CYLINDRICAL_SURFACE ( 'NONE', #33984, 5.999999999999998224 ) ;
#11999=CARTESIAN_POINT ( 'NONE',  ( 16.56230152254411436, 7.209453229046482114, -1.659374999385503591 ) ) ;
#12007=CARTESIAN_POINT ( 'NONE',  ( 22.56230152254394383, 3.464101615137847645, -6.374999998770999099 ) ) ;
#12032=DIRECTION ( 'NONE',  ( 1.000000000000000000, 0.000000000000000000, 0.000000000000000000 ) ) ;
#12033=CARTESIAN_POINT ( 'NONE',  ( 19.68408634441910721, -5.407089921784855591, -8.090624999385564564 ) ) ;
#12036=CARTESIAN_POINT ( 'NONE',  ( 11.02886091400724133, -2.913158743114809823, -10.00000000000000178 ) ) ;
#12044=CARTESIAN_POINT ( 'NONE',  ( 10.56230152254411081, 0.000000000000000000, -7.537499998771012955 ) ) ;
#12045=CARTESIAN_POINT ( 'NONE',  ( 16.56230152254411436, 7.209453229046475009, -4.753124999385526017 ) ) ;
#12078=CARTESIAN_POINT ( 'NONE',  ( 10.31873187879411091, 0.000000000000000000, -1.940624999385548444 ) ) ;
#12083=CARTESIAN_POINT ( 'NONE',  ( 10.56230152254410903, 0.000000000000000000, -4.950000000000037481 ) ) ;
#12107=CARTESIAN_POINT ( 'NONE',  ( 22.80587116629410716, 7.646167579472015790E-16, -5.315624999385537564 ) ) ;
#12113=CARTESIAN_POINT ( 'NONE',  ( 10.56230152254411614, -3.464101615137757051, -5.699999998771023257 ) ) ;
#12118=CARTESIAN_POINT ( 'NONE',  ( 13.44051670066910908, 5.407089921784862696, -4.771874999385556038 ) ) ;
#12130=CARTESIAN_POINT ( 'NONE',  ( 10.56230152254410903, 0.000000000000000000, -4.950000000000037481 ) ) ;
#12132=CARTESIAN_POINT ( 'NONE',  ( 10.56230152254410903, 0.000000000000000000, -5.737499998771017573 ) ) ;
#12133=LINE ( 'NONE', #6828, #16241 ) ;
#12135=CARTESIAN_POINT ( 'NONE',  ( 22.80587116629410716, 7.646167579472015790E-16, -0.8156249993855335667 ) ) ;
#12147=CARTESIAN_POINT ( 'NONE',  ( 19.68408634441912142, -5.407089921784861808, -3.196874999385534988 ) ) ;
#12167=CARTESIAN_POINT ( 'NONE',  ( 13.56230152254411792, -5.196152422706638241, -6.225000000000063594 ) ) ;
#12175=CARTESIAN_POINT ( 'NONE',  ( 22.53918047650689616, -0.9001358824703226125, -10.00000000000000355 ) ) ;
#12186=CARTESIAN_POINT ( 'NONE',  ( 22.80587116629412492, 3.604726614523243278, -3.534374999385544669 ) ) ;
#12194=CYLINDRICAL_SURFACE ( 'NONE', #7612, 5.999999999999998224 ) ;
#12208=DIRECTION ( 'NONE',  ( 0.000000000000000000, 0.000000000000000000, 1.000000000000000000 ) ) ;
#12215=CARTESIAN_POINT ( 'NONE',  ( 22.56230152254411436, -3.464101615137755275, -0.7125000000000065725 ) ) ;
#12220=CARTESIAN_POINT ( 'NONE',  ( 10.31873187879411091, 3.604726614523236616, -9.628124999385549998 ) ) ;
#12221=CARTESIAN_POINT ( 'NONE',  ( 10.56230152254371824, -3.464101615137531009, -2.662500000000047162 ) ) ;
#12233=CARTESIAN_POINT ( 'NONE',  ( 10.31873187879410914, 0.000000000000000000, -3.290624999385538541 ) ) ;
#12241=CARTESIAN_POINT ( 'NONE',  ( 22.56230152254412147, 7.347880794884125653E-16, -3.825000000000050804 ) ) ;
#12247=DIRECTION ( 'NONE',  ( 1.000000000000000000, 0.000000000000000000, 0.000000000000000000 ) ) ;
#12255=( BOUNDED_CURVE ( )  B_SPLINE_CURVE ( 2, ( #7360, #13610, #25345, #21956, #33133, #36151, #27440 ),
 .UNSPECIFIED., .F., .F. ) 
 B_SPLINE_CURVE_WITH_KNOTS ( ( 3, 2, 2, 3 ),
 ( 0.3478260869565210078, 0.3550724637681152984, 0.3623188405797095890, 0.3695652173913038241 ),
 .UNSPECIFIED. ) 
 CURVE ( )  GEOMETRIC_REPRESENTATION_ITEM ( )  RATIONAL_B_SPLINE_CURVE ( ( 1.000000000000013323, 0.8660254037844252739, 1.000000000000000000, 0.8660254037844387076, 1.000000000000000000, 0.8660254037844479225, 0.9999999999999907851 ) ) 
 REPRESENTATION_ITEM ( '' )  );
#12270=CARTESIAN_POINT ( 'NONE',  ( 13.44051670066911441, 5.407089921784856479, -2.465624999385545912 ) ) ;
#12274=CARTESIAN_POINT ( 'NONE',  ( 10.56230152254410903, 0.000000000000000000, -4.500000000000031974 ) ) ;
#12290=ORIENTED_EDGE ( 'NONE', *, *, #32495, .F. ) ;
#12299=CARTESIAN_POINT ( 'NONE',  ( 22.80587116629410716, 7.646167579472015790E-16, -6.215624999385549465 ) ) ;
#12306=CARTESIAN_POINT ( 'NONE',  ( 22.56230152254411081, 3.464101615137755275, -6.824999998770996612 ) ) ;
#12311=CARTESIAN_POINT ( 'NONE',  ( 16.56230152254411436, -7.209453229046482114, -3.684374999385500615 ) ) ;
#12326=CARTESIAN_POINT ( 'NONE',  ( 22.56230152254410370, 7.347880794884117764E-16, -5.962499998771020771 ) ) ;
#12339=ORIENTED_EDGE ( 'NONE', *, *, #18881, .F. ) ;
#12340=CARTESIAN_POINT ( 'NONE',  ( 16.56230152254411792, 7.209453229046482114, -4.359374999385510208 ) ) ;
#12362=CARTESIAN_POINT ( 'NONE',  ( 10.56230152254410726, 3.464101615137757051, -5.887500000000069456 ) ) ;
#12379=CARTESIAN_POINT ( 'NONE',  ( 22.80587116629411781, 3.604726614523243278, -3.084374999385516514 ) ) ;
#12386=ORIENTED_EDGE ( 'NONE', *, *, #30218, .T. ) ;
#12388=CARTESIAN_POINT ( 'NONE',  ( 22.56230152254349974, 3.464101615138115875, -1.087500000000032774 ) ) ;
#12398=CARTESIAN_POINT ( 'NONE',  ( 22.56230152254358501, 3.464101615138066137, -7.387500000000006395 ) ) ;
#12412=CARTESIAN_POINT ( 'NONE',  ( 10.56230152254410903, 0.000000000000000000, -2.700000000000063238 ) ) ;
#12414=CARTESIAN_POINT ( 'NONE',  ( 10.56230152254411081, 0.000000000000000000, -7.537499998771012955 ) ) ;
#12425=CARTESIAN_POINT ( 'NONE',  ( 19.68408634441910721, 5.407089921784857367, -6.140624999385558169 ) ) ;
#12440=EDGE_CURVE ( 'NONE', #17872, #6483, #21132, .T. ) ;
#12449=CARTESIAN_POINT ( 'NONE',  ( 22.56230152254410370, 7.347880794884117764E-16, -4.612499998771030008 ) ) ;
#12454=VERTEX_POINT ( 'NONE', #23978 ) ;
#12461=CARTESIAN_POINT ( 'NONE',  ( 10.31873187879411446, -3.604726614523240613, -2.803124999385555149 ) ) ;
#12472=CARTESIAN_POINT ( 'NONE',  ( 22.56230152254396160, -3.464101615137847645, -6.562500000000048850 ) ) ;
#12475=CARTESIAN_POINT ( 'NONE',  ( 16.56230152254410726, 0.000000000000000000, -10.00000000000000000 ) ) ;
#12480=ORIENTED_EDGE ( 'NONE', *, *, #2868, .T. ) ;
#12492=CARTESIAN_POINT ( 'NONE',  ( 19.68408634441910721, -5.407089921784855591, -4.940624999385550886 ) ) ;
#12499=CARTESIAN_POINT ( 'NONE',  ( 22.56230152254411792, -3.464101615137751278, -5.549999998771003362 ) ) ;
#12500=ADVANCED_FACE ( 'NONE', ( #32487 ), #3686, .F. ) ;
#12502=( BOUNDED_CURVE ( )  B_SPLINE_CURVE ( 2, ( #6079, #8934, #3428, #19637, #5204, #10896, #32049 ),
 .UNSPECIFIED., .F., .F. ) 
 B_SPLINE_CURVE_WITH_KNOTS ( ( 3, 2, 2, 3 ),
 ( 0.1086956521739117498, 0.1159420289855060821, 0.1231884057971004143, 0.1304347826086947326 ),
 .UNSPECIFIED. ) 
 CURVE ( )  GEOMETRIC_REPRESENTATION_ITEM ( )  RATIONAL_B_SPLINE_CURVE ( ( 1.000000000000023759, 0.8660254037844148378, 1.000000000000000000, 0.8660254037844387076, 1.000000000000000000, 0.8660254037844556940, 0.9999999999999830136 ) ) 
 REPRESENTATION_ITEM ( '' )  );
#12506=CARTESIAN_POINT ( 'NONE',  ( 13.44051670066911441, -5.407089921784865361, -5.071874999385522997 ) ) ;
#12508=CARTESIAN_POINT ( 'NONE',  ( 10.56230152254442700, 3.464101615137936019, -7.124999998771008869 ) ) ;
#12509=CARTESIAN_POINT ( 'NONE',  ( 10.56230152254410903, 7.347880794884117764E-16, -10.00000000000000000 ) ) ;
#12520=CARTESIAN_POINT ( 'NONE',  ( 16.56230152254411436, 6.928203230275514990, -7.762500000000014388 ) ) ;
#12535=CARTESIAN_POINT ( 'NONE',  ( 16.56230152254411436, 7.209453229046482114, -5.259374999385502569 ) ) ;
#12537=ORIENTED_EDGE ( 'NONE', *, *, #34486, .T. ) ;
#12555=CARTESIAN_POINT ( 'NONE',  ( 10.56230152254410903, 0.000000000000000000, -7.200000000000040146 ) ) ;
#12559=CARTESIAN_POINT ( 'NONE',  ( 22.56230152254410370, 0.000000000000000000, -10.00000000000000000 ) ) ;
#12564=CARTESIAN_POINT ( 'NONE',  ( 21.13469769562223988, -4.064762008813216809, -9.999999999999996447 ) ) ;
#12572=CARTESIAN_POINT ( 'NONE',  ( 10.31873187879410558, 3.604726614523240613, -3.384374999385492355 ) ) ;
#12595=CARTESIAN_POINT ( 'NONE',  ( 19.56230152254412502, 5.196152422706637353, -0.1500000000000112355 ) ) ;
#12612=CARTESIAN_POINT ( 'NONE',  ( 22.80587116629411071, -3.604726614523235284, -5.803124999385537386 ) ) ;
#12616=EDGE_CURVE ( 'NONE', #31449, #15078, #35522, .T. ) ;
#12622=CARTESIAN_POINT ( 'NONE',  ( 22.56230152254433818, -3.464101615137632706, -3.862500000000038014 ) ) ;
#12649=CARTESIAN_POINT ( 'NONE',  ( 16.56230152254411081, 7.209453229046475009, -4.303124999385498306 ) ) ;
#12671=CARTESIAN_POINT ( 'NONE',  ( 10.56230152254241439, -3.464101615136776946, -9.299999998771010468 ) ) ;
#12678=CARTESIAN_POINT ( 'NONE',  ( 16.56230152254411081, 7.209453229046475009, -7.903124999385497063 ) ) ;
#12684=CARTESIAN_POINT ( 'NONE',  ( 13.56230152254411614, -5.196152422706632912, -5.212499998771047416 ) ) ;
#12687=CARTESIAN_POINT ( 'NONE',  ( 22.80587116629412847, -3.604726614523238837, -4.059374999385534366 ) ) ;
#12700=( BOUNDED_CURVE ( )  B_SPLINE_CURVE ( 2, ( #8183, #33951, #4391, #15971, #28074, #24862, #36410 ),
 .UNSPECIFIED., .F., .F. ) 
 B_SPLINE_CURVE_WITH_KNOTS ( ( 3, 2, 2, 3 ),
 ( 0.7608695652173907975, 0.7681159420289841444, 0.7753623188405776023, 0.7826086956521710603 ),
 .UNSPECIFIED. ) 
 CURVE ( )  GEOMETRIC_REPRESENTATION_ITEM ( )  RATIONAL_B_SPLINE_CURVE ( ( 1.000000000000010214, 0.8660254037844284936, 1.000000000000000000, 0.8660254037844387076, 1.000000000000000000, 0.8660254037844921093, 0.9999999999999465983 ) ) 
 REPRESENTATION_ITEM ( '' )  );
#12704=CARTESIAN_POINT ( 'NONE',  ( 19.68408634441910721, -5.407089921784855591, -0.4406249993855471114 ) ) ;
#12712=ADVANCED_FACE ( 'NONE', ( #35893 ), #11924, .T. ) ;
#12719=CARTESIAN_POINT ( 'NONE',  ( 10.31873187879411091, 3.604726614523240613, -6.984374999385521754 ) ) ;
#12720=EDGE_LOOP ( 'NONE', ( #3642, #6101 ) ) ;
#12741=CARTESIAN_POINT ( 'NONE',  ( 19.56230152254411792, 5.196152422706637353, -7.800000000000029132 ) ) ;
#12745=CARTESIAN_POINT ( 'NONE',  ( 19.56230152254411081, -5.196152422706629359, -6.037499998771039600 ) ) ;
#12758=CARTESIAN_POINT ( 'NONE',  ( 13.44051670066911086, 5.407089921784862696, -3.871874999385516158 ) ) ;
#12786=CARTESIAN_POINT ( 'NONE',  ( 10.56230152254527788, 3.464101615138426737, -8.474999998771037824 ) ) ;
#12789=CARTESIAN_POINT ( 'NONE',  ( 19.56230152254410370, 5.196152422706631135, -7.687499998771024856 ) ) ;
#12791=DIRECTION ( 'NONE',  ( 0.000000000000000000, 0.000000000000000000, 1.000000000000000000 ) ) ;
#12797=CARTESIAN_POINT ( 'NONE',  ( 10.31873187879411091, -3.604726614523240613, -6.853124999385484806 ) ) ;
#12802=ORIENTED_EDGE ( 'NONE', *, *, #21001, .F. ) ;
#12813=CARTESIAN_POINT ( 'NONE',  ( 16.56230152254411436, 6.928203230275506996, -4.949999998771019705 ) ) ;
#12834=CARTESIAN_POINT ( 'NONE',  ( 22.80587116629411071, -3.604726614523235284, -4.453124999385550176 ) ) ;
#12852=EDGE_CURVE ( 'NONE', #29586, #21112, #25219, .T. ) ;
#12867=CARTESIAN_POINT ( 'NONE',  ( 16.56230152254411081, 7.209453229046475009, -8.803124999385518734 ) ) ;
#12872=CARTESIAN_POINT ( 'NONE',  ( 10.56230152254410548, 3.464101615137752166, -8.024999998771027876 ) ) ;
#12873=CARTESIAN_POINT ( 'NONE',  ( 22.56230152254411792, 7.347880794884125653E-16, -1.125000000000042633 ) ) ;
#12875=CARTESIAN_POINT ( 'NONE',  ( 19.68408634441910721, 5.407089921784862696, -4.396874999385541827 ) ) ;
#12882=EDGE_CURVE ( 'NONE', #23999, #21775, #27374, .T. ) ;
#12889=CARTESIAN_POINT ( 'NONE',  ( 13.56230152254411614, -5.196152422706632912, -5.212499998771047416 ) ) ;
#12896=CARTESIAN_POINT ( 'NONE',  ( 13.44051670066911264, -5.407089921784859143, -3.215624999385519267 ) ) ;
#12909=CARTESIAN_POINT ( 'NONE',  ( 16.56230152254411436, -7.209453229046482114, -5.934374999385512162 ) ) ;
#12919=LINE ( 'NONE', #13105, #30324 ) ;
#12928=EDGE_CURVE ( 'NONE', #15078, #13979, #5832, .T. ) ;
#12929=( BOUNDED_CURVE ( )  B_SPLINE_CURVE ( 2, ( #33791, #7830, #8202, #27912, #7456, #22611, #30766 ),
 .UNSPECIFIED., .F., .F. ) 
 B_SPLINE_CURVE_WITH_KNOTS ( ( 3, 2, 2, 3 ),
 ( 0.8695652173913078764, 0.8768115942029022225, 0.8840579710144965686, 0.8913043478260908037 ),
 .UNSPECIFIED. ) 
 CURVE ( )  GEOMETRIC_REPRESENTATION_ITEM ( )  RATIONAL_B_SPLINE_CURVE ( ( 0.9999999999999342748, 0.8660254037845044328, 1.000000000000000000, 0.8660254037844387076, 1.000000000000000000, 0.8660254037843668762, 1.000000000000071942 ) ) 
 REPRESENTATION_ITEM ( '' )  );
#12932=CARTESIAN_POINT ( 'NONE',  ( 13.56230152254411614, -5.196152422706638241, -8.025000000000058975 ) ) ;
#12948=CARTESIAN_POINT ( 'NONE',  ( 19.68408634441911786, -5.407089921784861808, -4.096874999385518912 ) ) ;
#12952=( BOUNDED_CURVE ( )  B_SPLINE_CURVE ( 2, ( #18980, #1708, #30721, #27864, #28034, #34282, #10785 ),
 .UNSPECIFIED., .F., .F. ) 
 B_SPLINE_CURVE_WITH_KNOTS ( ( 3, 2, 2, 3 ),
 ( 0.02173913043478281973, 0.02898550724637714848, 0.03623188405797147377, 0.04347826086956579905 ),
 .UNSPECIFIED. ) 
 CURVE ( )  GEOMETRIC_REPRESENTATION_ITEM ( )  RATIONAL_B_SPLINE_CURVE ( ( 0.9999999999999961142, 0.8660254037844425934, 1.000000000000000000, 0.8660254037844387076, 1.000000000000000000, 0.8660254037844279384, 1.000000000000010658 ) ) 
 REPRESENTATION_ITEM ( '' )  );
#12966=DIRECTION ( 'NONE',  ( 1.000000000000000000, 0.000000000000000000, 0.000000000000000000 ) ) ;
#12989=ORIENTED_EDGE ( 'NONE', *, *, #20849, .F. ) ;
#12993=CARTESIAN_POINT ( 'NONE',  ( 19.68408634441910721, 5.407089921784857367, -7.940624999385553551 ) ) ;
#12997=VERTEX_POINT ( 'NONE', #7 ) ;
#13001=DIRECTION ( 'NONE',  ( 0.000000000000000000, 0.000000000000000000, 1.000000000000000000 ) ) ;
#13009=CARTESIAN_POINT ( 'NONE',  ( 19.56230152254411081, 5.196152422706631135, -4.987499998771016685 ) ) ;
#13028=CARTESIAN_POINT ( 'NONE',  ( 10.31873187879411091, -3.604726614523240613, -3.703124999385514649 ) ) ;
#13033=EDGE_CURVE ( 'NONE', #21578, #2980, #5693, .T. ) ;
#13060=CARTESIAN_POINT ( 'NONE',  ( 13.44051670066910908, 5.407089921784856479, -7.865624999385534721 ) ) ;
#13065=CARTESIAN_POINT ( 'NONE',  ( 10.56230152254410726, 0.000000000000000000, -8.887499998771003717 ) ) ;
#13069=CARTESIAN_POINT ( 'NONE',  ( 19.68408634441911431, 5.407089921784862696, -6.196874999385537208 ) ) ;
#13088=VERTEX_POINT ( 'NONE', #25790 ) ;
#13096=CARTESIAN_POINT ( 'NONE',  ( 22.80587116629411781, 7.646167579472024665E-16, -5.371874999385517491 ) ) ;
#13100=CARTESIAN_POINT ( 'NONE',  ( 19.68408634441910721, 5.407089921784857367, -0.7406249993855418268 ) ) ;
#13105=CARTESIAN_POINT ( 'NONE',  ( 10.56230152254410903, 7.347880794884117764E-16, -10.00000000000000000 ) ) ;
#13108=CARTESIAN_POINT ( 'NONE',  ( 10.56230152254411436, 3.464101615137752166, -1.724999998770991416 ) ) ;
#13118=CARTESIAN_POINT ( 'NONE',  ( 10.56230152254410726, 0.000000000000000000, -8.550000000000029132 ) ) ;
#13119=ORIENTED_EDGE ( 'NONE', *, *, #36911, .T. ) ;
#13122=CARTESIAN_POINT ( 'NONE',  ( 22.56230152254410370, 7.347880794884117764E-16, -5.962499998771020771 ) ) ;
#13125=CARTESIAN_POINT ( 'NONE',  ( 16.56230152254410726, 0.000000000000000000, -10.00000000000000000 ) ) ;
#13128=CARTESIAN_POINT ( 'NONE',  ( 19.56230152254411792, 5.196152422706637353, -3.750000000000031086 ) ) ;
#13133=CARTESIAN_POINT ( 'NONE',  ( 19.68408634441911431, 5.407089921784862696, -6.196874999385537208 ) ) ;
#13157=CARTESIAN_POINT ( 'NONE',  ( 19.56230152254411792, 5.196152422706637353, -3.300000000000025135 ) ) ;
#13175=CARTESIAN_POINT ( 'NONE',  ( 13.44051670066911441, -5.407089921784859143, -5.915624999385554972 ) ) ;
#13190=EDGE_CURVE ( 'NONE', #28808, #2436, #17475, .T. ) ;
#13197=AXIS2_PLACEMENT_3D ( 'NONE', #17541, #3869, #23407 ) ;
#13217=CARTESIAN_POINT ( 'NONE',  ( 10.31873187879411269, 3.604726614523236616, -4.678124999385532945 ) ) ;
#13221=CARTESIAN_POINT ( 'NONE',  ( 10.31873187879410736, 3.604726614523240613, -9.684374999385530813 ) ) ;
#13224=CLOSED_SHELL ( 'NONE', ( #3888, #18471, #23841, #30820, #34941, #14472, #15637, #27001, #10100, #12500, #27031, #3044, #24022, #10573, #28705, #15630, #11196, #4699, #24570, #28797, #6100, #5643, #16968, #23276, #18656, #26137, #4095, #28777, #17379, #27683, #30228, #1250, #5082, #19452, #23498, #25921, #2780, #29928, #35543, #25131, #26830, #30969, #14207, #8986, #20258, #26605, #9174, #17710, #11910, #16228, #37364, #3675, #3373, #6240, #15340, #12712, #135, #16143 ) ) ;
#13228=CARTESIAN_POINT ( 'NONE',  ( 13.44051670066911086, 5.407089921784862696, -1.171874999385535965 ) ) ;
#13249=CARTESIAN_POINT ( 'NONE',  ( 10.31873187879411091, -3.604726614523240613, -6.853124999385484806 ) ) ;
#13250=AXIS2_PLACEMENT_3D ( 'NONE', #28209, #24987, #11151 ) ;
#13255=CARTESIAN_POINT ( 'NONE',  ( 19.56230152254411436, -5.196152422706629359, -8.287499998771014731 ) ) ;
#13258=CARTESIAN_POINT ( 'NONE',  ( 22.80587116629411781, 3.604726614523243278, -6.684374999385514826 ) ) ;
#13261=CARTESIAN_POINT ( 'NONE',  ( 10.56230152254410726, 0.000000000000000000, -5.850000000000049383 ) ) ;
#13263=CARTESIAN_POINT ( 'NONE',  ( 16.56230152254411436, 6.928203230275514990, -3.262500000000057021 ) ) ;
#13280=CARTESIAN_POINT ( 'NONE',  ( 10.56230152254410903, 0.000000000000000000, -2.250000000000057732 ) ) ;
#13282=CARTESIAN_POINT ( 'NONE',  ( 10.31873187879410736, 3.604726614523240613, -5.184374999385507721 ) ) ;
#13286=CARTESIAN_POINT ( 'NONE',  ( 13.44051670066910908, -5.407089921784859143, -0.5156249993855110958 ) ) ;
#13294=CARTESIAN_POINT ( 'NONE',  ( 10.56230152254410903, 0.000000000000000000, -1.687499998771019305 ) ) ;
#13301=EDGE_CURVE ( 'NONE', #26963, #31128, #4396, .T. ) ;
#13302=CARTESIAN_POINT ( 'NONE',  ( 19.56230152254411792, 5.196152422706637353, -9.600000000000052935 ) ) ;
#13312=EDGE_CURVE ( 'NONE', #19909, #31630, #21619, .T. ) ;
#13318=CARTESIAN_POINT ( 'NONE',  ( 10.31873187879411091, 3.604726614523240613, -6.984374999385522642 ) ) ;
#13330=CARTESIAN_POINT ( 'NONE',  ( 10.56230152254410548, 0.000000000000000000, -9.450000000000041922 ) ) ;
#13342=CARTESIAN_POINT ( 'NONE',  ( 13.56230152254410726, 5.196152422706636465, -0.9750000000000591527 ) ) ;
#13344=VERTEX_POINT ( 'NONE', #5650 ) ;
#13357=EDGE_LOOP ( 'NONE', ( #34103, #29203, #1088, #2545 ) ) ;
#13360=CARTESIAN_POINT ( 'NONE',  ( 10.31873187879411269, 3.604726614523236616, -9.178124999385520510 ) ) ;
#13362=DIRECTION ( 'NONE',  ( 0.000000000000000000, 0.000000000000000000, 1.000000000000000000 ) ) ;
#13364=ORIENTED_EDGE ( 'NONE', *, *, #25401, .T. ) ;
#13399=CARTESIAN_POINT ( 'NONE',  ( 13.44051670066911797, -5.407089921784859143, -6.365624999385560479 ) ) ;
#13406=CARTESIAN_POINT ( 'NONE',  ( 10.56230152254410548, 0.000000000000000000, -6.750000000000061284 ) ) ;
#13408=CARTESIAN_POINT ( 'NONE',  ( 19.68408634441912142, -5.407089921784861808, -2.296874999385551064 ) ) ;
#13416=CARTESIAN_POINT ( 'NONE',  ( 22.56230152254410015, 7.347880794884117764E-16, -2.812499998771006204 ) ) ;
#13429=CARTESIAN_POINT ( 'NONE',  ( 10.31873187879410914, 0.000000000000000000, -8.690624999385526905 ) ) ;
#13434=EDGE_CURVE ( 'NONE', #33087, #31762, #24983, .T. ) ;
#13436=CARTESIAN_POINT ( 'NONE',  ( 16.56230152254410015, -6.928203230275506996, -7.874999998770975118 ) ) ;
#13441=CARTESIAN_POINT ( 'NONE',  ( 16.56230152254411436, -7.209453229046482114, -7.284374999385498484 ) ) ;
#13442=CARTESIAN_POINT ( 'NONE',  ( 10.56230152254410903, 0.000000000000000000, -1.800000000000051559 ) ) ;
#13445=DIRECTION ( 'NONE',  ( -0.000000000000000000, -0.000000000000000000, -1.000000000000000000 ) ) ;
#13448=CARTESIAN_POINT ( 'NONE',  ( 19.56230152254411792, 5.196152422706637353, -3.300000000000025135 ) ) ;
#13469=CARTESIAN_POINT ( 'NONE',  ( 10.31873187879410736, 0.000000000000000000, -7.846874999385494931 ) ) ;
#13470=ORIENTED_EDGE ( 'NONE', *, *, #4155, .F. ) ;
#13473=CARTESIAN_POINT ( 'NONE',  ( 22.80587116629410716, 7.646167579472015790E-16, -1.265624999385539518 ) ) ;
#13479=CARTESIAN_POINT ( 'NONE',  ( 16.56230152254411081, -6.928203230275506996, -1.574999998771003495 ) ) ;
#13485=CARTESIAN_POINT ( 'NONE',  ( 10.56230152254410726, 0.000000000000000000, -9.900000000000048317 ) ) ;
#13489=CARTESIAN_POINT ( 'NONE',  ( 13.56230152254410548, 5.196152422706630247, -2.212499998771017218 ) ) ;
#13492=DIRECTION ( 'NONE',  ( 1.000000000000000000, 0.000000000000000000, 0.000000000000000000 ) ) ;
#13496=( BOUNDED_CURVE ( )  B_SPLINE_CURVE ( 2, ( #17423, #342, #23294, #31444, #28404, #25567, #17614 ),
 .UNSPECIFIED., .F., .F. ) 
 B_SPLINE_CURVE_WITH_KNOTS ( ( 3, 2, 2, 3 ),
 ( 0.8695652173913026584, 0.8768115942028961163, 0.8840579710144895742, 0.8913043478260829211 ),
 .UNSPECIFIED. ) 
 CURVE ( )  GEOMETRIC_REPRESENTATION_ITEM ( )  RATIONAL_B_SPLINE_CURVE ( ( 1.000000000000030864, 0.8660254037844079544, 1.000000000000000000, 0.8660254037844387076, 1.000000000000000000, 0.8660254037845126485, 0.9999999999999260591 ) ) 
 REPRESENTATION_ITEM ( '' )  );
#13502=CARTESIAN_POINT ( 'NONE',  ( 10.31873187879411091, 3.604726614523240613, -6.534374999385494043 ) ) ;
#13507=EDGE_LOOP ( 'NONE', ( #15171, #32913, #21591, #27413 ) ) ;
#13509=CARTESIAN_POINT ( 'NONE',  ( 19.68408634441911076, 5.407089921784862696, -2.146874999385511629 ) ) ;
#13529=CARTESIAN_POINT ( 'NONE',  ( 10.56230152254410548, 3.464101615137757051, -2.737500000000003375 ) ) ;
#13548=CARTESIAN_POINT ( 'NONE',  ( 19.83830452692373925, 6.917534487978453051, -10.19247752355789416 ) ) ;
#13583=DIRECTION ( 'NONE',  ( 1.000000000000000000, 0.000000000000000000, 0.000000000000000000 ) ) ;
#13591=CARTESIAN_POINT ( 'NONE',  ( 19.68408634441910721, -5.407089921784855591, -7.190624999385525129 ) ) ;
#13600=CARTESIAN_POINT ( 'NONE',  ( 22.80587116629411426, -3.604726614523238837, -1.809374999385491511 ) ) ;
#13606=CARTESIAN_POINT ( 'NONE',  ( 10.31873187879411269, -3.604726614523240613, -1.003124999385540450 ) ) ;
#13610=CARTESIAN_POINT ( 'NONE',  ( 10.56230152254377153, 3.464101615137553658, -3.974999998771030274 ) ) ;
#13625=CARTESIAN_POINT ( 'NONE',  ( 12.11180837762981533, -4.639959813803625543, -9.981585920767699349 ) ) ;
#13631=CARTESIAN_POINT ( 'NONE',  ( 22.56230152254410726, 7.347880794884117764E-16, -9.562499998771039955 ) ) ;
#13635=CARTESIAN_POINT ( 'NONE',  ( 22.80587116629411781, 7.646167579472024665E-16, -9.871874999385521932 ) ) ;
#13636=CARTESIAN_POINT ( 'NONE',  ( 16.56230152254411436, 7.209453229046482114, -7.509374999385480365 ) ) ;
#13641=ORIENTED_EDGE ( 'NONE', *, *, #16190, .T. ) ;
#13649=CARTESIAN_POINT ( 'NONE',  ( 22.56230152254400068, -3.464101615137812562, -6.899999998771023435 ) ) ;
#13656=CARTESIAN_POINT ( 'NONE',  ( 16.56230152254410726, 0.000000000000000000, -10.00000000000000000 ) ) ;
#13663=CARTESIAN_POINT ( 'NONE',  ( 19.68408634441912142, -5.407089921784861808, -7.696874999385511451 ) ) ;
#13664=( BOUNDED_CURVE ( )  B_SPLINE_CURVE ( 2, ( #14191, #28764, #11343, #5642, #11708, #14934, #11526 ),
 .UNSPECIFIED., .F., .F. ) 
 B_SPLINE_CURVE_WITH_KNOTS ( ( 3, 2, 2, 3 ),
 ( 0.06521739130435129372, 0.07246376811594562595, 0.07971014492753994429, 0.08695652173913427652 ),
 .UNSPECIFIED. ) 
 CURVE ( )  GEOMETRIC_REPRESENTATION_ITEM ( )  RATIONAL_B_SPLINE_CURVE ( ( 0.9999999999999359401, 0.8660254037845028785, 1.000000000000000000, 0.8660254037844387076, 1.000000000000000000, 0.8660254037843676533, 1.000000000000071054 ) ) 
 REPRESENTATION_ITEM ( '' )  );
#13677=CARTESIAN_POINT ( 'NONE',  ( 16.56230152254411081, 6.928203230275506996, -1.799999998770985377 ) ) ;
#13685=CARTESIAN_POINT ( 'NONE',  ( 19.56230152254411792, 5.196152422706637353, -8.250000000000062172 ) ) ;
#13698=CARTESIAN_POINT ( 'NONE',  ( 10.31873187879411091, -3.604726614523244610, -5.559374999385509497 ) ) ;
#13704=CARTESIAN_POINT ( 'NONE',  ( 13.44051670066911086, 5.407089921784862696, -1.171874999385535965 ) ) ;
#13711=VECTOR ( 'NONE', #9230, 1000.000000000000000 ) ;
#13717=DIRECTION ( 'NONE',  ( 0.000000000000000000, 0.000000000000000000, 1.000000000000000000 ) ) ;
#13724=CARTESIAN_POINT ( 'NONE',  ( 10.56230152254411259, -3.464101615137761048, -2.212500000000045652 ) ) ;
#13744=CARTESIAN_POINT ( 'NONE',  ( 16.56230152254411081, -7.209453229046475009, -9.478124999385530103 ) ) ;
#13749=ORIENTED_EDGE ( 'NONE', *, *, #22810, .F. ) ;
#13750=ORIENTED_EDGE ( 'NONE', *, *, #22645, .F. ) ;
#13778=CARTESIAN_POINT ( 'NONE',  ( 13.44051670066911441, -5.407089921784859143, -5.915624999385554972 ) ) ;
#13788=CARTESIAN_POINT ( 'NONE',  ( 10.31873187879410558, 0.000000000000000000, -1.546874999385550176 ) ) ;
#13795=CARTESIAN_POINT ( 'NONE',  ( 19.68408634441910721, 5.407089921784857367, -2.090624999385559679 ) ) ;
#13801=ORIENTED_EDGE ( 'NONE', *, *, #29389, .T. ) ;
#13812=CARTESIAN_POINT ( 'NONE',  ( 10.31873187879410914, 0.000000000000000000, -9.590624999385537919 ) ) ;
#13821=CARTESIAN_POINT ( 'NONE',  ( 16.56230152254411436, 7.209453229046482114, -6.159374999385525129 ) ) ;
#13847=CARTESIAN_POINT ( 'NONE',  ( 22.56230152254411792, 7.347880794884125653E-16, -9.675000000000045119 ) ) ;
#13850=CARTESIAN_POINT ( 'NONE',  ( 10.31873187879410736, 3.604726614523240613, -8.784374999385505589 ) ) ;
#13853=CARTESIAN_POINT ( 'NONE',  ( 10.31873187879411091, -3.604726614523240613, -3.703124999385514649 ) ) ;
#13859=CARTESIAN_POINT ( 'NONE',  ( 19.56230152254411081, -5.196152422706629359, -1.087499998771029874 ) ) ;
#13867=CARTESIAN_POINT ( 'NONE',  ( 22.80587116629410716, 3.604726614523238837, -0.3281249993855308578 ) ) ;
#13879=CARTESIAN_POINT ( 'NONE',  ( 13.56230152254410548, 5.196152422706630247, -6.712499998771020771 ) ) ;
#13882=EDGE_LOOP ( 'NONE', ( #17930, #14347, #1656, #13749 ) ) ;
#13885=CARTESIAN_POINT ( 'NONE',  ( 22.80587116629411426, 3.604726614523243278, -7.134374999385543425 ) ) ;
#13890=CARTESIAN_POINT ( 'NONE',  ( 10.31873187879410736, 0.000000000000000000, -0.6468749993855105185 ) ) ;
#13891=DIRECTION ( 'NONE',  ( 0.000000000000000000, 0.000000000000000000, 1.000000000000000000 ) ) ;
#13896=DIRECTION ( 'NONE',  ( 0.000000000000000000, -1.000000000000000000, 0.000000000000000000 ) ) ;
#13907=CARTESIAN_POINT ( 'NONE',  ( 10.56230152254410903, 0.000000000000000000, -2.250000000000057732 ) ) ;
#13913=CARTESIAN_POINT ( 'NONE',  ( 22.56230152254410370, 7.347880794884117764E-16, -6.412499998770998744 ) ) ;
#13925=CARTESIAN_POINT ( 'NONE',  ( 16.56230152254410726, 7.209453229046475009, -9.253124999385514471 ) ) ;
#13927=( BOUNDED_CURVE ( )  B_SPLINE_CURVE ( 2, ( #7389, #33721, #36367, #13263, #13448, #36181, #18591 ),
 .UNSPECIFIED., .F., .F. ) 
 B_SPLINE_CURVE_WITH_KNOTS ( ( 3, 2, 2, 3 ),
 ( 0.3043478260869552643, 0.3115942028985494994, 0.3188405797101437900, 0.3260869565217380805 ),
 .UNSPECIFIED. ) 
 CURVE ( )  GEOMETRIC_REPRESENTATION_ITEM ( )  RATIONAL_B_SPLINE_CURVE ( ( 1.000000000000023759, 0.8660254037844151709, 1.000000000000000000, 0.8660254037844387076, 1.000000000000000000, 0.8660254037844582475, 0.9999999999999804601 ) ) 
 REPRESENTATION_ITEM ( '' )  );
#13960=CARTESIAN_POINT ( 'NONE',  ( 13.44051670066911619, -5.407089921784859143, -5.465624999385548577 ) ) ;
#13962=DIRECTION ( 'NONE',  ( 1.000000000000000000, 0.000000000000000000, 0.000000000000000000 ) ) ;
#13964=CARTESIAN_POINT ( 'NONE',  ( 10.56230152254410903, 0.000000000000000000, -7.200000000000040146 ) ) ;
#13969=CARTESIAN_POINT ( 'NONE',  ( 10.31873187879410736, -3.604726614523244610, -2.409374999385539340 ) ) ;
#13975=CARTESIAN_POINT ( 'NONE',  ( 16.56230152254411081, -7.209453229046475009, -2.278124999385533478 ) ) ;
#13979=VERTEX_POINT ( 'NONE', #33006 ) ;
#13980=ORIENTED_EDGE ( 'NONE', *, *, #29782, .T. ) ;
#13991=CARTESIAN_POINT ( 'NONE',  ( 10.31873187879410736, 3.604726614523236616, -9.628124999385549998 ) ) ;
#14001=CARTESIAN_POINT ( 'NONE',  ( 10.31873187879410736, -3.604726614523244610, -8.709374999385511629 ) ) ;
#14002=CARTESIAN_POINT ( 'NONE',  ( 22.56230152254411792, 7.347880794884125653E-16, -0.2250000000000584865 ) ) ;
#14008=CARTESIAN_POINT ( 'NONE',  ( 22.56230152254410370, 7.347880794884117764E-16, -3.712499998771018106 ) ) ;
#14028=CARTESIAN_POINT ( 'NONE',  ( 12.31958322920955062, -4.655204641349882877, -9.999999999999996447 ) ) ;
#14030=CARTESIAN_POINT ( 'NONE',  ( 22.80587116629411426, 3.604726614523243278, -7.584374999385507188 ) ) ;
#14034=CARTESIAN_POINT ( 'NONE',  ( 22.80587116629411426, 3.604726614523238837, -3.928124999385560923 ) ) ;
#14041=CARTESIAN_POINT ( 'NONE',  ( 19.56230152254411436, -5.196152422706629359, -3.787499998771037824 ) ) ;
#14047=EDGE_CURVE ( 'NONE', #29619, #2209, #19615, .T. ) ;
#14050=CARTESIAN_POINT ( 'NONE',  ( 22.80587116629410716, 3.604726614523238837, -2.578124999385541738 ) ) ;
#14052=ORIENTED_EDGE ( 'NONE', *, *, #6243, .F. ) ;
#14053=CARTESIAN_POINT ( 'NONE',  ( 22.56230152254410370, 7.347880794884117764E-16, -4.612499998771030008 ) ) ;
#14067=CARTESIAN_POINT ( 'NONE',  ( 16.56230152254411436, 7.209453229046482114, -8.409374999385503813 ) ) ;
#14071=CARTESIAN_POINT ( 'NONE',  ( 10.31873187879410736, 0.000000000000000000, -1.096874999385516469 ) ) ;
#14088=CARTESIAN_POINT ( 'NONE',  ( 19.56230152254412147, -5.196152422706635576, -5.700000000000065903 ) ) ;
#14094=CARTESIAN_POINT ( 'NONE',  ( 16.56230152254411081, -6.928203230275506996, -6.524999998771020771 ) ) ;
#14105=ORIENTED_EDGE ( 'NONE', *, *, #8631, .T. ) ;
#14107=CARTESIAN_POINT ( 'NONE',  ( 13.44051670066911264, 5.407089921784862696, -0.2718749993855240632 ) ) ;
#14131=CARTESIAN_POINT ( 'NONE',  ( 16.56230152254410726, -6.928203230275506996, -4.274999998770978138 ) ) ;
#14139=AXIS2_PLACEMENT_3D ( 'NONE', #33815, #15825, #7667 ) ;
#14142=CARTESIAN_POINT ( 'NONE',  ( 22.80587116629410360, 3.604726614523238837, -7.078124999385530636 ) ) ;
#14149=CARTESIAN_POINT ( 'NONE',  ( 10.56230152254447852, 3.464101615137971546, -6.787500000000034284 ) ) ;
#14156=CARTESIAN_POINT ( 'NONE',  ( 16.56230152254411081, 7.209453229046475009, -2.953124999385511096 ) ) ;
#14179=AXIS2_PLACEMENT_3D ( 'NONE', #20257, #3738, #514 ) ;
#14188=CARTESIAN_POINT ( 'NONE',  ( 22.80587116629411781, 7.646167579472024665E-16, -9.871874999385521932 ) ) ;
#14189=CARTESIAN_POINT ( 'NONE',  ( 10.56230152254410370, 3.464101615137757051, -0.03749999999999697325 ) ) ;
#14191=CARTESIAN_POINT ( 'NONE',  ( 22.56230152254410370, 7.347880794884117764E-16, -1.012499998771038134 ) ) ;
#14194=FACE_OUTER_BOUND ( 'NONE', #8937, .T. ) ;
#14195=ORIENTED_EDGE ( 'NONE', *, *, #195, .T. ) ;
#14207=ADVANCED_FACE ( 'NONE', ( #23001 ), #34550, .F. ) ;
#14218=CARTESIAN_POINT ( 'NONE',  ( 22.80587116629410716, 7.646167579472015790E-16, -3.965624999385547689 ) ) ;
#14223=CARTESIAN_POINT ( 'NONE',  ( 16.56230152254411081, -6.928203230275506996, -3.824999998771013932 ) ) ;
#14226=DIRECTION ( 'NONE',  ( 0.000000000000000000, 0.000000000000000000, 1.000000000000000000 ) ) ;
#14234=CARTESIAN_POINT ( 'NONE',  ( 19.68408634441910721, 5.407089921784857367, -2.540624999385538096 ) ) ;
#14252=CARTESIAN_POINT ( 'NONE',  ( 16.56230152254411081, -7.209453229046482114, -8.184374999385489957 ) ) ;
#14256=CARTESIAN_POINT ( 'NONE',  ( 16.56230152254411792, 7.209453229046482114, -1.659374999385503591 ) ) ;
#14275=CARTESIAN_POINT ( 'NONE',  ( 16.56230152254411436, 6.928203230275514990, -4.162500000000017408 ) ) ;
#14279=CARTESIAN_POINT ( 'NONE',  ( 22.56230152254427779, 3.464101615137667789, -6.487500000000022915 ) ) ;
#14293=CARTESIAN_POINT ( 'NONE',  ( 10.31873187879411091, -3.604726614523244610, -0.6093749993855241964 ) ) ;
#14327=CARTESIAN_POINT ( 'NONE',  ( 16.56230152254411081, -7.209453229046475009, -9.478124999385530103 ) ) ;
#14341=CARTESIAN_POINT ( 'NONE',  ( 13.44051670066911797, -5.407089921784859143, -3.665624999385552751 ) ) ;
#14347=ORIENTED_EDGE ( 'NONE', *, *, #35174, .T. ) ;
#14352=CONICAL_SURFACE ( 'NONE', #36422, 5.999999999999998224, 0.2617993877991499074 ) ;
#14358=CYLINDRICAL_SURFACE ( 'NONE', #27645, 5.999999999999998224 ) ;
#14368=CARTESIAN_POINT ( 'NONE',  ( 13.56230152254411436, -5.196152422706632912, -8.362499998771033560 ) ) ;
#14372=CARTESIAN_POINT ( 'NONE',  ( 13.44051670066911264, -5.407089921784865361, -8.671874999385515537 ) ) ;
#14373=CARTESIAN_POINT ( 'NONE',  ( 16.56230152254411792, 6.928203230275514990, -0.1125000000000229705 ) ) ;
#14384=CARTESIAN_POINT ( 'NONE',  ( 22.56230152254411792, 7.347880794884125653E-16, -6.075000000000052580 ) ) ;
#14400=CARTESIAN_POINT ( 'NONE',  ( 10.31873187879410914, 0.000000000000000000, -3.740624999385516958 ) ) ;
#14406=CARTESIAN_POINT ( 'NONE',  ( 22.56230152254412147, -3.464101615137751278, -3.299999998771024678 ) ) ;
#14414=FACE_OUTER_BOUND ( 'NONE', #34198, .T. ) ;
#14434=CARTESIAN_POINT ( 'NONE',  ( 22.80587116629411426, 3.604726614523243278, -7.584374999385505411 ) ) ;
#14438=CARTESIAN_POINT ( 'NONE',  ( 10.31873187879410381, 3.604726614523240613, -2.934374999385496618 ) ) ;
#14455=CARTESIAN_POINT ( 'NONE',  ( 22.56230152254412857, -3.464101615137755275, -3.862500000000040679 ) ) ;
#14472=ADVANCED_FACE ( 'NONE', ( #6689 ), #9905, .F. ) ;
#14476=CARTESIAN_POINT ( 'NONE',  ( 10.31873187879410914, 0.000000000000000000, -2.446874999385534544 ) ) ;
#14505=EDGE_CURVE ( 'NONE', #15610, #22453, #3837, .T. ) ;
#14510=CARTESIAN_POINT ( 'NONE',  ( 10.31873187879411091, -3.604726614523240613, -10.00312499938551802 ) ) ;
#14519=EDGE_LOOP ( 'NONE', ( #13364, #3521, #23713, #29150 ) ) ;
#14523=CARTESIAN_POINT ( 'NONE',  ( 19.68408634441911076, 5.407089921784857367, -5.240624999385545379 ) ) ;
#14552=CARTESIAN_POINT ( 'NONE',  ( 16.56230152254411081, 6.928203230275506996, -9.899999998771034981 ) ) ;
#14556=CARTESIAN_POINT ( 'NONE',  ( 10.31873187879410736, 0.000000000000000000, -8.296874999385501326 ) ) ;
#14563=CARTESIAN_POINT ( 'NONE',  ( 22.56230152254345711, 3.464101615138142520, -5.137500000000025935 ) ) ;
#14578=ORIENTED_EDGE ( 'NONE', *, *, #30423, .F. ) ;
#14586=CARTESIAN_POINT ( 'NONE',  ( 13.44051670066911441, 5.407089921784856479, -2.915624999385552307 ) ) ;
#14591=CARTESIAN_POINT ( 'NONE',  ( 16.56230152254410726, 0.000000000000000000, -10.00000000000000000 ) ) ;
#14593=CARTESIAN_POINT ( 'NONE',  ( 10.56230152254411259, -3.464101615137757051, -4.799999998770999809 ) ) ;
#14602=LINE ( 'NONE', #6055, #35690 ) ;
#14606=ORIENTED_EDGE ( 'NONE', *, *, #20289, .F. ) ;
#14610=CARTESIAN_POINT ( 'NONE',  ( 10.56230152254378929, 3.464101615137573198, -7.687500000000015987 ) ) ;
#14617=ORIENTED_EDGE ( 'NONE', *, *, #15854, .T. ) ;
#14621=CARTESIAN_POINT ( 'NONE',  ( 13.44051670066910908, 5.407089921784862696, -8.821874999385526550 ) ) ;
#14625=CARTESIAN_POINT ( 'NONE',  ( 22.80587116629412137, 7.646167579472024665E-16, -3.571874999385521221 ) ) ;
#14635=CYLINDRICAL_SURFACE ( 'NONE', #23393, 5.999999999999998224 ) ;
#14636=CARTESIAN_POINT ( 'NONE',  ( 19.56230152254412147, 5.196152422706637353, -1.500000000000029088 ) ) ;
#14643=CARTESIAN_POINT ( 'NONE',  ( 10.56230152254410903, 0.000000000000000000, -4.500000000000031974 ) ) ;
#14648=CARTESIAN_POINT ( 'NONE',  ( 19.56230152254411081, -5.196152422706629359, -6.487499998771045995 ) ) ;
#14650=FACE_OUTER_BOUND ( 'NONE', #17647, .T. ) ;
#14660=CARTESIAN_POINT ( 'NONE',  ( 22.80587116629411426, -3.604726614523238837, -1.809374999385491511 ) ) ;
#14666=ORIENTED_EDGE ( 'NONE', *, *, #12852, .F. ) ;
#14694=CARTESIAN_POINT ( 'NONE',  ( 13.44051670066911619, -5.407089921784859143, -9.065624999385569538 ) ) ;
#14695=CARTESIAN_POINT ( 'NONE',  ( 10.56230152254410903, 7.347880794884117764E-16, -10.00000000000000000 ) ) ;
#14698=CARTESIAN_POINT ( 'NONE',  ( 12.38894624757142360, 4.437320182635244414, -9.999999999999994671 ) ) ;
#14709=CARTESIAN_POINT ( 'NONE',  ( 10.31873187879411091, -3.604726614523240613, -3.703124999385514649 ) ) ;
#14715=ORIENTED_EDGE ( 'NONE', *, *, #14047, .T. ) ;
#14717=DIRECTION ( 'NONE',  ( 1.000000000000000000, 0.000000000000000000, -0.000000000000000000 ) ) ;
#14720=CARTESIAN_POINT ( 'NONE',  ( 22.56230152254410370, 7.347880794884117764E-16, -4.612499998771030008 ) ) ;
#14734=DIRECTION ( 'NONE',  ( 0.000000000000000000, 0.000000000000000000, 1.000000000000000000 ) ) ;
#14745=CARTESIAN_POINT ( 'NONE',  ( 13.44051670066911264, -5.407089921784865361, -7.771874999385531169 ) ) ;
#14751=EDGE_CURVE ( 'NONE', #31857, #10703, #16808, .T. ) ;
#14766=ORIENTED_EDGE ( 'NONE', *, *, #14505, .F. ) ;
#14778=CARTESIAN_POINT ( 'NONE',  ( 22.80587116629411071, -3.604726614523235284, -5.803124999385537386 ) ) ;
#14784=CARTESIAN_POINT ( 'NONE',  ( 22.56230152254410370, 3.464101615137755275, -3.674999998771026011 ) ) ;
#14788=CARTESIAN_POINT ( 'NONE',  ( 22.56230152254410726, 7.347880794884117764E-16, -3.262499998771012599 ) ) ;
#14793=DIRECTION ( 'NONE',  ( 1.000000000000000000, 0.000000000000000000, 0.000000000000000000 ) ) ;
#14801=EDGE_CURVE ( 'NONE', #8245, #36001, #33518, .T. ) ;
#14817=CARTESIAN_POINT ( 'NONE',  ( 16.56230152254411081, 7.209453229046482114, -3.909374999385482496 ) ) ;
#14835=CARTESIAN_POINT ( 'NONE',  ( 16.56230152254411436, 6.928203230275514990, -5.062500000000007994 ) ) ;
#14852=CARTESIAN_POINT ( 'NONE',  ( 10.31873187879410381, 3.604726614523240613, -1.134374999385481697 ) ) ;
#14857=VECTOR ( 'NONE', #5799, 1000.000000000000000 ) ;
#14884=CARTESIAN_POINT ( 'NONE',  ( 22.80587116629410360, 3.604726614523238837, -8.428124999385516958 ) ) ;
#14890=DIRECTION ( 'NONE',  ( 0.000000000000000000, 0.000000000000000000, -1.000000000000000000 ) ) ;
#14897=CARTESIAN_POINT ( 'NONE',  ( 22.80587116629411071, -3.604726614523235284, -4.903124999385513938 ) ) ;
#14908=FACE_OUTER_BOUND ( 'NONE', #5978, .T. ) ;
#14916=( BOUNDED_CURVE ( )  B_SPLINE_CURVE ( 2, ( #12083, #29520, #34830, #35387, #32741, #14563, #18165 ),
 .UNSPECIFIED., .F., .F. ) 
 B_SPLINE_CURVE_WITH_KNOTS ( ( 3, 2, 2, 3 ),
 ( 0.4782608695652158515, 0.4855072463768100866, 0.4927536231884043771, 0.4999999999999986122 ),
 .UNSPECIFIED. ) 
 CURVE ( )  GEOMETRIC_REPRESENTATION_ITEM ( )  RATIONAL_B_SPLINE_CURVE ( ( 1.000000000000028644, 0.8660254037844099528, 1.000000000000000000, 0.8660254037844387076, 1.000000000000000000, 0.8660254037844643538, 0.9999999999999743538 ) ) 
 REPRESENTATION_ITEM ( '' )  );
#14919=CARTESIAN_POINT ( 'NONE',  ( 16.56230152254411081, 6.928203230275506996, -4.499999998770991105 ) ) ;
#14923=CIRCLE ( 'NONE', #16738, 5.999999999999998224 ) ;
#14932=CARTESIAN_POINT ( 'NONE',  ( 13.44051670066911619, -5.407089921784859143, -0.9656249993855170466 ) ) ;
#14934=CARTESIAN_POINT ( 'NONE',  ( 10.56230152254227228, -3.464101615136696122, -1.199999998771057008 ) ) ;
#14935=PLANE ( 'NONE',  #14179 ) ;
#14938=DIRECTION ( 'NONE',  ( 0.000000000000000000, 0.000000000000000000, 1.000000000000000000 ) ) ;
#14955=VECTOR ( 'NONE', #3157, 1000.000000000000000 ) ;
#14963=CARTESIAN_POINT ( 'NONE',  ( 10.31873187879411269, 3.604726614523236616, -4.678124999385532945 ) ) ;
#14968=CARTESIAN_POINT ( 'NONE',  ( 22.56230152254410370, 3.464101615137755275, -5.024999998771013665 ) ) ;
#14984=CARTESIAN_POINT ( 'NONE',  ( 19.56230152254411081, -5.196152422706629359, -5.137499998771027698 ) ) ;
#14988=CARTESIAN_POINT ( 'NONE',  ( 16.56230152254411081, 7.209453229046475009, -0.7031249993855005487 ) ) ;
#14998=CARTESIAN_POINT ( 'NONE',  ( 16.56230152254411436, 7.209453229046482114, -2.559374999385494842 ) ) ;
#15014=PRODUCT_DEFINITION_SHAPE ( 'NONE', 'NONE',  #6956 ) ;
#15018=EDGE_CURVE ( 'NONE', #15581, #28127, #37362, .T. ) ;
#15019=CARTESIAN_POINT ( 'NONE',  ( 13.56230152254410548, 5.196152422706636465, -7.725000000000036948 ) ) ;
#15035=ORIENTED_EDGE ( 'NONE', *, *, #32395, .F. ) ;
#15039=CARTESIAN_POINT ( 'NONE',  ( 13.44051670066911086, 5.407089921784862696, -1.621874999385541916 ) ) ;
#15047=CARTESIAN_POINT ( 'NONE',  ( 16.56230152254410726, 0.000000000000000000, -10.00000000000000000 ) ) ;
#15070=CARTESIAN_POINT ( 'NONE',  ( 22.80587116629410716, 3.604726614523238837, -7.978124999385491023 ) ) ;
#15078=VERTEX_POINT ( 'NONE', #26350 ) ;
#15081=CARTESIAN_POINT ( 'NONE',  ( 19.56230152254411792, -5.196152422706629359, -3.337499998771031873 ) ) ;
#15082=CARTESIAN_POINT ( 'NONE',  ( 16.56230152254411081, -7.209453229046475009, -5.428124999385503635 ) ) ;
#15113=CARTESIAN_POINT ( 'NONE',  ( 22.56230152254411792, 7.347880794884125653E-16, -9.675000000000045119 ) ) ;
#15117=CARTESIAN_POINT ( 'NONE',  ( 13.44051670066911619, -5.407089921784859143, -1.415624999385550753 ) ) ;
#15143=AXIS2_PLACEMENT_3D ( 'NONE', #3690, #464, #12032 ) ;
#15147=CARTESIAN_POINT ( 'NONE',  ( 19.68408634441910721, -5.407089921784855591, -4.490624999385572913 ) ) ;
#15151=FACE_OUTER_BOUND ( 'NONE', #579, .T. ) ;
#15153=CARTESIAN_POINT ( 'NONE',  ( 13.56230152254410548, 5.196152422706630247, -6.262499998771015264 ) ) ;
#15155=( BOUNDED_CURVE ( )  B_SPLINE_CURVE ( 2, ( #1287, #30109, #35974, #10011, #15523, #12671, #35218 ),
 .UNSPECIFIED., .F., .F. ) 
 B_SPLINE_CURVE_WITH_KNOTS ( ( 3, 2, 2, 3 ),
 ( 0.8478260869565249491, 0.8550724637681192952, 0.8623188405797136413, 0.8695652173913078764 ),
 .UNSPECIFIED. ) 
 CURVE ( )  GEOMETRIC_REPRESENTATION_ITEM ( )  RATIONAL_B_SPLINE_CURVE ( ( 0.9999999999999404920, 0.8660254037844982156, 1.000000000000000000, 0.8660254037844387076, 1.000000000000000000, 0.8660254037843729824, 1.000000000000065725 ) ) 
 REPRESENTATION_ITEM ( '' )  );
#15160=CARTESIAN_POINT ( 'NONE',  ( 22.80587116629411781, 7.646167579472024665E-16, -4.921874999385511984 ) ) ;
#15171=ORIENTED_EDGE ( 'NONE', *, *, #30732, .T. ) ;
#15174=CARTESIAN_POINT ( 'NONE',  ( 10.56230152254485155, -3.464101615138189594, -4.912500000000042277 ) ) ;
#15176=CARTESIAN_POINT ( 'NONE',  ( 13.56230152254410548, 5.196152422706630247, -5.812499998771008869 ) ) ;
#15190=CARTESIAN_POINT ( 'NONE',  ( 10.31873187879411091, -3.604726614523244610, -3.759374999385526994 ) ) ;
#15198=CARTESIAN_POINT ( 'NONE',  ( 10.56230152254410903, 0.000000000000000000, -9.787499998771043153 ) ) ;
#15211=CARTESIAN_POINT ( 'NONE',  ( 16.56230152254411081, 6.928203230275514990, -6.412500000000027178 ) ) ;
#15219=CARTESIAN_POINT ( 'NONE',  ( 22.56230152254410370, 7.347880794884117764E-16, -1.462499998771016330 ) ) ;
#15228=CARTESIAN_POINT ( 'NONE',  ( 10.31873187879410558, 0.000000000000000000, -4.246874999385502392 ) ) ;
#15233=ORIENTED_EDGE ( 'NONE', *, *, #25845, .F. ) ;
#15241=CARTESIAN_POINT ( 'NONE',  ( 16.56230152254411436, 7.209453229046475009, -1.153124999385528371 ) ) ;
#15248=CARTESIAN_POINT ( 'NONE',  ( 22.56230152254411792, 7.347880794884125653E-16, -0.6750000000000366818 ) ) ;
#15271=CARTESIAN_POINT ( 'NONE',  ( 22.80587116629411071, -3.604726614523235284, -7.603124999385552307 ) ) ;
#15273=CARTESIAN_POINT ( 'NONE',  ( 19.56230152254411792, -5.196152422706629359, -2.437499998771047949 ) ) ;
#15277=ORIENTED_EDGE ( 'NONE', *, *, #34020, .T. ) ;
#15279=CARTESIAN_POINT ( 'NONE',  ( 19.56230152254411792, -5.196152422706629359, -1.987499998771014020 ) ) ;
#15285=EDGE_CURVE ( 'NONE', #11580, #20044, #32605, .T. ) ;
#15300=ORIENTED_EDGE ( 'NONE', *, *, #7804, .F. ) ;
#15303=AXIS2_PLACEMENT_3D ( 'NONE', #7164, #15503, #4120 ) ;
#15308=CARTESIAN_POINT ( 'NONE',  ( 13.44051670066911441, 5.407089921784856479, -0.6656249993855500868 ) ) ;
#15315=ORIENTED_EDGE ( 'NONE', *, *, #34344, .F. ) ;
#15339=CARTESIAN_POINT ( 'NONE',  ( 22.80587116629410716, 7.646167579472015790E-16, -4.415624999385525662 ) ) ;
#15340=ADVANCED_FACE ( 'NONE', ( #18031 ), #33743, .T. ) ;
#15345=CARTESIAN_POINT ( 'NONE',  ( 22.56230152254411081, -3.464101615137751278, -5.999999998770999099 ) ) ;
#15350=CARTESIAN_POINT ( 'NONE',  ( 13.44051670066911441, -5.407089921784865361, -4.171874999385538629 ) ) ;
#15351=CARTESIAN_POINT ( 'NONE',  ( 10.56230152254411081, 0.000000000000000000, -3.037499998771009402 ) ) ;
#15352=CARTESIAN_POINT ( 'NONE',  ( 13.56230152254410370, 5.196152422706630247, -7.162499998770998744 ) ) ;
#15363=CARTESIAN_POINT ( 'NONE',  ( 19.56230152254412147, -5.196152422706635576, -4.800000000000082423 ) ) ;
#15366=CARTESIAN_POINT ( 'NONE',  ( 10.56230152254411081, 0.000000000000000000, -3.037499998771009402 ) ) ;
#15379=CARTESIAN_POINT ( 'NONE',  ( 16.56230152254410726, 6.928203230275506996, -8.099999998770989862 ) ) ;
#15381=CARTESIAN_POINT ( 'NONE',  ( 10.31873187879410736, -3.604726614523244610, -6.909374999385496707 ) ) ;
#15394=ORIENTED_EDGE ( 'NONE', *, *, #15931, .F. ) ;
#15405=CARTESIAN_POINT ( 'NONE',  ( 10.56230152254410726, 0.000000000000000000, -6.300000000000055778 ) ) ;
#15413=CARTESIAN_POINT ( 'NONE',  ( 22.56378207682202586, 0.6013373594316471227, -10.00000000000000000 ) ) ;
#15421=CARTESIAN_POINT ( 'NONE',  ( 10.31873187879411091, -3.604726614523244610, -2.859374999385534633 ) ) ;
#15432=CARTESIAN_POINT ( 'NONE',  ( 10.31873187879410736, 3.604726614523236616, -0.1781249993854788494 ) ) ;
#15445=CARTESIAN_POINT ( 'NONE',  ( 10.56230152254410726, 0.000000000000000000, -0.9000000000000396572 ) ) ;
#15447=ORIENTED_EDGE ( 'NONE', *, *, #30218, .F. ) ;
#15458=EDGE_LOOP ( 'NONE', ( #25706, #4690, #657, #31084 ) ) ;
#15462=CARTESIAN_POINT ( 'NONE',  ( 22.80587116629410716, 3.604726614523238837, -7.528124999385559235 ) ) ;
#15471=CARTESIAN_POINT ( 'NONE',  ( 16.56230152254410726, 0.000000000000000000, -10.00000000000000000 ) ) ;
#15476=CARTESIAN_POINT ( 'NONE',  ( 19.56230152254412147, -5.196152422706635576, -5.700000000000065903 ) ) ;
#15498=CARTESIAN_POINT ( 'NONE',  ( 10.31873187879410914, 0.000000000000000000, -3.740624999385516958 ) ) ;
#15503=DIRECTION ( 'NONE',  ( 0.000000000000000000, 0.000000000000000000, 1.000000000000000000 ) ) ;
#15508=CARTESIAN_POINT ( 'NONE',  ( 10.56230152254410903, 0.000000000000000000, -1.800000000000051559 ) ) ;
#15523=CARTESIAN_POINT ( 'NONE',  ( 13.56230152254411614, -5.196152422706632912, -9.262499998771044574 ) ) ;
#15530=CARTESIAN_POINT ( 'NONE',  ( 16.56230152254411081, 7.209453229046475009, -5.653124999385517491 ) ) ;
#15536=CARTESIAN_POINT ( 'NONE',  ( 19.56230152254410726, 5.196152422706631135, -6.787499998771012955 ) ) ;
#15537=DIRECTION ( 'NONE',  ( 0.000000000000000000, 0.000000000000000000, 1.000000000000000000 ) ) ;
#15539=CARTESIAN_POINT ( 'NONE',  ( 13.44051670066911086, 5.407089921784862696, -3.421874999385537741 ) ) ;
#15540=CARTESIAN_POINT ( 'NONE',  ( 19.56230152254410370, 5.196152422706631135, -3.187499998770992882 ) ) ;
#15559=ORIENTED_EDGE ( 'NONE', *, *, #32387, .T. ) ;
#15560=ORIENTED_EDGE ( 'NONE', *, *, #29857, .T. ) ;
#15568=CARTESIAN_POINT ( 'NONE',  ( 22.80587116629411781, -3.604726614523238837, -5.859374999385516425 ) ) ;
#15581=VERTEX_POINT ( 'NONE', #32146 ) ;
#15589=CARTESIAN_POINT ( 'NONE',  ( 22.56230152254411792, 7.347880794884125653E-16, -6.075000000000052580 ) ) ;
#15596=CYLINDRICAL_SURFACE ( 'NONE', #27454, 5.999999999999998224 ) ;
#15605=CARTESIAN_POINT ( 'NONE',  ( 13.44051670066910908, 5.407089921784862696, -4.321874999385522109 ) ) ;
#15610=VERTEX_POINT ( 'NONE', #26271 ) ;
#15630=ADVANCED_FACE ( 'NONE', ( #14908 ), #17391, .F. ) ;
#15637=ADVANCED_FACE ( 'NONE', ( #32520 ), #32337, .F. ) ;
#15651=CARTESIAN_POINT ( 'NONE',  ( 22.80587116629410360, 3.604726614523238837, -7.078124999385530636 ) ) ;
#15653=CARTESIAN_POINT ( 'NONE',  ( 22.56230152254289578, -3.464101615138448054, -2.399999998770984799 ) ) ;
#15688=EDGE_CURVE ( 'NONE', #33455, #6605, #18247, .T. ) ;
#15689=CARTESIAN_POINT ( 'NONE',  ( 22.80587116629411426, 3.604726614523238837, -3.928124999385561367 ) ) ;
#15720=CARTESIAN_POINT ( 'NONE',  ( 10.31873187879411091, -3.604726614523240613, -8.653124999385532590 ) ) ;
#15725=CARTESIAN_POINT ( 'NONE',  ( 16.56230152254410726, -6.928203230275506996, -6.074999998771025034 ) ) ;
#15728=CARTESIAN_POINT ( 'NONE',  ( 16.56230152254411436, -7.209453229046482114, -4.584374999385491201 ) ) ;
#15745=CARTESIAN_POINT ( 'NONE',  ( 22.80587116629410716, 3.604726614523238837, -0.3281249993855308578 ) ) ;
#15749=ORIENTED_EDGE ( 'NONE', *, *, #13033, .T. ) ;
#15758=CARTESIAN_POINT ( 'NONE',  ( 19.68408634441912142, -5.407089921784861808, -7.246874999385532590 ) ) ;
#15781=CARTESIAN_POINT ( 'NONE',  ( 16.56230152254411081, -6.928203230275514990, -6.637500000000041034 ) ) ;
#15791=CARTESIAN_POINT ( 'NONE',  ( 22.56230152254247301, 3.464101615138709178, -5.587500000000009237 ) ) ;
#15797=CARTESIAN_POINT ( 'NONE',  ( 10.31873187879410558, 3.604726614523240613, -4.734374999385511984 ) ) ;
#15813=CARTESIAN_POINT ( 'NONE',  ( 10.56230152254410903, 0.000000000000000000, -0.4500000000000614619 ) ) ;
#15825=DIRECTION ( 'NONE',  ( 0.000000000000000000, 0.000000000000000000, 1.000000000000000000 ) ) ;
#15837=CARTESIAN_POINT ( 'NONE',  ( 13.44051670066910908, 5.407089921784856479, -7.865624999385534721 ) ) ;
#15839=DIRECTION ( 'NONE',  ( 0.000000000000000000, 0.000000000000000000, 1.000000000000000000 ) ) ;
#15854=EDGE_CURVE ( 'NONE', #16407, #9264, #34942, .T. ) ;
#15863=EDGE_CURVE ( 'NONE', #16407, #15581, #29871, .T. ) ;
#15878=CARTESIAN_POINT ( 'NONE',  ( 22.80587116629410360, 3.604726614523238837, -3.478124999385532767 ) ) ;
#15880=FACE_OUTER_BOUND ( 'NONE', #136, .T. ) ;
#15910=CARTESIAN_POINT ( 'NONE',  ( 10.31873187879411091, -3.604726614523240613, -7.303124999385512517 ) ) ;
#15915=CARTESIAN_POINT ( 'NONE',  ( 16.56230152254411081, -6.928203230275506996, -8.774999998770997678 ) ) ;
#15919=CARTESIAN_POINT ( 'NONE',  ( 10.31873187879410558, 3.604726614523240613, -4.734374999385511984 ) ) ;
#15926=CARTESIAN_POINT ( 'NONE',  ( 19.56230152254412502, 5.196152422706637353, -4.650000000000070521 ) ) ;
#15928=ORIENTED_EDGE ( 'NONE', *, *, #30706, .F. ) ;
#15931=EDGE_CURVE ( 'NONE', #27686, #20044, #12929, .T. ) ;
#15937=CARTESIAN_POINT ( 'NONE',  ( 16.56230152254411436, 7.209453229046475009, -1.153124999385528371 ) ) ;
#15948=CARTESIAN_POINT ( 'NONE',  ( 22.80587116629411426, 7.646167579472024665E-16, -6.271874999385529392 ) ) ;
#15959=CARTESIAN_POINT ( 'NONE',  ( 10.31873187879410558, 3.604726614523240613, -10.13437499938549280 ) ) ;
#15961=AXIS2_PLACEMENT_3D ( 'NONE', #13125, #24679, #13492 ) ;
#15969=CARTESIAN_POINT ( 'NONE',  ( 22.56230152254412147, 7.347880794884125653E-16, -8.325000000000027711 ) ) ;
#15971=CARTESIAN_POINT ( 'NONE',  ( 16.56230152254411436, -6.928203230275514990, -7.987500000000027356 ) ) ;
#15976=EDGE_CURVE ( 'NONE', #32727, #35189, #4232, .T. ) ;
#15988=CARTESIAN_POINT ( 'NONE',  ( 22.80587116629412847, -3.604726614523238837, -4.059374999385534366 ) ) ;
#16000=CARTESIAN_POINT ( 'NONE',  ( 10.56230152254410726, 0.000000000000000000, -8.100000000000024514 ) ) ;
#16003=VECTOR ( 'NONE', #1625, 1000.000000000000000 ) ;
#16020=CARTESIAN_POINT ( 'NONE',  ( 16.56230152254411436, 6.928203230275506996, -7.649999998770994125 ) ) ;
#16024=VERTEX_POINT ( 'NONE', #16000 ) ;
#16028=CARTESIAN_POINT ( 'NONE',  ( 16.56230152254411081, -7.209453229046475009, -5.878124999385531346 ) ) ;
#16038=CARTESIAN_POINT ( 'NONE',  ( 22.56230152254602928, -3.464101615136651713, -9.262499999999995737 ) ) ;
#16044=CARTESIAN_POINT ( 'NONE',  ( 22.56230152254411792, 7.347880794884125653E-16, -5.625000000000018652 ) ) ;
#16047=CARTESIAN_POINT ( 'NONE',  ( 0.000000000000000000, 0.000000000000000000, 0.000000000000000000 ) ) ;
#16066=CARTESIAN_POINT ( 'NONE',  ( 10.31873187879411091, 0.000000000000000000, -4.640624999385528859 ) ) ;
#16070=CARTESIAN_POINT ( 'NONE',  ( 10.31873187879410381, 0.000000000000000000, -9.646874999385518734 ) ) ;
#16075=CARTESIAN_POINT ( 'NONE',  ( 22.80587116629411781, -3.604726614523238837, -0.9093749993854999270 ) ) ;
#16082=DIRECTION ( 'NONE',  ( 0.000000000000000000, 0.000000000000000000, -1.000000000000000000 ) ) ;
#16095=CARTESIAN_POINT ( 'NONE',  ( 22.80587116629411071, 7.646167579472015790E-16, -8.915624999385585170 ) ) ;
#16102=CARTESIAN_POINT ( 'NONE',  ( 10.56230152254410903, 3.464101615137752166, -8.924999998771019349 ) ) ;
#16106=CARTESIAN_POINT ( 'NONE',  ( 16.56230152254411081, 7.209453229046482114, -5.709374999385496530 ) ) ;
#16133=CARTESIAN_POINT ( 'NONE',  ( 22.80587116629411781, 7.646167579472024665E-16, -5.821874999385522997 ) ) ;
#16137=CARTESIAN_POINT ( 'NONE',  ( 13.44051670066911619, -5.407089921784859143, -0.9656249993855170466 ) ) ;
#16143=ADVANCED_FACE ( 'NONE', ( #16369 ), #22615, .F. ) ;
#16147=CARTESIAN_POINT ( 'NONE',  ( 10.56230152254410903, 3.464101615137752166, -2.174999998770987375 ) ) ;
#16156=CARTESIAN_POINT ( 'NONE',  ( 22.56230152254412147, -3.464101615137755275, -9.262500000000022382 ) ) ;
#16165=CARTESIAN_POINT ( 'NONE',  ( 10.56230152254410903, 0.000000000000000000, 10.00000000000000000 ) ) ;
#16172=CARTESIAN_POINT ( 'NONE',  ( 10.31873187879410558, 3.604726614523240613, -5.634374999385534544 ) ) ;
#16188=CARTESIAN_POINT ( 'NONE',  ( 16.56230152254410726, 0.000000000000000000, -10.00000000000000000 ) ) ;
#16189=CARTESIAN_POINT ( 'NONE',  ( 22.56230152254428489, -3.464101615137663348, -6.112500000000050449 ) ) ;
#16190=EDGE_CURVE ( 'NONE', #25502, #11580, #7836, .T. ) ;
#16196=CARTESIAN_POINT ( 'NONE',  ( 19.56230152254412502, -5.196152422706635576, -1.650000000000068079 ) ) ;
#16198=ORIENTED_EDGE ( 'NONE', *, *, #37122, .F. ) ;
#16213=CARTESIAN_POINT ( 'NONE',  ( 16.56230152254411081, 7.209453229046475009, -8.803124999385520510 ) ) ;
#16215=CARTESIAN_POINT ( 'NONE',  ( 8.562301522544109034, 9.797174393178823685E-16, -10.00000000000000000 ) ) ;
#16228=ADVANCED_FACE ( 'NONE', ( #30768 ), #2324, .T. ) ;
#16241=VECTOR ( 'NONE', #6267, 1000.000000000000000 ) ;
#16252=CARTESIAN_POINT ( 'NONE',  ( 13.44051670066911619, -5.407089921784859143, -5.015624999385570604 ) ) ;
#16261=CARTESIAN_POINT ( 'NONE',  ( 10.31873187879410914, 0.000000000000000000, -1.996874999385528371 ) ) ;
#16272=ORIENTED_EDGE ( 'NONE', *, *, #19380, .F. ) ;
#16282=CARTESIAN_POINT ( 'NONE',  ( 22.80587116629410360, 3.604726614523238837, -7.078124999385530636 ) ) ;
#16288=CARTESIAN_POINT ( 'NONE',  ( 22.56230152254410726, 7.347880794884117764E-16, -9.112499998771033560 ) ) ;
#16292=CARTESIAN_POINT ( 'NONE',  ( 22.80587116629411426, -3.604726614523238837, -6.309374999385513050 ) ) ;
#16318=CARTESIAN_POINT ( 'NONE',  ( 19.68408634441912142, -5.407089921784861808, -8.146874999385516958 ) ) ;
#16323=CARTESIAN_POINT ( 'NONE',  ( 19.68408634441910721, 5.407089921784857367, -1.640624999385525973 ) ) ;
#16324=EDGE_CURVE ( 'NONE', #29619, #20388, #31090, .T. ) ;
#16330=CARTESIAN_POINT ( 'NONE',  ( 22.56230152254410370, -3.464101615137751278, -2.399999998770968812 ) ) ;
#16333=DIRECTION ( 'NONE',  ( 0.000000000000000000, 0.000000000000000000, 1.000000000000000000 ) ) ;
#16338=CARTESIAN_POINT ( 'NONE',  ( 22.56230152254411436, 3.464101615137759271, -8.287500000000068923 ) ) ;
#16348=CARTESIAN_POINT ( 'NONE',  ( 22.56230152254410370, 7.347880794884117764E-16, -6.862499998771004250 ) ) ;
#16355=CARTESIAN_POINT ( 'NONE',  ( 19.68408634441912142, -5.407089921784861808, -6.796874999385527083 ) ) ;
#16360=CARTESIAN_POINT ( 'NONE',  ( 22.80587116629411426, 7.646167579472024665E-16, -2.221874999385531346 ) ) ;
#16363=( BOUNDED_CURVE ( )  B_SPLINE_CURVE ( 2, ( #25422, #36974, #13489, #11018, #22592, #34138, #25605 ),
 .UNSPECIFIED., .F., .F. ) 
 B_SPLINE_CURVE_WITH_KNOTS ( ( 3, 2, 2, 3 ),
 ( 0.1739130434782631685, 0.1811594202898574590, 0.1884057971014517219, 0.1956521739130460125 ),
 .UNSPECIFIED. ) 
 CURVE ( )  GEOMETRIC_REPRESENTATION_ITEM ( )  RATIONAL_B_SPLINE_CURVE ( ( 0.9999999999999574785, 0.8660254037844813402, 1.000000000000000000, 0.8660254037844387076, 1.000000000000000000, 0.8660254037843919672, 1.000000000000046629 ) ) 
 REPRESENTATION_ITEM ( '' )  );
#16369=FACE_OUTER_BOUND ( 'NONE', #222, .T. ) ;
#16381=CARTESIAN_POINT ( 'NONE',  ( 22.56230152254412147, -3.464101615137755275, -1.612500000000030020 ) ) ;
#16400=CARTESIAN_POINT ( 'NONE',  ( 10.31873187879411269, 0.000000000000000000, -10.04062499938554431 ) ) ;
#16407=VERTEX_POINT ( 'NONE', #968 ) ;
#16423=AXIS2_PLACEMENT_3D ( 'NONE', #5991, #17570, #14717 ) ;
#16437=CARTESIAN_POINT ( 'NONE',  ( 13.44051670066911086, 5.407089921784856479, -6.515624999385543958 ) ) ;
#16447=CARTESIAN_POINT ( 'NONE',  ( 13.44051670066911086, 5.407089921784862696, -1.621874999385541916 ) ) ;
#16475=CARTESIAN_POINT ( 'NONE',  ( 19.56230152254411792, -5.196152422706629359, -7.837499998771035870 ) ) ;
#16479=CARTESIAN_POINT ( 'NONE',  ( 13.44051670066910731, 5.407089921784862696, -7.471874999385508254 ) ) ;
#16495=CARTESIAN_POINT ( 'NONE',  ( 16.56230152254410370, -6.928203230275506996, -6.974999998770984533 ) ) ;
#16507=CARTESIAN_POINT ( 'NONE',  ( 16.56230152254411436, 7.209453229046482114, -9.309374999385525484 ) ) ;
#16511=CARTESIAN_POINT ( 'NONE',  ( 22.80587116629411071, 3.604726614523238837, -0.7781249993855585689 ) ) ;
#16514=CARTESIAN_POINT ( 'NONE',  ( 10.56230152254411081, 0.000000000000000000, -3.037499998771009402 ) ) ;
#16517=CARTESIAN_POINT ( 'NONE',  ( 10.31873187879410558, -3.604726614523244610, -10.05937499938549884 ) ) ;
#16524=AXIS2_PLACEMENT_3D ( 'NONE', #13656, #25209, #7966 ) ;
#16525=CARTESIAN_POINT ( 'NONE',  ( 16.56230152254411436, 6.928203230275514990, -9.562500000000060396 ) ) ;
#16534=CARTESIAN_POINT ( 'NONE',  ( 22.56230152254410370, 0.000000000000000000, -10.00000000000000000 ) ) ;
#16543=CARTESIAN_POINT ( 'NONE',  ( 22.80587116629411781, 3.604726614523243278, -6.684374999385514826 ) ) ;
#16550=CARTESIAN_POINT ( 'NONE',  ( 16.56230152254411792, -7.209453229046482114, -1.884374999385517446 ) ) ;
#16561=DIRECTION ( 'NONE',  ( 0.000000000000000000, 0.000000000000000000, 1.000000000000000000 ) ) ;
#16568=CARTESIAN_POINT ( 'NONE',  ( 19.56230152254412502, -5.196152422706635576, -2.550000000000052225 ) ) ;
#16584=EDGE_CURVE ( 'NONE', #20044, #17872, #11699, .T. ) ;
#16587=CARTESIAN_POINT ( 'NONE',  ( 10.31873187879411091, -3.604726614523240613, -8.653124999385532590 ) ) ;
#16619=CARTESIAN_POINT ( 'NONE',  ( 13.56230152254411792, -5.196152422706638241, -0.8250000000000479172 ) ) ;
#16626=CARTESIAN_POINT ( 'NONE',  ( 10.31873187879410736, 0.000000000000000000, -6.890624999385530636 ) ) ;
#16635=CARTESIAN_POINT ( 'NONE',  ( 13.44051670066911264, 5.407089921784862696, -0.2718749993855240632 ) ) ;
#16637=ORIENTED_EDGE ( 'NONE', *, *, #29749, .T. ) ;
#16641=CARTESIAN_POINT ( 'NONE',  ( 16.56230152254411436, 7.209453229046475009, -1.603124999385524108 ) ) ;
#16647=ORIENTED_EDGE ( 'NONE', *, *, #37122, .T. ) ;
#16662=CARTESIAN_POINT ( 'NONE',  ( 22.56230152254409660, 3.464101615137755275, -7.724999998770988086 ) ) ;
#16666=CARTESIAN_POINT ( 'NONE',  ( 22.80587116629411426, 7.646167579472024665E-16, -7.621874999385519267 ) ) ;
#16671=EDGE_CURVE ( 'NONE', #31762, #31857, #12919, .T. ) ;
#16693=CARTESIAN_POINT ( 'NONE',  ( 22.56230152254411792, 7.347880794884125653E-16, -2.475000000000060485 ) ) ;
#16695=CARTESIAN_POINT ( 'NONE',  ( 16.56230152254411436, 7.209453229046482114, -7.959374999385475213 ) ) ;
#16698=CARTESIAN_POINT ( 'NONE',  ( 19.68408634441910721, -5.407089921784855591, -2.690624999385549110 ) ) ;
#16702=CARTESIAN_POINT ( 'NONE',  ( 13.56230152254410726, 5.196152422706630247, -2.662499998771022724 ) ) ;
#16705=CARTESIAN_POINT ( 'NONE',  ( 22.56230152254411081, 3.464101615137755275, -1.874999998771011311 ) ) ;
#16713=CARTESIAN_POINT ( 'NONE',  ( 10.56230152254411436, -3.464101615137761048, -8.962500000000044764 ) ) ;
#16729=CARTESIAN_POINT ( 'NONE',  ( 10.31873187879410558, 0.000000000000000000, -6.946874999385510563 ) ) ;
#16733=CARTESIAN_POINT ( 'NONE',  ( 16.56230152254412147, -7.209453229046482114, -0.9843749993855260838 ) ) ;
#16738=AXIS2_PLACEMENT_3D ( 'NONE', #1392, #13717, #12966 ) ;
#16739=DIRECTION ( 'NONE',  ( 0.000000000000000000, 0.000000000000000000, 1.000000000000000000 ) ) ;
#16743=DIRECTION ( 'NONE',  ( 1.000000000000000000, 0.000000000000000000, 0.000000000000000000 ) ) ;
#16750=CARTESIAN_POINT ( 'NONE',  ( 13.56230152254411614, -5.196152422706638241, -1.725000000000059819 ) ) ;
#16759=CARTESIAN_POINT ( 'NONE',  ( 10.56230152254410903, 7.347880794884117764E-16, -10.00000000000000000 ) ) ;
#16769=CARTESIAN_POINT ( 'NONE',  ( 16.56230152254411081, 7.209453229046475009, -8.353124999385522997 ) ) ;
#16775=EDGE_LOOP ( 'NONE', ( #32052, #30295, #18614, #28343 ) ) ;
#16776=ORIENTED_EDGE ( 'NONE', *, *, #13301, .F. ) ;
#16779=CARTESIAN_POINT ( 'NONE',  ( 22.56230152254411792, 7.347880794884125653E-16, -0.6750000000000366818 ) ) ;
#16803=EDGE_CURVE ( 'NONE', #23009, #24665, #6616, .T. ) ;
#16807=CARTESIAN_POINT ( 'NONE',  ( 10.31873187879411091, -3.604726614523240613, -7.753124999385540228 ) ) ;
#16808=( BOUNDED_CURVE ( )  B_SPLINE_CURVE ( 2, ( #36793, #10835, #13879, #33958, #36418, #25427, #16348 ),
 .UNSPECIFIED., .F., .F. ) 
 B_SPLINE_CURVE_WITH_KNOTS ( ( 3, 2, 2, 3 ),
 ( 0.6086956521739130821, 0.6159420289855073172, 0.6231884057971015523, 0.6304347826086958984 ),
 .UNSPECIFIED. ) 
 CURVE ( )  GEOMETRIC_REPRESENTATION_ITEM ( )  RATIONAL_B_SPLINE_CURVE ( ( 1.000000000000000000, 0.8660254037844387076, 1.000000000000000000, 0.8660254037844387076, 1.000000000000000000, 0.8660254037844345998, 1.000000000000003997 ) ) 
 REPRESENTATION_ITEM ( '' )  );
#16817=CARTESIAN_POINT ( 'NONE',  ( 19.68408634441911076, 5.407089921784862696, -2.146874999385511629 ) ) ;
#16819=EDGE_LOOP ( 'NONE', ( #31409, #24861, #28522, #16272 ) ) ;
#16823=CARTESIAN_POINT ( 'NONE',  ( 10.31873187879411091, 3.604726614523236616, -1.528124999385498173 ) ) ;
#16832=EDGE_CURVE ( 'NONE', #18251, #9681, #24550, .T. ) ;
#16849=CARTESIAN_POINT ( 'NONE',  ( 14.47852538368266195, 5.725134515572932514, -10.32395279703524871 ) ) ;
#16854=CARTESIAN_POINT ( 'NONE',  ( 10.31873187879410736, 0.000000000000000000, -6.046874999385526195 ) ) ;
#16855=CARTESIAN_POINT ( 'NONE',  ( 10.56230152254410903, 0.000000000000000000, -0.7874999987710074034 ) ) ;
#16877=EDGE_CURVE ( 'NONE', #2209, #23009, #1297, .T. ) ;
#16881=CARTESIAN_POINT ( 'NONE',  ( 13.44051670066910908, 5.407089921784862696, -8.821874999385526550 ) ) ;
#16884=CARTESIAN_POINT ( 'NONE',  ( 13.44051670066911086, 5.407089921784856479, -2.015624999385540406 ) ) ;
#16890=CARTESIAN_POINT ( 'NONE',  ( 13.56230152254410726, 5.196152422706630247, -2.662499998771022724 ) ) ;
#16897=CARTESIAN_POINT ( 'NONE',  ( 16.56230152254411081, 7.209453229046475009, -2.953124999385511096 ) ) ;
#16898=CARTESIAN_POINT ( 'NONE',  ( 10.56230152254410903, 0.000000000000000000, -3.487499998771015353 ) ) ;
#16900=CARTESIAN_POINT ( 'NONE',  ( 19.56230152254411436, -5.196152422706629359, -4.687499998771022192 ) ) ;
#16915=CARTESIAN_POINT ( 'NONE',  ( 13.44051670066911441, -5.407089921784865361, -6.421874999385540406 ) ) ;
#16920=CARTESIAN_POINT ( 'NONE',  ( 19.68408634441911431, 5.407089921784862696, -0.7968749993855217539 ) ) ;
#16936=CARTESIAN_POINT ( 'NONE',  ( 13.56230152254410903, 5.196152422706636465, -3.225000000000033396 ) ) ;
#16954=CARTESIAN_POINT ( 'NONE',  ( 10.31873187879411091, 3.604726614523236616, -10.07812499938551198 ) ) ;
#16968=ADVANCED_FACE ( 'NONE', ( #34858 ), #23129, .F. ) ;
#16989=CARTESIAN_POINT ( 'NONE',  ( 22.80587116629410360, -3.604726614523235284, -6.253124999385533123 ) ) ;
#16997=CARTESIAN_POINT ( 'NONE',  ( 10.31873187879410558, 3.604726614523240613, -2.484374999385500882 ) ) ;
#17003=CARTESIAN_POINT ( 'NONE',  ( 10.31873187879411446, -3.604726614523240613, -2.803124999385555149 ) ) ;
#17007=EDGE_CURVE ( 'NONE', #2700, #10334, #32118, .T. ) ;
#17010=ORIENTED_EDGE ( 'NONE', *, *, #26495, .T. ) ;
#17017=VECTOR ( 'NONE', #24252, 1000.000000000000000 ) ;
#17022=CARTESIAN_POINT ( 'NONE',  ( 22.80587116629411071, 3.604726614523238837, -9.328124999385510208 ) ) ;
#17030=CARTESIAN_POINT ( 'NONE',  ( 10.56230152254411259, 3.464101615137752166, -10.27499999877103853 ) ) ;
#17035=CARTESIAN_POINT ( 'NONE',  ( 10.31873187879410558, 0.000000000000000000, -8.746874999385534366 ) ) ;
#17041=CARTESIAN_POINT ( 'NONE',  ( 16.56230152254410726, 0.000000000000000000, -10.00000000000000000 ) ) ;
#17042=VERTEX_POINT ( 'NONE', #20098 ) ;
#17059=CARTESIAN_POINT ( 'NONE',  ( 19.56230152254412502, -5.196152422706635576, -3.000000000000058176 ) ) ;
#17066=CARTESIAN_POINT ( 'NONE',  ( 10.31873187879410736, 0.000000000000000000, -4.190624999385549998 ) ) ;
#17070=CARTESIAN_POINT ( 'NONE',  ( 10.56230152254410903, 0.000000000000000000, -3.487499998771015353 ) ) ;
#17073=CYLINDRICAL_SURFACE ( 'NONE', #28835, 5.999999999999998224 ) ;
#17081=CARTESIAN_POINT ( 'NONE',  ( 10.31873187879411091, -3.604726614523240613, -2.353124999385527882 ) ) ;
#17082=CARTESIAN_POINT ( 'NONE',  ( 16.56230152254410726, 6.928203230275506996, -8.999999998771013310 ) ) ;
#17092=CARTESIAN_POINT ( 'NONE',  ( 19.56230152254411436, -5.196152422706629359, -8.737499998771019349 ) ) ;
#17096=EDGE_LOOP ( 'NONE', ( #11962, #34188, #35972, #11043 ) ) ;
#17100=CARTESIAN_POINT ( 'NONE',  ( 22.80587116629411781, -3.604726614523238837, -9.459374999385547156 ) ) ;
#17104=CARTESIAN_POINT ( 'NONE',  ( 10.31873187879410736, -3.604726614523244610, -0.6093749993855241964 ) ) ;
#17108=CARTESIAN_POINT ( 'NONE',  ( 22.56230152254410370, 7.347880794884117764E-16, -0.5624999987710044280 ) ) ;
#17109=SHAPE_DEFINITION_REPRESENTATION ( #15014, #201 ) ;
#17122=EDGE_CURVE ( 'NONE', #4455, #18743, #3728, .T. ) ;
#17125=CARTESIAN_POINT ( 'NONE',  ( 19.56230152254412502, -5.196152422706635576, -4.350000000000076028 ) ) ;
#17143=CARTESIAN_POINT ( 'NONE',  ( 22.80587116629411781, 7.646167579472024665E-16, -0.4218749993855352987 ) ) ;
#17177=CARTESIAN_POINT ( 'NONE',  ( 16.56230152254411081, 7.209453229046475009, -6.103124999385545202 ) ) ;
#17186=EDGE_LOOP ( 'NONE', ( #2764, #37170, #8575, #32249 ) ) ;
#17190=CARTESIAN_POINT ( 'NONE',  ( 13.44051670066911086, 5.407089921784856479, -4.715624999385548577 ) ) ;
#17197=ORIENTED_EDGE ( 'NONE', *, *, #36630, .F. ) ;
#17215=AXIS2_PLACEMENT_3D ( 'NONE', #16047, #4651, #19645 ) ;
#17223=CARTESIAN_POINT ( 'NONE',  ( 13.44051670066911441, -5.407089921784865361, -9.121874999385520155 ) ) ;
#17226=FACE_OUTER_BOUND ( 'NONE', #12720, .T. ) ;
#17250=CARTESIAN_POINT ( 'NONE',  ( 10.31873187879411091, -3.604726614523240613, -1.903124999385531924 ) ) ;
#17251=( BOUNDED_CURVE ( )  B_SPLINE_CURVE ( 2, ( #22492, #11106, #37244, #22680, #16619, #28526, #19841 ),
 .UNSPECIFIED., .F., .F. ) 
 B_SPLINE_CURVE_WITH_KNOTS ( ( 3, 2, 2, 3 ),
 ( 0.06521739130434593690, 0.07246376811594026912, 0.07971014492753460134, 0.08695652173912893357 ),
 .UNSPECIFIED. ) 
 CURVE ( )  GEOMETRIC_REPRESENTATION_ITEM ( )  RATIONAL_B_SPLINE_CURVE ( ( 1.000000000000034861, 0.8660254037844038466, 1.000000000000000000, 0.8660254037844387076, 1.000000000000000000, 0.8660254037844664632, 0.9999999999999722444 ) ) 
 REPRESENTATION_ITEM ( '' )  );
#17252=EDGE_CURVE ( 'NONE', #31128, #7808, #21230, .T. ) ;
#17257=CARTESIAN_POINT ( 'NONE',  ( 13.56230152254410548, 5.196152422706630247, -4.462499998771018994 ) ) ;
#17284=CARTESIAN_POINT ( 'NONE',  ( 10.31873187879410736, 3.604726614523240613, -8.334374999385541827 ) ) ;
#17288=CARTESIAN_POINT ( 'NONE',  ( 22.80587116629412492, 3.604726614523243278, -3.534374999385544669 ) ) ;
#17302=CARTESIAN_POINT ( 'NONE',  ( 22.56230152254377330, 3.464101615137958667, -1.537500000000063816 ) ) ;
#17308=CARTESIAN_POINT ( 'NONE',  ( 19.56230152254412502, 5.196152422706637353, -5.100000000000049383 ) ) ;
#17312=CARTESIAN_POINT ( 'NONE',  ( 22.56230152254426358, -3.464101615137659351, -6.449999998771025922 ) ) ;
#17314=CARTESIAN_POINT ( 'NONE',  ( 16.56230152254410726, 0.000000000000000000, -10.00000000000000000 ) ) ;
#17326=CARTESIAN_POINT ( 'NONE',  ( 10.31873187879410736, 0.000000000000000000, -1.096874999385516469 ) ) ;
#17332=ORIENTED_EDGE ( 'NONE', *, *, #19875, .T. ) ;
#17351=CARTESIAN_POINT ( 'NONE',  ( 16.56230152254411081, -6.928203230275514990, -5.287500000000021849 ) ) ;
#17363=CARTESIAN_POINT ( 'NONE',  ( 13.44051670066911619, -5.407089921784859143, -9.965624999385552130 ) ) ;
#17364=DIRECTION ( 'NONE',  ( 0.000000000000000000, 0.000000000000000000, 1.000000000000000000 ) ) ;
#17376=CARTESIAN_POINT ( 'NONE',  ( 22.80587116629410716, 7.646167579472015790E-16, -3.515624999385541294 ) ) ;
#17379=ADVANCED_FACE ( 'NONE', ( #15151 ), #3769, .F. ) ;
#17391=CYLINDRICAL_SURFACE ( 'NONE', #21231, 5.999999999999998224 ) ;
#17405=CARTESIAN_POINT ( 'NONE',  ( 13.56230152254411436, -5.196152422706632912, -10.16249999877102894 ) ) ;
#17409=CARTESIAN_POINT ( 'NONE',  ( 16.56230152254411436, -7.209453229046482114, -8.634374999385517668 ) ) ;
#17423=CARTESIAN_POINT ( 'NONE',  ( 10.56230152254410548, 0.000000000000000000, -9.000000000000035527 ) ) ;
#17428=EDGE_LOOP ( 'NONE', ( #4360, #33315, #8221, #10746 ) ) ;
#17438=CARTESIAN_POINT ( 'NONE',  ( 16.56230152254411436, 7.209453229046475009, -3.853124999385534544 ) ) ;
#17443=CARTESIAN_POINT ( 'NONE',  ( 13.56230152254411614, -5.196152422706632912, -4.762499998771041021 ) ) ;
#17447=AXIS2_PLACEMENT_3D ( 'NONE', #19392, #30935, #33957 ) ;
#17456=ORIENTED_EDGE ( 'NONE', *, *, #5436, .F. ) ;
#17472=CARTESIAN_POINT ( 'NONE',  ( 19.68408634441910721, 5.407089921784862696, -8.896874999385516958 ) ) ;
#17475=( BOUNDED_CURVE ( )  B_SPLINE_CURVE ( 2, ( #21251, #29570, #14984, #3978, #12889, #9674, #27291 ),
 .UNSPECIFIED., .F., .F. ) 
 B_SPLINE_CURVE_WITH_KNOTS ( ( 3, 2, 2, 3 ),
 ( 0.4565217391304354777, 0.4637681159420298238, 0.4710144927536240589, 0.4782608695652184050 ),
 .UNSPECIFIED. ) 
 CURVE ( )  GEOMETRIC_REPRESENTATION_ITEM ( )  RATIONAL_B_SPLINE_CURVE ( ( 0.9999999999999866773, 0.8660254037844520303, 1.000000000000000000, 0.8660254037844387076, 1.000000000000000000, 0.8660254037844202779, 1.000000000000018430 ) ) 
 REPRESENTATION_ITEM ( '' )  );
#17478=CARTESIAN_POINT ( 'NONE',  ( 10.31873187879410736, 0.000000000000000000, -3.796874999385524418 ) ) ;
#17494=CARTESIAN_POINT ( 'NONE',  ( 22.56230152254412147, -3.464101615137755275, -5.212500000000060751 ) ) ;
#17502=CARTESIAN_POINT ( 'NONE',  ( 16.56230152254410726, 0.000000000000000000, 10.00000000000000000 ) ) ;
#17503=DIRECTION ( 'NONE',  ( 1.000000000000000000, 0.000000000000000000, 0.000000000000000000 ) ) ;
#17514=CARTESIAN_POINT ( 'NONE',  ( 22.80587116629411781, 7.646167579472024665E-16, -0.8718749993855412495 ) ) ;
#17520=ORIENTED_EDGE ( 'NONE', *, *, #20778, .F. ) ;
#17523=DIRECTION ( 'NONE',  ( 1.000000000000000000, 0.000000000000000000, 0.000000000000000000 ) ) ;
#17541=CARTESIAN_POINT ( 'NONE',  ( 16.56230152254410726, 0.000000000000000000, -10.00000000000000000 ) ) ;
#17549=CARTESIAN_POINT ( 'NONE',  ( 15.47812198514404258, 6.148716665048038266, -10.14010144556222315 ) ) ;
#17552=CARTESIAN_POINT ( 'NONE',  ( 10.39871248152193672, 0.5029693937725558950, -9.999999999999998224 ) ) ;
#17559=ORIENTED_EDGE ( 'NONE', *, *, #28353, .T. ) ;
#17563=CARTESIAN_POINT ( 'NONE',  ( 19.68408634441910365, 5.407089921784857367, -4.340624999385561900 ) ) ;
#17566=CYLINDRICAL_SURFACE ( 'NONE', #313, 5.999999999999998224 ) ;
#17570=DIRECTION ( 'NONE',  ( 0.000000000000000000, 0.000000000000000000, 1.000000000000000000 ) ) ;
#17572=DIRECTION ( 'NONE',  ( 1.000000000000000000, 0.000000000000000000, 0.000000000000000000 ) ) ;
#17580=CARTESIAN_POINT ( 'NONE',  ( 22.56230152254410370, 7.347880794884117764E-16, -5.062499998771007981 ) ) ;
#17584=( BOUNDED_CURVE ( )  B_SPLINE_CURVE ( 2, ( #34085, #14189, #20254, #14373, #5453, #22913, #14002 ),
 .UNSPECIFIED., .F., .F. ) 
 B_SPLINE_CURVE_WITH_KNOTS ( ( 3, 2, 2, 3 ),
 ( 0.000000000000000000, 0.007246376811594273243, 0.01449275362318854649, 0.02173913043478281973 ),
 .UNSPECIFIED. ) 
 CURVE ( )  GEOMETRIC_REPRESENTATION_ITEM ( )  RATIONAL_B_SPLINE_CURVE ( ( 1.000000000000000000, 0.8660254037844387076, 1.000000000000000000, 0.8660254037844387076, 1.000000000000000000, 0.8660254037844348218, 1.000000000000003997 ) ) 
 REPRESENTATION_ITEM ( '' )  );
#17598=CARTESIAN_POINT ( 'NONE',  ( 10.31873187879410381, -3.604726614523244610, -7.809374999385488181 ) ) ;
#17599=VECTOR ( 'NONE', #35738, 1000.000000000000000 ) ;
#17614=CARTESIAN_POINT ( 'NONE',  ( 22.56230152254412147, 7.347880794884125653E-16, -9.225000000000010303 ) ) ;
#17620=ORIENTED_EDGE ( 'NONE', *, *, #4155, .T. ) ;
#17629=CARTESIAN_POINT ( 'NONE',  ( 19.68408634441910721, 5.407089921784857367, -6.140624999385558169 ) ) ;
#17634=CARTESIAN_POINT ( 'NONE',  ( 19.56230152254410370, 5.196152422706631135, -3.187499998770992882 ) ) ;
#17645=DIRECTION ( 'NONE',  ( 0.000000000000000000, 0.000000000000000000, 1.000000000000000000 ) ) ;
#17647=EDGE_LOOP ( 'NONE', ( #31408, #27635, #30583 ) ) ;
#17653=CARTESIAN_POINT ( 'NONE',  ( 16.56230152254411081, -6.928203230275506996, -8.774999998770997678 ) ) ;
#17658=ORIENTED_EDGE ( 'NONE', *, *, #25713, .T. ) ;
#17661=CARTESIAN_POINT ( 'NONE',  ( 10.31873187879410558, -3.604726614523244610, -9.159374999385507365 ) ) ;
#17666=CARTESIAN_POINT ( 'NONE',  ( 10.31873187879410381, -3.604726614523244610, -4.209374999385490312 ) ) ;
#17683=CARTESIAN_POINT ( 'NONE',  ( 22.56230152254412147, 7.347880794884125653E-16, -4.275000000000028777 ) ) ;
#17699=CARTESIAN_POINT ( 'NONE',  ( 19.68408634441912142, -5.407089921784861808, -2.296874999385551064 ) ) ;
#17710=ADVANCED_FACE ( 'NONE', ( #34800, #20416 ), #31959, .F. ) ;
#17724=CARTESIAN_POINT ( 'NONE',  ( 14.47852626837769563, 5.725135026351853007, -9.986452809322953428 ) ) ;
#17732=CARTESIAN_POINT ( 'NONE',  ( 22.80587116629410716, 7.646167579472015790E-16, -8.465624999385523708 ) ) ;
#17746=CARTESIAN_POINT ( 'NONE',  ( 22.80587116629410360, -3.604726614523235284, -4.003124999385554439 ) ) ;
#17781=CARTESIAN_POINT ( 'NONE',  ( 19.68408634441910365, 5.407089921784857367, -2.990624999385543603 ) ) ;
#17783=CARTESIAN_POINT ( 'NONE',  ( 16.56230152254410726, 0.000000000000000000, 10.00000000000000000 ) ) ;
#17801=ORIENTED_EDGE ( 'NONE', *, *, #15976, .F. ) ;
#17806=( BOUNDED_CURVE ( )  B_SPLINE_CURVE ( 2, ( #15351, #9846, #26905, #32778, #15540, #7017, #14788 ),
 .UNSPECIFIED., .F., .F. ) 
 B_SPLINE_CURVE_WITH_KNOTS ( ( 3, 2, 2, 3 ),
 ( 0.2608695652173921298, 0.2681159420289864204, 0.2753623188405806554, 0.2826086956521748905 ),
 .UNSPECIFIED. ) 
 CURVE ( )  GEOMETRIC_REPRESENTATION_ITEM ( )  RATIONAL_B_SPLINE_CURVE ( ( 0.9999999999999845679, 0.8660254037844541397, 1.000000000000000000, 0.8660254037844387076, 1.000000000000000000, 0.8660254037844202779, 1.000000000000018430 ) ) 
 REPRESENTATION_ITEM ( '' )  );
#17816=CARTESIAN_POINT ( 'NONE',  ( 13.44051670066911086, 5.407089921784856479, -6.515624999385543958 ) ) ;
#17823=CARTESIAN_POINT ( 'NONE',  ( 19.56230152254410726, 5.196152422706631135, -5.887499998771001053 ) ) ;
#17845=CARTESIAN_POINT ( 'NONE',  ( 13.44051670066911441, 5.407089921784856479, -0.6656249993855500868 ) ) ;
#17848=VERTEX_POINT ( 'NONE', #9405 ) ;
#17854=ORIENTED_EDGE ( 'NONE', *, *, #36911, .F. ) ;
#17855=CARTESIAN_POINT ( 'NONE',  ( 16.56230152254411436, -7.209453229046482114, -3.234374999385536409 ) ) ;
#17871=CARTESIAN_POINT ( 'NONE',  ( 10.56230152254411259, -3.464101615137761048, -7.612500000000058442 ) ) ;
#17872=VERTEX_POINT ( 'NONE', #18514 ) ;
#17889=CARTESIAN_POINT ( 'NONE',  ( 22.80587116629411781, 3.604726614523243278, -0.8343749993855380520 ) ) ;
#17898=CARTESIAN_POINT ( 'NONE',  ( 19.56230152254410726, 5.196152422706631135, -6.337499998771006560 ) ) ;
#17912=VECTOR ( 'NONE', #34325, 1000.000000000000000 ) ;
#17913=ORIENTED_EDGE ( 'NONE', *, *, #19662, .T. ) ;
#17921=CARTESIAN_POINT ( 'NONE',  ( 16.56230152254410726, 7.209453229046475009, -9.253124999385514471 ) ) ;
#17930=ORIENTED_EDGE ( 'NONE', *, *, #18990, .F. ) ;
#17934=CARTESIAN_POINT ( 'NONE',  ( 16.56230152254410726, 7.209453229046475009, -5.203124999385489780 ) ) ;
#17942=CARTESIAN_POINT ( 'NONE',  ( 22.56230152254361698, -3.464101615138046597, -2.962500000000023892 ) ) ;
#17964=ORIENTED_EDGE ( 'NONE', *, *, #12440, .F. ) ;
#17967=DIRECTION ( 'NONE',  ( 0.000000000000000000, 0.000000000000000000, 1.000000000000000000 ) ) ;
#17971=CARTESIAN_POINT ( 'NONE',  ( 16.56230152254411436, 7.209453229046475009, -1.153124999385528371 ) ) ;
#17982=EDGE_CURVE ( 'NONE', #36330, #31630, #4271, .T. ) ;
#17994=AXIS2_PLACEMENT_3D ( 'NONE', #23443, #5437, #34996 ) ;
#18003=CARTESIAN_POINT ( 'NONE',  ( 16.56230152254411081, -7.209453229046475009, -5.428124999385503635 ) ) ;
#18008=CARTESIAN_POINT ( 'NONE',  ( 10.56230152254410903, 0.000000000000000000, -6.187499998771023080 ) ) ;
#18013=CARTESIAN_POINT ( 'NONE',  ( 10.31873187879410736, 0.000000000000000000, -2.896874999385512517 ) ) ;
#18031=FACE_OUTER_BOUND ( 'NONE', #13507, .T. ) ;
#18042=CARTESIAN_POINT ( 'NONE',  ( 13.44051670066911441, -5.407089921784865361, -4.171874999385538629 ) ) ;
#18047=( BOUNDED_CURVE ( )  B_SPLINE_CURVE ( 2, ( #13280, #37131, #7409, #25019, #30902, #31273, #16693 ),
 .UNSPECIFIED., .F., .F. ) 
 B_SPLINE_CURVE_WITH_KNOTS ( ( 3, 2, 2, 3 ),
 ( 0.2173913043478263585, 0.2246376811594206213, 0.2318840579710148841, 0.2391304347826091470 ),
 .UNSPECIFIED. ) 
 CURVE ( )  GEOMETRIC_REPRESENTATION_ITEM ( )  RATIONAL_B_SPLINE_CURVE ( ( 0.9999999999999948930, 0.8660254037844438146, 1.000000000000000000, 0.8660254037844387076, 1.000000000000000000, 0.8660254037844304920, 1.000000000000008216 ) ) 
 REPRESENTATION_ITEM ( '' )  );
#18062=CARTESIAN_POINT ( 'NONE',  ( 19.56230152254412502, 5.196152422706637353, -6.000000000000060396 ) ) ;
#18071=CARTESIAN_POINT ( 'NONE',  ( 16.25485273795005625, -6.235291796180306712, -10.00000000000000000 ) ) ;
#18081=CARTESIAN_POINT ( 'NONE',  ( 10.31873187879410736, 0.000000000000000000, -3.346874999385518468 ) ) ;
#18094=CARTESIAN_POINT ( 'NONE',  ( 22.80587116629410716, 3.604726614523238837, -1.678124999385517846 ) ) ;
#18102=CARTESIAN_POINT ( 'NONE',  ( 10.56230152254438970, 3.464101615137910706, -0.8249999987710033844 ) ) ;
#18112=CARTESIAN_POINT ( 'NONE',  ( 10.31873187879411091, -3.604726614523240613, -9.103124999385528326 ) ) ;
#18124=CARTESIAN_POINT ( 'NONE',  ( 10.31873187879411269, -3.604726614523240613, -6.403124999385521043 ) ) ;
#18133=CARTESIAN_POINT ( 'NONE',  ( 10.56230152254472188, -3.464101615138113210, -3.112499999999997158 ) ) ;
#18149=EDGE_CURVE ( 'NONE', #12997, #2700, #29792, .T. ) ;
#18160=CARTESIAN_POINT ( 'NONE',  ( 19.68408634441910721, -5.407089921784855591, -2.240624999385543159 ) ) ;
#18165=CARTESIAN_POINT ( 'NONE',  ( 22.56230152254411792, 7.347880794884125653E-16, -5.175000000000040679 ) ) ;
#18166=CARTESIAN_POINT ( 'NONE',  ( 16.56230152254410370, -6.928203230275506996, -7.874999998770976006 ) ) ;
#18180=EDGE_LOOP ( 'NONE', ( #26341, #19730, #4967, #8426 ) ) ;
#18188=CARTESIAN_POINT ( 'NONE',  ( 10.56230152254410903, 7.347880794884117764E-16, -10.00000000000000000 ) ) ;
#18190=CARTESIAN_POINT ( 'NONE',  ( 10.31873187879411091, 0.000000000000000000, -5.090624999385534366 ) ) ;
#18198=CARTESIAN_POINT ( 'NONE',  ( 10.56230152254411259, 3.464101615137752166, -6.224999998771012955 ) ) ;
#18203=CARTESIAN_POINT ( 'NONE',  ( 22.80587116629412492, 3.604726614523243278, -3.534374999385544669 ) ) ;
#18205=DIRECTION ( 'NONE',  ( 0.000000000000000000, 0.000000000000000000, 1.000000000000000000 ) ) ;
#18232=CARTESIAN_POINT ( 'NONE',  ( 10.31873187879410558, 0.000000000000000000, -6.496874999385504168 ) ) ;
#18247=( BOUNDED_CURVE ( )  B_SPLINE_CURVE ( 2, ( #30060, #33094, #27400, #26839, #9968, #18894, #7139 ),
 .UNSPECIFIED., .F., .F. ) 
 B_SPLINE_CURVE_WITH_KNOTS ( ( 3, 2, 2, 3 ),
 ( 0.3260869565217406896, 0.3333333333333340920, 0.3405797101449276054, 0.3478260869565210078 ),
 .UNSPECIFIED. ) 
 CURVE ( )  GEOMETRIC_REPRESENTATION_ITEM ( )  RATIONAL_B_SPLINE_CURVE ( ( 0.9999999999999712452, 0.8660254037844674624, 1.000000000000000000, 0.8660254037844387076, 1.000000000000000000, 0.8660254037844520303, 0.9999999999999866773 ) ) 
 REPRESENTATION_ITEM ( '' )  );
#18250=CARTESIAN_POINT ( 'NONE',  ( 10.56230152254411259, 3.464101615137757051, -7.237500000000056666 ) ) ;
#18251=VERTEX_POINT ( 'NONE', #26947 ) ;
#18266=CARTESIAN_POINT ( 'NONE',  ( 22.80587116629412137, 7.646167579472024665E-16, -4.471874999385533123 ) ) ;
#18278=CARTESIAN_POINT ( 'NONE',  ( 10.31873187879411091, 3.604726614523236616, -1.528124999385497729 ) ) ;
#18290=VECTOR ( 'NONE', #17364, 1000.000000000000000 ) ;
#18297=B_SPLINE_CURVE_WITH_KNOTS ( 'NONE', 3,
 ( #34109, #10990, #33371, #8161, #4741, #14028, #33559, #22006 ),
 .UNSPECIFIED., .F., .F.,
 ( 4, 2, 2, 4 ),
 ( 0.000000000000000000, 0.001245943103805707310, 0.002491886207611414619, 0.004983772415222829238 ),
 .UNSPECIFIED. ) ;
#18300=CARTESIAN_POINT ( 'NONE',  ( 19.56230152254411081, -5.196152422706629359, -0.6374999987710516791 ) ) ;
#18313=CARTESIAN_POINT ( 'NONE',  ( 19.68408634441910365, -5.407089921784855591, -6.290624999385540761 ) ) ;
#18346=CARTESIAN_POINT ( 'NONE',  ( 10.31873187879411091, 3.604726614523236616, -3.328124999385545291 ) ) ;
#18348=FACE_OUTER_BOUND ( 'NONE', #37258, .T. ) ;
#18377=CARTESIAN_POINT ( 'NONE',  ( 10.31873187879410914, 0.000000000000000000, -5.540624999385540761 ) ) ;
#18382=DIRECTION ( 'NONE',  ( 0.000000000000000000, 0.000000000000000000, 1.000000000000000000 ) ) ;
#18384=CARTESIAN_POINT ( 'NONE',  ( 13.56230152254410370, 5.196152422706630247, -5.362499998771003362 ) ) ;
#18388=CARTESIAN_POINT ( 'NONE',  ( 13.44051670066910731, 5.407089921784862696, -5.221874999385534011 ) ) ;
#18396=CYLINDRICAL_SURFACE ( 'NONE', #31782, 5.999999999999998224 ) ;
#18401=DIRECTION ( 'NONE',  ( 0.2588190451025212391, 3.169619151431769872E-17, -0.9659258262890682012 ) ) ;
#18422=CARTESIAN_POINT ( 'NONE',  ( 10.31873187879410736, -3.604726614523244610, -6.459374999385468996 ) ) ;
#18431=CARTESIAN_POINT ( 'NONE',  ( 10.56230152254209642, -3.464101615136592649, -9.749999998771011533 ) ) ;
#18438=AXIS2_PLACEMENT_3D ( 'NONE', #22264, #31521, #5181 ) ;
#18443=CARTESIAN_POINT ( 'NONE',  ( 10.56230152254410726, 0.000000000000000000, -7.650000000000045652 ) ) ;
#18445=ORIENTED_EDGE ( 'NONE', *, *, #16584, .T. ) ;
#18453=CARTESIAN_POINT ( 'NONE',  ( 22.56230152254476451, 3.464101615137376022, -1.424999998770992038 ) ) ;
#18462=CARTESIAN_POINT ( 'NONE',  ( 16.56230152254411436, -7.209453229046482114, -3.684374999385500615 ) ) ;
#18471=ADVANCED_FACE ( 'NONE', ( #34128 ), #33579, .F. ) ;
#18481=CARTESIAN_POINT ( 'NONE',  ( 13.56230152254410548, 5.196152422706636465, -7.275000000000058975 ) ) ;
#18487=CARTESIAN_POINT ( 'NONE',  ( 22.56230152254411792, 7.347880794884125653E-16, -0.2250000000000584865 ) ) ;
#18506=CARTESIAN_POINT ( 'NONE',  ( 19.68408634441910721, -5.407089921784855591, -6.740624999385547156 ) ) ;
#18514=CARTESIAN_POINT ( 'NONE',  ( 10.56230152254410903, 0.000000000000000000, -9.787499998771043153 ) ) ;
#18531=LINE ( 'NONE', #27409, #13711 ) ;
#18541=( BOUNDED_CURVE ( )  B_SPLINE_CURVE ( 2, ( #13913, #17312, #14648, #14094, #25831, #37378, #22634 ),
 .UNSPECIFIED., .F., .F. ) 
 B_SPLINE_CURVE_WITH_KNOTS ( ( 3, 2, 2, 3 ),
 ( 0.5869565217391301548, 0.5942028985507243899, 0.6014492753623187360, 0.6086956521739130821 ),
 .UNSPECIFIED. ) 
 CURVE ( )  GEOMETRIC_REPRESENTATION_ITEM ( )  RATIONAL_B_SPLINE_CURVE ( ( 1.000000000000006217, 0.8660254037844326014, 1.000000000000000000, 0.8660254037844387076, 1.000000000000000000, 0.8660254037844387076, 1.000000000000000000 ) ) 
 REPRESENTATION_ITEM ( '' )  );
#18543=CARTESIAN_POINT ( 'NONE',  ( 19.68408634441910365, -5.407089921784855591, -5.390624999385557281 ) ) ;
#18548=FACE_OUTER_BOUND ( 'NONE', #4308, .T. ) ;
#18553=CARTESIAN_POINT ( 'NONE',  ( 16.56230152254411436, 6.928203230275514990, -1.912500000000037836 ) ) ;
#18566=VERTEX_POINT ( 'NONE', #31472 ) ;
#18574=CARTESIAN_POINT ( 'NONE',  ( 15.26155779561005232, -6.106572496351636126, -10.00000000000000000 ) ) ;
#18576=CARTESIAN_POINT ( 'NONE',  ( 10.31873187879411091, 0.000000000000000000, -7.340624999385508609 ) ) ;
#18578=CARTESIAN_POINT ( 'NONE',  ( 22.56230152254410370, 7.347880794884117764E-16, -0.5624999987710044280 ) ) ;
#18581=CARTESIAN_POINT ( 'NONE',  ( 13.56230152254410548, 5.196152422706630247, -6.712499998771020771 ) ) ;
#18584=CARTESIAN_POINT ( 'NONE',  ( 19.68408634441910721, 5.407089921784862696, -3.046874999385523530 ) ) ;
#18589=FACE_OUTER_BOUND ( 'NONE', #24828, .T. ) ;
#18591=CARTESIAN_POINT ( 'NONE',  ( 22.56230152254412502, 7.347880794884125653E-16, -3.375000000000044409 ) ) ;
#18596=VECTOR ( 'NONE', #35790, 1000.000000000000000 ) ;
#18602=CARTESIAN_POINT ( 'NONE',  ( 13.44051670066910908, -5.407089921784859143, -0.5156249993855110958 ) ) ;
#18614=ORIENTED_EDGE ( 'NONE', *, *, #31562, .F. ) ;
#18615=CARTESIAN_POINT ( 'NONE',  ( 19.68408634441911431, -5.407089921784861808, -5.446874999385537208 ) ) ;
#18622=SURFACE_STYLE_FILL_AREA ( #24846 ) ;
#18636=CARTESIAN_POINT ( 'NONE',  ( 16.56230152254411436, -6.928203230275514990, -7.537500000000000533 ) ) ;
#18645=CARTESIAN_POINT ( 'NONE',  ( 21.97516523924395315, -2.816244198902225992, -10.00000000000000178 ) ) ;
#18652=CARTESIAN_POINT ( 'NONE',  ( 10.31873187879411091, -3.604726614523244610, -4.659374999385518024 ) ) ;
#18656=ADVANCED_FACE ( 'NONE', ( #14414 ), #11752, .F. ) ;
#18670=CARTESIAN_POINT ( 'NONE',  ( 10.56230152254410903, 0.000000000000000000, -0.7874999987710074034 ) ) ;
#18676=CARTESIAN_POINT ( 'NONE',  ( 13.56230152254411436, -5.196152422706638241, -0.3750000000000419664 ) ) ;
#18695=CARTESIAN_POINT ( 'NONE',  ( 10.31873187879411091, 3.604726614523236616, -7.378124999385539340 ) ) ;
#18712=EDGE_CURVE ( 'NONE', #25502, #27686, #14602, .T. ) ;
#18728=( BOUNDED_CURVE ( )  B_SPLINE_CURVE ( 2, ( #34132, #20110, #8544, #17082, #37334, #22771, #36970 ),
 .UNSPECIFIED., .F., .F. ) 
 B_SPLINE_CURVE_WITH_KNOTS ( ( 3, 2, 2, 3 ),
 ( 0.8260869565217394683, 0.8333333333333347026, 0.8405797101449297148, 0.8478260869565249491 ),
 .UNSPECIFIED. ) 
 CURVE ( )  GEOMETRIC_REPRESENTATION_ITEM ( )  RATIONAL_B_SPLINE_CURVE ( ( 0.9999999999999938938, 0.8660254037844448138, 1.000000000000000000, 0.8660254037844387076, 1.000000000000000000, 0.8660254037843791997, 1.000000000000059508 ) ) 
 REPRESENTATION_ITEM ( '' )  );
#18732=CARTESIAN_POINT ( 'NONE',  ( 10.31873187879410736, 0.000000000000000000, -4.190624999385549998 ) ) ;
#18736=CARTESIAN_POINT ( 'NONE',  ( 13.44051670066910908, 5.407089921784862696, -9.721874999385510918 ) ) ;
#18743=VERTEX_POINT ( 'NONE', #5319 ) ;
#18752=VERTEX_POINT ( 'NONE', #28434 ) ;
#18764=CARTESIAN_POINT ( 'NONE',  ( 10.31873187879410914, 0.000000000000000000, -8.240624999385548932 ) ) ;
#18771=CARTESIAN_POINT ( 'NONE',  ( 19.56230152254411436, -5.196152422706629359, -8.737499998771019349 ) ) ;
#18776=CARTESIAN_POINT ( 'NONE',  ( 10.31873187879411091, -3.604726614523244610, -3.759374999385526106 ) ) ;
#18777=CARTESIAN_POINT ( 'NONE',  ( 16.56230152254411792, -6.928203230275514990, -1.687500000000023981 ) ) ;
#18780=DIRECTION ( 'NONE',  ( 1.000000000000000000, 0.000000000000000000, 0.000000000000000000 ) ) ;
#18784=ORIENTED_EDGE ( 'NONE', *, *, #3203, .F. ) ;
#18789=FACE_OUTER_BOUND ( 'NONE', #14519, .T. ) ;
#18791=CARTESIAN_POINT ( 'NONE',  ( 19.68408634441910721, -5.407089921784855591, -2.240624999385543159 ) ) ;
#18803=CARTESIAN_POINT ( 'NONE',  ( 16.56230152254411436, 7.209453229046482114, -6.159374999385524241 ) ) ;
#18815=CARTESIAN_POINT ( 'NONE',  ( 13.56230152254411436, -5.196152422706632912, -2.062499998771005760 ) ) ;
#18822=CARTESIAN_POINT ( 'NONE',  ( 10.31873187879411091, -3.604726614523240613, -0.5531249993855127389 ) ) ;
#18838=CARTESIAN_POINT ( 'NONE',  ( 13.44051670066911441, -5.407089921784865361, -4.171874999385538629 ) ) ;
#18860=CARTESIAN_POINT ( 'NONE',  ( 22.56230152254412147, 3.464101615137759271, -0.6375000000000446976 ) ) ;
#18866=CARTESIAN_POINT ( 'NONE',  ( 10.56230152254410903, 0.000000000000000000, -8.437499998771025744 ) ) ;
#18877=CARTESIAN_POINT ( 'NONE',  ( 22.80587116629410360, 7.646167579472015790E-16, -8.015624999385517313 ) ) ;
#18879=LINE ( 'NONE', #35912, #10525 ) ;
#18881=EDGE_CURVE ( 'NONE', #2700, #36053, #23613, .T. ) ;
#18885=EDGE_LOOP ( 'NONE', ( #12989, #36475 ) ) ;
#18888=CARTESIAN_POINT ( 'NONE',  ( 10.56230152254463661, -3.464101615138067469, -9.412500000000033396 ) ) ;
#18894=CARTESIAN_POINT ( 'NONE',  ( 10.56230152254446075, -3.464101615137956003, -3.899999998771003895 ) ) ;
#18917=CARTESIAN_POINT ( 'NONE',  ( 16.56230152254410726, -7.209453229046475009, -3.178124999385525395 ) ) ;
#18921=CARTESIAN_POINT ( 'NONE',  ( 17.60716167209216110, -6.606202940439405147, -9.971823764164746251 ) ) ;
#18926=CARTESIAN_POINT ( 'NONE',  ( 10.31873187879411091, -3.604726614523244610, -1.059374999385519933 ) ) ;
#18927=EDGE_LOOP ( 'NONE', ( #26593, #19817, #25205, #27677 ) ) ;
#18946=CARTESIAN_POINT ( 'NONE',  ( 19.68408634441910721, 5.407089921784857367, -7.490624999385548044 ) ) ;
#18952=CARTESIAN_POINT ( 'NONE',  ( 13.56230152254411614, -5.196152422706632912, -7.462499998771049192 ) ) ;
#18955=CARTESIAN_POINT ( 'NONE',  ( 10.31873187879411091, 3.604726614523240613, -6.984374999385522642 ) ) ;
#18976=FACE_OUTER_BOUND ( 'NONE', #11913, .T. ) ;
#18980=CARTESIAN_POINT ( 'NONE',  ( 22.56230152254411792, 7.347880794884125653E-16, -0.2250000000000584865 ) ) ;
#18982=ORIENTED_EDGE ( 'NONE', *, *, #35212, .F. ) ;
#18983=CARTESIAN_POINT ( 'NONE',  ( 13.44051670066911264, -5.407089921784865361, -5.521874999385528504 ) ) ;
#18988=CARTESIAN_POINT ( 'NONE',  ( 16.56230152254411081, 7.209453229046475009, -0.7031249993855005487 ) ) ;
#18990=EDGE_CURVE ( 'NONE', #29181, #6605, #26524, .T. ) ;
#18993=CARTESIAN_POINT ( 'NONE',  ( 22.56230152254410015, 7.347880794884117764E-16, -7.312499998771010645 ) ) ;
#18996=CARTESIAN_POINT ( 'NONE',  ( 22.56230152254411436, -3.464101615137751278, -1.499999998770977561 ) ) ;
#18999=CARTESIAN_POINT ( 'NONE',  ( 19.56230152254412502, -5.196152422706635576, -8.850000000000052935 ) ) ;
#19004=CARTESIAN_POINT ( 'NONE',  ( 16.56230152254411436, -6.928203230275514990, -9.337500000000014566 ) ) ;
#19006=CARTESIAN_POINT ( 'NONE',  ( 22.56230152254463306, -3.464101615137464840, -3.412500000000038725 ) ) ;
#19022=CARTESIAN_POINT ( 'NONE',  ( 16.56230152254411081, -7.209453229046482114, -6.834374999385502747 ) ) ;
#19027=APPLICATION_CONTEXT ( 'automotive_design' ) ;
#19043=CARTESIAN_POINT ( 'NONE',  ( 19.56230152254411792, -5.196152422706635576, -6.150000000000044764 ) ) ;
#19049=CARTESIAN_POINT ( 'NONE',  ( 22.56230152254411792, 7.347880794884125653E-16, -2.025000000000027001 ) ) ;
#19065=CARTESIAN_POINT ( 'NONE',  ( 19.68408634441910721, 5.407089921784857367, -8.840624999385537919 ) ) ;
#19067=LINE ( 'NONE', #2542, #29257 ) ;
#19069=ORIENTED_EDGE ( 'NONE', *, *, #17007, .F. ) ;
#19071=ORIENTED_EDGE ( 'NONE', *, *, #34130, .F. ) ;
#19103=CARTESIAN_POINT ( 'NONE',  ( 10.31873187879411269, -3.604726614523240613, -4.603124999385506122 ) ) ;
#19105=CARTESIAN_POINT ( 'NONE',  ( 10.56230152254443055, -3.464101615137944457, -7.612500000000054001 ) ) ;
#19107=CARTESIAN_POINT ( 'NONE',  ( 22.56230152254410370, 7.347880794884117764E-16, -6.862499998771004250 ) ) ;
#19112=CARTESIAN_POINT ( 'NONE',  ( 22.80587116629412492, 3.604726614523243278, -1.284374999385501814 ) ) ;
#19120=EDGE_CURVE ( 'NONE', #11418, #18743, #31066, .T. ) ;
#19123=ORIENTED_EDGE ( 'NONE', *, *, #30952, .T. ) ;
#19124=ORIENTED_EDGE ( 'NONE', *, *, #30266, .T. ) ;
#19136=CARTESIAN_POINT ( 'NONE',  ( 19.68408634441910721, -5.407089921784855591, -7.190624999385525129 ) ) ;
#19141=CARTESIAN_POINT ( 'NONE',  ( 16.56230152254411081, -6.928203230275506996, -8.324999998771001941 ) ) ;
#19145=CARTESIAN_POINT ( 'NONE',  ( 10.31873187879410736, -3.604726614523244610, -6.459374999385468996 ) ) ;
#19150=CIRCLE ( 'NONE', #25190, 8.000000000000000000 ) ;
#19152=CARTESIAN_POINT ( 'NONE',  ( 16.56230152254411436, 6.928203230275514990, -4.612500000000012257 ) ) ;
#19174=CARTESIAN_POINT ( 'NONE',  ( 13.44051670066910731, 5.407089921784862696, -7.921874999385513760 ) ) ;
#19183=SHAPE_REPRESENTATION_RELATIONSHIP ( 'NONE' , 'NONE' ,  #201, #20554 ) ;
#19186=CARTESIAN_POINT ( 'NONE',  ( 22.56230152254410370, 7.347880794884117764E-16, -2.362499998771028231 ) ) ;
#19195=CARTESIAN_POINT ( 'NONE',  ( 22.56230152254412147, 7.347880794884125653E-16, -9.225000000000010303 ) ) ;
#19199=CYLINDRICAL_SURFACE ( 'NONE', #36346, 5.999999999999998224 ) ;
#19213=CARTESIAN_POINT ( 'NONE',  ( 13.44051670066911441, -5.407089921784865361, -7.321874999385524774 ) ) ;
#19225=CARTESIAN_POINT ( 'NONE',  ( 10.56230152254357968, 3.464101615137450185, -9.487500000000061107 ) ) ;
#19238=CARTESIAN_POINT ( 'NONE',  ( 16.56230152254411436, 6.928203230275514990, -2.362500000000001155 ) ) ;
#19240=ORIENTED_EDGE ( 'NONE', *, *, #22220, .T. ) ;
#19257=CARTESIAN_POINT ( 'NONE',  ( 22.80587116629411071, 3.604726614523238837, -9.328124999385510208 ) ) ;
#19266=CARTESIAN_POINT ( 'NONE',  ( 22.56230152254410370, 0.000000000000000000, 0.000000000000000000 ) ) ;
#19295=CARTESIAN_POINT ( 'NONE',  ( 22.80587116629410716, 7.646167579472015790E-16, -6.215624999385549465 ) ) ;
#19305=CARTESIAN_POINT ( 'NONE',  ( 13.44051670066911264, -5.407089921784865361, -2.371874999385514826 ) ) ;
#19327=CARTESIAN_POINT ( 'NONE',  ( 10.31873187879411446, 3.604726614523236616, -6.928124999385510741 ) ) ;
#19332=CARTESIAN_POINT ( 'NONE',  ( 10.56230152254411259, 3.464101615137752166, -9.374999998770983112 ) ) ;
#19336=CARTESIAN_POINT ( 'NONE',  ( 19.68408634441911431, -5.407089921784861808, -5.446874999385537208 ) ) ;
#19337=CARTESIAN_POINT ( 'NONE',  ( 22.56230152254446253, -3.464101615137556767, -1.612500000000025357 ) ) ;
#19343=CARTESIAN_POINT ( 'NONE',  ( 16.56230152254410726, 0.000000000000000000, -10.00000000000000000 ) ) ;
#19352=CARTESIAN_POINT ( 'NONE',  ( 19.56230152254411792, -5.196152422706629359, -6.937499998771023968 ) ) ;
#19364=CARTESIAN_POINT ( 'NONE',  ( 10.31873187879410558, 0.000000000000000000, -9.196874999385512339 ) ) ;
#19368=CARTESIAN_POINT ( 'NONE',  ( 10.31873187879411269, -3.604726614523240613, -1.003124999385540450 ) ) ;
#19374=CARTESIAN_POINT ( 'NONE',  ( 19.56230152254410370, 5.196152422706631135, -0.9374999987709908833 ) ) ;
#19380=EDGE_CURVE ( 'NONE', #28622, #4455, #31936, .T. ) ;
#19383=CARTESIAN_POINT ( 'NONE',  ( 13.56230152254410548, 5.196152422706636465, -9.075000000000027711 ) ) ;
#19392=CARTESIAN_POINT ( 'NONE',  ( 16.56230152254410726, 0.000000000000000000, -10.00000000000000000 ) ) ;
#19399=CARTESIAN_POINT ( 'NONE',  ( 10.31873187879410736, 0.000000000000000000, -6.046874999385526195 ) ) ;
#19404=CARTESIAN_POINT ( 'NONE',  ( 22.80587116629412492, 3.604726614523243278, -1.734374999385497551 ) ) ;
#19410=CYLINDRICAL_SURFACE ( 'NONE', #34879, 5.999999999999998224 ) ;
#19411=CARTESIAN_POINT ( 'NONE',  ( 22.56230152254411792, 7.347880794884125653E-16, -6.075000000000052580 ) ) ;
#19419=CARTESIAN_POINT ( 'NONE',  ( 22.56230152254411792, 7.347880794884125653E-16, -1.125000000000042633 ) ) ;
#19438=CARTESIAN_POINT ( 'NONE',  ( 22.80587116629410716, 7.646167579472015790E-16, -8.465624999385523708 ) ) ;
#19448=CARTESIAN_POINT ( 'NONE',  ( 16.56230152254411436, -6.928203230275514990, -4.387500000000030376 ) ) ;
#19452=ADVANCED_FACE ( 'NONE', ( #11844 ), #26430, .F. ) ;
#19475=CARTESIAN_POINT ( 'NONE',  ( 19.68408634441910721, 5.407089921784857367, -7.040624999385541649 ) ) ;
#19484=CARTESIAN_POINT ( 'NONE',  ( 16.56230152254411436, 7.209453229046482114, -2.109374999385531080 ) ) ;
#19489=VECTOR ( 'NONE', #1783, 1000.000000000000000 ) ;
#19491=CARTESIAN_POINT ( 'NONE',  ( 19.68408634441910721, 5.407089921784857367, -1.640624999385525973 ) ) ;
#19497=ORIENTED_EDGE ( 'NONE', *, *, #16324, .F. ) ;
#19504=( BOUNDED_CURVE ( )  B_SPLINE_CURVE ( 2, ( #15813, #26799, #9559, #26610, #639, #3680, #15248 ),
 .UNSPECIFIED., .F., .F. ) 
 B_SPLINE_CURVE_WITH_KNOTS ( ( 3, 2, 2, 3 ),
 ( 0.04347826086956579905, 0.05072463768115918065, 0.05797101449275256224, 0.06521739130434593690 ),
 .UNSPECIFIED. ) 
 CURVE ( )  GEOMETRIC_REPRESENTATION_ITEM ( )  RATIONAL_B_SPLINE_CURVE ( ( 0.9999999999999892308, 0.8660254037844494768, 1.000000000000000000, 0.8660254037844387076, 1.000000000000000000, 0.8660254037844735686, 0.9999999999999651390 ) ) 
 REPRESENTATION_ITEM ( '' )  );
#19514=CARTESIAN_POINT ( 'NONE',  ( 13.56230152254411436, -5.196152422706632912, -7.912499998771055587 ) ) ;
#19517=CARTESIAN_POINT ( 'NONE',  ( 10.31873187879410558, 3.604726614523240613, -10.13437499938549280 ) ) ;
#19518=CARTESIAN_POINT ( 'NONE',  ( 13.44051670066910908, 5.407089921784862696, -7.021874999385530280 ) ) ;
#19543=CARTESIAN_POINT ( 'NONE',  ( 22.56230152254454424, -3.464101615137510137, -9.712500000000012790 ) ) ;
#19545=CARTESIAN_POINT ( 'NONE',  ( 19.68408634441910721, 5.407089921784862696, -9.346874999385523353 ) ) ;
#19549=CARTESIAN_POINT ( 'NONE',  ( 22.80587116629410360, 3.604726614523238837, -3.478124999385532767 ) ) ;
#19555=CARTESIAN_POINT ( 'NONE',  ( 19.56230152254410370, 5.196152422706631135, -1.837499998771002785 ) ) ;
#19561=VECTOR ( 'NONE', #15537, 1000.000000000000000 ) ;
#19562=EDGE_CURVE ( 'NONE', #4918, #9681, #23414, .T. ) ;
#19563=CARTESIAN_POINT ( 'NONE',  ( 13.44051670066911086, 5.407089921784856479, -0.2156249993855441360 ) ) ;
#19579=CARTESIAN_POINT ( 'NONE',  ( 13.44051670066911264, -5.407089921784865361, -5.971874999385562433 ) ) ;
#19585=CARTESIAN_POINT ( 'NONE',  ( 10.31873187879410736, -3.604726614523244610, -2.409374999385539340 ) ) ;
#19587=LINE ( 'NONE', #31136, #37313 ) ;
#19597=FACE_OUTER_BOUND ( 'NONE', #18927, .T. ) ;
#19603=VECTOR ( 'NONE', #15839, 1000.000000000000000 ) ;
#19605=CARTESIAN_POINT ( 'NONE',  ( 13.56230152254411614, -5.196152422706638241, -2.175000000000065548 ) ) ;
#19615=LINE ( 'NONE', #16759, #26644 ) ;
#19626=CARTESIAN_POINT ( 'NONE',  ( 13.44051670066911086, 5.407089921784856479, -9.665624999385530103 ) ) ;
#19635=( GEOMETRIC_REPRESENTATION_CONTEXT ( 3 ) GLOBAL_UNCERTAINTY_ASSIGNED_CONTEXT ( ( #33763 ) ) GLOBAL_UNIT_ASSIGNED_CONTEXT ( ( #28256, #21837, #34125 ) ) REPRESENTATION_CONTEXT ( 'NONE', 'WORKASPACE' ) );
#19636=CARTESIAN_POINT ( 'NONE',  ( 19.56230152254411792, -5.196152422706629359, -2.887499998771053455 ) ) ;
#19637=CARTESIAN_POINT ( 'NONE',  ( 16.56230152254411436, -6.928203230275514990, -1.237499999999996270 ) ) ;
#19645=DIRECTION ( 'NONE',  ( 1.000000000000000000, 0.000000000000000000, 0.000000000000000000 ) ) ;
#19662=EDGE_CURVE ( 'NONE', #26963, #36019, #602, .T. ) ;
#19663=CARTESIAN_POINT ( 'NONE',  ( 22.80587116629410716, 3.604726614523238837, -7.528124999385559235 ) ) ;
#19665=CARTESIAN_POINT ( 'NONE',  ( 13.56230152254411614, -5.196152422706638241, -7.575000000000054357 ) ) ;
#19672=CARTESIAN_POINT ( 'NONE',  ( 10.31873187879411091, 3.604726614523240613, -0.6843749993854860714 ) ) ;
#19678=CARTESIAN_POINT ( 'NONE',  ( 10.31873187879410914, 0.000000000000000000, -1.040624999385536542 ) ) ;
#19695=CARTESIAN_POINT ( 'NONE',  ( 22.80587116629411071, -3.604726614523235284, -9.403124999385534366 ) ) ;
#19706=CARTESIAN_POINT ( 'NONE',  ( 19.68408634441911431, 5.407089921784862696, -5.746874999385531702 ) ) ;
#19715=ORIENTED_EDGE ( 'NONE', *, *, #23847, .T. ) ;
#19721=CARTESIAN_POINT ( 'NONE',  ( 22.56230152254412147, 7.347880794884125653E-16, -4.275000000000028777 ) ) ;
#19730=ORIENTED_EDGE ( 'NONE', *, *, #18990, .T. ) ;
#19737=CARTESIAN_POINT ( 'NONE',  ( 22.80587116629412492, 3.604726614523243278, -8.484374999385497773 ) ) ;
#19740=CARTESIAN_POINT ( 'NONE',  ( 10.31873187879410914, 0.000000000000000000, -3.290624999385538541 ) ) ;
#19744=CARTESIAN_POINT ( 'NONE',  ( 16.56230152254411081, -6.928203230275506996, -2.924999998770990928 ) ) ;
#19747=CARTESIAN_POINT ( 'NONE',  ( 22.56230152254412147, -3.464101615137751278, -3.749999998771020415 ) ) ;
#19754=CARTESIAN_POINT ( 'NONE',  ( 19.68408634441910365, -5.407089921784855591, -0.8906249993855530622 ) ) ;
#19757=CARTESIAN_POINT ( 'NONE',  ( 10.56230152254411081, 0.000000000000000000, -4.837499998771033205 ) ) ;
#19769=B_SPLINE_CURVE_WITH_KNOTS ( 'NONE', 3,
 ( #36049, #15413, #7257, #606, #12175, #9345, #988, #23749, #18645, #9902, #10094, #12564, #35287, #21486, #26768, #9724, #33217, #9532, #20915, #32454, #6498, #18071, #21297, #32833 ),
 .UNSPECIFIED., .F., .F.,
 ( 4, 2, 2, 2, 2, 2, 2, 2, 2, 2, 2, 4 ),
 ( 0.000000000000000000, 0.001514496631480036389, 0.002271744947220054583, 0.003028993262960072777, 0.004543489894440108298, 0.005300738210180123457, 0.006057986525920138615, 0.007572483157400161126, 0.008329731473140176284, 0.009086979788880192310, 0.01060147642036021222, 0.01211597305184023213 ),
 .UNSPECIFIED. ) ;
#19772=CARTESIAN_POINT ( 'NONE',  ( 22.80587116629411426, 7.646167579472024665E-16, -7.171874999385541294 ) ) ;
#19777=CARTESIAN_POINT ( 'NONE',  ( 10.31873187879410203, 3.604726614523240613, -0.2343749993854903624 ) ) ;
#19779=EDGE_CURVE ( 'NONE', #2436, #15581, #20014, .T. ) ;
#19783=CARTESIAN_POINT ( 'NONE',  ( 10.31873187879411091, 0.000000000000000000, -0.1687499993855423597 ) ) ;
#19788=CARTESIAN_POINT ( 'NONE',  ( 22.56230152254411792, 7.347880794884125653E-16, -1.575000000000048583 ) ) ;
#19794=CARTESIAN_POINT ( 'NONE',  ( 10.56230152254411436, -3.464101615137761048, -3.112500000000005596 ) ) ;
#19814=CARTESIAN_POINT ( 'NONE',  ( 24.19849202207518246, 7.686353184319896670, -10.24485366105522743 ) ) ;
#19817=ORIENTED_EDGE ( 'NONE', *, *, #29984, .T. ) ;
#19841=CARTESIAN_POINT ( 'NONE',  ( 10.56230152254410726, 0.000000000000000000, -0.9000000000000396572 ) ) ;
#19845=CARTESIAN_POINT ( 'NONE',  ( 10.31873187879411091, -3.604726614523240613, -7.303124999385512517 ) ) ;
#19854=CARTESIAN_POINT ( 'NONE',  ( 16.56230152254411436, -7.209453229046482114, -2.784374999385508698 ) ) ;
#19860=CARTESIAN_POINT ( 'NONE',  ( 22.80587116629410716, -3.604726614523235284, -0.8531249993855525293 ) ) ;
#19865=VERTEX_POINT ( 'NONE', #31888 ) ;
#19875=EDGE_CURVE ( 'NONE', #25619, #29586, #43, .T. ) ;
#19879=FILL_AREA_STYLE_COLOUR ( '', #37161 ) ;
#19886=VECTOR ( 'NONE', #4059, 1000.000000000000000 ) ;
#19889=CARTESIAN_POINT ( 'NONE',  ( 16.56230152254411081, -7.209453229046482114, -9.084374999385513405 ) ) ;
#19895=CARTESIAN_POINT ( 'NONE',  ( 10.56230152254410903, 0.000000000000000000, -3.487499998771015353 ) ) ;
#19909=VERTEX_POINT ( 'NONE', #24125 ) ;
#19920=CARTESIAN_POINT ( 'NONE',  ( 22.80587116629411781, -3.604726614523235284, -3.553124999385526728 ) ) ;
#19924=DIRECTION ( 'NONE',  ( 0.000000000000000000, 0.000000000000000000, 1.000000000000000000 ) ) ;
#19927=CARTESIAN_POINT ( 'NONE',  ( 22.56230152254410370, -3.464101615137751278, -4.199999998771048126 ) ) ;
#19934=CARTESIAN_POINT ( 'NONE',  ( 22.80587116629411071, 3.604726614523238837, -2.128124999385546001 ) ) ;
#19935=( BOUNDED_CURVE ( )  B_SPLINE_CURVE ( 2, ( #36442, #33424, #22062, #24893, #33613, #10117, #25076 ),
 .UNSPECIFIED., .F., .F. ) 
 B_SPLINE_CURVE_WITH_KNOTS ( ( 3, 2, 2, 3 ),
 ( 0.1304347826086973972, 0.1376811594202916600, 0.1449275362318859506, 0.1521739130434802134 ),
 .UNSPECIFIED. ) 
 CURVE ( )  GEOMETRIC_REPRESENTATION_ITEM ( )  RATIONAL_B_SPLINE_CURVE ( ( 0.9999999999999676925, 0.8660254037844710151, 1.000000000000000000, 0.8660254037844387076, 1.000000000000000000, 0.8660254037844028474, 1.000000000000035971 ) ) 
 REPRESENTATION_ITEM ( '' )  );
#19938=CARTESIAN_POINT ( 'NONE',  ( 10.56230152254259735, -3.464101615136883527, -4.799999998771018461 ) ) ;
#19945=CARTESIAN_POINT ( 'NONE',  ( 19.56230152254411081, -5.196152422706629359, -5.587499998771034093 ) ) ;
#19951=CARTESIAN_POINT ( 'NONE',  ( 19.68408634441910721, 5.407089921784862696, -9.346874999385523353 ) ) ;
#19955=CARTESIAN_POINT ( 'NONE',  ( 16.56230152254411436, -7.209453229046482114, -1.434374999385489735 ) ) ;
#19971=CARTESIAN_POINT ( 'NONE',  ( 13.56230152254410726, 5.196152422706636465, -3.675000000000067324 ) ) ;
#19977=CARTESIAN_POINT ( 'NONE',  ( 19.56230152254412502, 5.196152422706637353, -6.450000000000039257 ) ) ;
#19979=CYLINDRICAL_SURFACE ( 'NONE', #18438, 5.999999999999998224 ) ;
#19989=CARTESIAN_POINT ( 'NONE',  ( 10.31873187879410736, 0.000000000000000000, -0.6468749993855105185 ) ) ;
#19993=VERTEX_POINT ( 'NONE', #36045 ) ;
#20014=( BOUNDED_CURVE ( )  B_SPLINE_CURVE ( 2, ( #23745, #418, #23556, #34916, #35100, #9149, #34545 ),
 .UNSPECIFIED., .F., .F. ) 
 B_SPLINE_CURVE_WITH_KNOTS ( ( 3, 2, 2, 3 ),
 ( 0.4782608695652184050, 0.4855072463768126401, 0.4927536231884069862, 0.5000000000000012212 ),
 .UNSPECIFIED. ) 
 CURVE ( )  GEOMETRIC_REPRESENTATION_ITEM ( )  RATIONAL_B_SPLINE_CURVE ( ( 0.9999999999999815703, 0.8660254037844571373, 1.000000000000000000, 0.8660254037844387076, 1.000000000000000000, 0.8660254037844161701, 1.000000000000022649 ) ) 
 REPRESENTATION_ITEM ( '' )  );
#20022=CARTESIAN_POINT ( 'NONE',  ( 10.31873187879411091, -3.604726614523240613, -6.853124999385484806 ) ) ;
#20036=CARTESIAN_POINT ( 'NONE',  ( 22.80587116629410716, 7.646167579472015790E-16, -3.065624999385535787 ) ) ;
#20044=VERTEX_POINT ( 'NONE', #983 ) ;
#20067=CARTESIAN_POINT ( 'NONE',  ( 22.80587116629411781, -3.604726614523238837, -8.559374999385489957 ) ) ;
#20087=ORIENTED_EDGE ( 'NONE', *, *, #1288, .T. ) ;
#20096=CARTESIAN_POINT ( 'NONE',  ( 10.31873187879411091, 0.000000000000000000, -1.940624999385548444 ) ) ;
#20098=CARTESIAN_POINT ( 'NONE',  ( 22.56230152254412147, 7.347880794884125653E-16, -8.325000000000027711 ) ) ;
#20100=CARTESIAN_POINT ( 'NONE',  ( 13.56230152254411614, -5.196152422706632912, -4.312499998771063048 ) ) ;
#20101=EDGE_CURVE ( 'NONE', #13088, #11631, #841, .T. ) ;
#20110=CARTESIAN_POINT ( 'NONE',  ( 10.56230152254426891, 3.464101615137844981, -8.924999998771019349 ) ) ;
#20128=CARTESIAN_POINT ( 'NONE',  ( 10.31873187879410736, 0.000000000000000000, -7.846874999385494931 ) ) ;
#20133=CARTESIAN_POINT ( 'NONE',  ( 13.44051670066911086, 5.407089921784862696, -3.421874999385537741 ) ) ;
#20152=CARTESIAN_POINT ( 'NONE',  ( 22.56230152254411792, 7.347880794884125653E-16, -4.725000000000035172 ) ) ;
#20160=DIRECTION ( 'NONE',  ( 1.000000000000000000, 0.000000000000000000, 0.000000000000000000 ) ) ;
#20171=CARTESIAN_POINT ( 'NONE',  ( 13.44051670066910908, 5.407089921784862696, -2.071874999385547866 ) ) ;
#20204=CARTESIAN_POINT ( 'NONE',  ( 13.44051670066911086, 5.407089921784856479, -9.215624999385523708 ) ) ;
#20207=CARTESIAN_POINT ( 'NONE',  ( 11.41114437030077866, 3.308917692602460825, -9.999999999999996447 ) ) ;
#20219=CARTESIAN_POINT ( 'NONE',  ( 16.56230152254411436, -7.209453229046475009, -4.528124999385512162 ) ) ;
#20250=CARTESIAN_POINT ( 'NONE',  ( 10.56230152254410903, 0.000000000000000000, -1.800000000000051559 ) ) ;
#20253=CARTESIAN_POINT ( 'NONE',  ( 22.80587116629412492, -3.604726614523238837, -7.659374999385500260 ) ) ;
#20254=CARTESIAN_POINT ( 'NONE',  ( 13.56230152254410903, 5.196152422706636465, -0.07500000000004725109 ) ) ;
#20257=CARTESIAN_POINT ( 'NONE',  ( 16.56230152254410726, 0.000000000000000000, 0.000000000000000000 ) ) ;
#20258=ADVANCED_FACE ( 'NONE', ( #28442 ), #19199, .F. ) ;
#20259=( BOUNDED_CURVE ( )  B_SPLINE_CURVE ( 2, ( #6654, #32993, #3802, #15379, #6842, #29964, #7045 ),
 .UNSPECIFIED., .F., .F. ) 
 B_SPLINE_CURVE_WITH_KNOTS ( ( 3, 2, 2, 3 ),
 ( 0.7391304347826105348, 0.7463768115942048809, 0.7536231884057991159, 0.7608695652173934620 ),
 .UNSPECIFIED. ) 
 CURVE ( )  GEOMETRIC_REPRESENTATION_ITEM ( )  RATIONAL_B_SPLINE_CURVE ( ( 0.9999999999999651390, 0.8660254037844735686, 1.000000000000000000, 0.8660254037844387076, 1.000000000000000000, 0.8660254037843997388, 1.000000000000039080 ) ) 
 REPRESENTATION_ITEM ( '' )  );
#20261=FACE_OUTER_BOUND ( 'NONE', #24353, .T. ) ;
#20269=CARTESIAN_POINT ( 'NONE',  ( 10.56230152254410548, 0.000000000000000000, -4.050000000000054001 ) ) ;
#20285=CARTESIAN_POINT ( 'NONE',  ( 10.31873187879411446, -3.604726614523240613, -2.803124999385555149 ) ) ;
#20289=EDGE_CURVE ( 'NONE', #29417, #20367, #16363, .T. ) ;
#20291=CARTESIAN_POINT ( 'NONE',  ( 10.56230152254411436, 3.464101615137752166, -3.974999998771034715 ) ) ;
#20303=ORIENTED_EDGE ( 'NONE', *, *, #14801, .T. ) ;
#20312=CARTESIAN_POINT ( 'NONE',  ( 10.56230152254410903, 0.000000000000000000, -5.737499998771017573 ) ) ;
#20316=ORIENTED_EDGE ( 'NONE', *, *, #16671, .F. ) ;
#20319=CARTESIAN_POINT ( 'NONE',  ( 16.56230152254411436, -7.209453229046482114, -8.634374999385517668 ) ) ;
#20324=CARTESIAN_POINT ( 'NONE',  ( 19.68408634441910721, 5.407089921784862696, -2.596874999385518024 ) ) ;
#20343=CARTESIAN_POINT ( 'NONE',  ( 10.56230152254410726, 3.464101615137757051, -5.437500000000041744 ) ) ;
#20360=ORIENTED_EDGE ( 'NONE', *, *, #32395, .T. ) ;
#20362=CARTESIAN_POINT ( 'NONE',  ( 10.31873187879411091, 3.604726614523240613, -0.6843749993854860714 ) ) ;
#20367=VERTEX_POINT ( 'NONE', #30938 ) ;
#20385=CARTESIAN_POINT ( 'NONE',  ( 22.56230152254411792, 7.347880794884125653E-16, -5.175000000000040679 ) ) ;
#20388=VERTEX_POINT ( 'NONE', #20685 ) ;
#20396=CARTESIAN_POINT ( 'NONE',  ( 10.31873187879411091, 3.604726614523236616, -7.828124999385535965 ) ) ;
#20399=CARTESIAN_POINT ( 'NONE',  ( 10.53357014895476951, 1.237016744030756454, -9.999999999999998224 ) ) ;
#20408=CARTESIAN_POINT ( 'NONE',  ( 16.56230152254410726, 0.000000000000000000, -10.00000000000000000 ) ) ;
#20409=CARTESIAN_POINT ( 'NONE',  ( 22.80587116629410360, 3.604726614523238837, -3.478124999385532767 ) ) ;
#20415=ORIENTED_EDGE ( 'NONE', *, *, #36569, .T. ) ;
#20416=FACE_BOUND ( 'NONE', #34613, .T. ) ;
#20420=AXIS2_PLACEMENT_3D ( 'NONE', #8220, #29177, #3219 ) ;
#20438=CARTESIAN_POINT ( 'NONE',  ( 10.56230152254411259, 0.000000000000000000, -10.23749999877102113 ) ) ;
#20443=CARTESIAN_POINT ( 'NONE',  ( 19.68408634441911786, -5.407089921784861808, -9.496874999385534366 ) ) ;
#20449=CARTESIAN_POINT ( 'NONE',  ( 16.56230152254410726, 0.000000000000000000, -10.00000000000000000 ) ) ;
#20451=ORIENTED_EDGE ( 'NONE', *, *, #28157, .T. ) ;
#20463=VERTEX_POINT ( 'NONE', #8555 ) ;
#20473=CARTESIAN_POINT ( 'NONE',  ( 22.80587116629410716, 7.646167579472015790E-16, -4.865624999385531169 ) ) ;
#20478=CARTESIAN_POINT ( 'NONE',  ( 10.56230152254410903, 3.464101615137752166, -2.624999998770982668 ) ) ;
#20485=CARTESIAN_POINT ( 'NONE',  ( 13.56230152254410726, 5.196152422706636465, -8.175000000000043343 ) ) ;
#20488=FACE_OUTER_BOUND ( 'NONE', #6637, .T. ) ;
#20491=EDGE_LOOP ( 'NONE', ( #26396, #1537, #24372, #14052 ) ) ;
#20505=ORIENTED_EDGE ( 'NONE', *, *, #15854, .F. ) ;
#20508=CARTESIAN_POINT ( 'NONE',  ( 16.56230152254411081, -7.209453229046482114, -9.084374999385513405 ) ) ;
#20513=CARTESIAN_POINT ( 'NONE',  ( 22.80587116629411781, 7.646167579472024665E-16, -4.921874999385511984 ) ) ;
#20529=CARTESIAN_POINT ( 'NONE',  ( 19.56230152254412147, -5.196152422706635576, -5.250000000000060396 ) ) ;
#20532=DIRECTION ( 'NONE',  ( 0.000000000000000000, 0.000000000000000000, 1.000000000000000000 ) ) ;
#20546=CARTESIAN_POINT ( 'NONE',  ( 10.31873187879410558, 3.604726614523240613, -2.484374999385500882 ) ) ;
#20554=ADVANCED_BREP_SHAPE_REPRESENTATION ( '', ( #7886, #17215 ), #24466 ) ;
#20578=CARTESIAN_POINT ( 'NONE',  ( 22.80587116629411071, 3.604726614523238837, -9.778124999385537919 ) ) ;
#20579=CARTESIAN_POINT ( 'NONE',  ( 10.56230152254305032, 3.464101615137144652, -8.587500000000064304 ) ) ;
#20581=CARTESIAN_POINT ( 'NONE',  ( 11.14485736792927284, 2.876095549794589257, -10.00000000000000000 ) ) ;
#20593=CARTESIAN_POINT ( 'NONE',  ( 22.80587116629410716, 7.646167579472015790E-16, -3.965624999385547689 ) ) ;
#20627=CARTESIAN_POINT ( 'NONE',  ( 16.56230152254411436, -7.209453229046482114, -7.734374999385493332 ) ) ;
#20629=CARTESIAN_POINT ( 'NONE',  ( 22.80587116629411071, 3.604726614523238837, -1.228124999385522331 ) ) ;
#20657=CARTESIAN_POINT ( 'NONE',  ( 16.56230152254411081, 7.209453229046475009, -4.303124999385498306 ) ) ;
#20663=CARTESIAN_POINT ( 'NONE',  ( 19.56230152254410370, 5.196152422706631135, -7.237499998771018461 ) ) ;
#20685=CARTESIAN_POINT ( 'NONE',  ( 22.56230152254412502, 7.347880794884125653E-16, -2.925000000000066436 ) ) ;
#20694=CARTESIAN_POINT ( 'NONE',  ( 16.56230152254411436, 7.209453229046482114, -3.459374999385518734 ) ) ;
#20713=CARTESIAN_POINT ( 'NONE',  ( 16.56230152254411436, 6.928203230275514990, -5.512500000000036593 ) ) ;
#20731=CARTESIAN_POINT ( 'NONE',  ( 13.44051670066911264, 5.407089921784862696, -2.521874999385525840 ) ) ;
#20736=EDGE_CURVE ( 'NONE', #24665, #25759, #17806, .T. ) ;
#20741=( BOUNDED_CURVE ( )  B_SPLINE_CURVE ( 2, ( #1213, #32875, #26432, #20767, #9387, #12221, #12412 ),
 .UNSPECIFIED., .F., .F. ) 
 B_SPLINE_CURVE_WITH_KNOTS ( ( 3, 2, 2, 3 ),
 ( 0.2391304347826091470, 0.2463768115942034931, 0.2536231884057978392, 0.2608695652173921298 ),
 .UNSPECIFIED. ) 
 CURVE ( )  GEOMETRIC_REPRESENTATION_ITEM ( )  RATIONAL_B_SPLINE_CURVE ( ( 0.9999999999999917843, 0.8660254037844469233, 1.000000000000000000, 0.8660254037844387076, 1.000000000000000000, 0.8660254037844232755, 1.000000000000015321 ) ) 
 REPRESENTATION_ITEM ( '' )  );
#20766=CARTESIAN_POINT ( 'NONE',  ( 16.56230152254411081, -7.209453229046475009, -9.028124999385500615 ) ) ;
#20767=CARTESIAN_POINT ( 'NONE',  ( 16.56230152254411792, -6.928203230275514990, -2.587500000000015454 ) ) ;
#20769=CARTESIAN_POINT ( 'NONE',  ( 10.59328565399995803, 1.478247113626270481, -10.00000000000000355 ) ) ;
#20771=DIRECTION ( 'NONE',  ( -0.000000000000000000, -0.000000000000000000, -1.000000000000000000 ) ) ;
#20778=EDGE_CURVE ( 'NONE', #28622, #11418, #4939, .T. ) ;
#20780=CARTESIAN_POINT ( 'NONE',  ( 10.31873187879411269, 3.604726614523236616, -4.678124999385532945 ) ) ;
#20794=DIRECTION ( 'NONE',  ( 1.000000000000000000, 0.000000000000000000, 0.000000000000000000 ) ) ;
#20817=CARTESIAN_POINT ( 'NONE',  ( 16.56230152254411436, -7.209453229046475009, -1.378124999385542226 ) ) ;
#20819=DIRECTION ( 'NONE',  ( 0.000000000000000000, 0.000000000000000000, -1.000000000000000000 ) ) ;
#20848=CARTESIAN_POINT ( 'NONE',  ( 10.31873187879411269, 3.604726614523236616, -6.028124999385552130 ) ) ;
#20849=EDGE_CURVE ( 'NONE', #27522, #23999, #32095, .T. ) ;
#20855=CARTESIAN_POINT ( 'NONE',  ( 10.56230152254411614, -3.464101615137757051, -7.049999998771010468 ) ) ;
#20861=CARTESIAN_POINT ( 'NONE',  ( 10.31873187879411269, 3.604726614523240613, -4.284374999385515359 ) ) ;
#20866=CARTESIAN_POINT ( 'NONE',  ( 10.44051670066910908, 0.000000000000000000, -0.2671874990782807657 ) ) ;
#20875=CARTESIAN_POINT ( 'NONE',  ( 19.56230152254410726, 5.196152422706631135, -5.887499998771001053 ) ) ;
#20887=CARTESIAN_POINT ( 'NONE',  ( 10.31873187879410736, 0.000000000000000000, -3.346874999385518468 ) ) ;
#20898=AXIS2_PLACEMENT_3D ( 'NONE', #25934, #36744, #10784 ) ;
#20906=CARTESIAN_POINT ( 'NONE',  ( 19.56230152254412502, 5.196152422706637353, -6.450000000000039257 ) ) ;
#20915=CARTESIAN_POINT ( 'NONE',  ( 18.47613065999978232, -5.877663906574049690, -10.00000000000000178 ) ) ;
#20924=CARTESIAN_POINT ( 'NONE',  ( 16.56230152254411436, 7.209453229046482114, -3.009374999385522553 ) ) ;
#20931=VERTEX_POINT ( 'NONE', #22538 ) ;
#20932=( BOUNDED_CURVE ( )  B_SPLINE_CURVE ( 2, ( #7875, #5017, #2549, #19448, #22467, #28141, #10895 ),
 .UNSPECIFIED., .F., .F. ) 
 B_SPLINE_CURVE_WITH_KNOTS ( ( 3, 2, 2, 3 ),
 ( 0.4130434782608670141, 0.4202898550724613047, 0.4275362318840557063, 0.4347826086956499969 ),
 .UNSPECIFIED. ) 
 CURVE ( )  GEOMETRIC_REPRESENTATION_ITEM ( )  RATIONAL_B_SPLINE_CURVE ( ( 1.000000000000047296, 0.8660254037843915231, 1.000000000000000000, 0.8660254037844387076, 1.000000000000000000, 0.8660254037844787867, 0.9999999999999599209 ) ) 
 REPRESENTATION_ITEM ( '' )  );
#20936=CARTESIAN_POINT ( 'NONE',  ( 13.56230152254410548, 5.196152422706630247, -6.262499998771015264 ) ) ;
#20940=DIRECTION ( 'NONE',  ( 0.000000000000000000, 0.000000000000000000, 1.000000000000000000 ) ) ;
#20954=EDGE_CURVE ( 'NONE', #2700, #32942, #17584, .T. ) ;
#20956=DIRECTION ( 'NONE',  ( 0.000000000000000000, 0.000000000000000000, 1.000000000000000000 ) ) ;
#20960=CARTESIAN_POINT ( 'NONE',  ( 22.80587116629411071, -3.604726614523235284, -8.503124999385544669 ) ) ;
#20973=CARTESIAN_POINT ( 'NONE',  ( 10.31873187879410736, 0.000000000000000000, -4.190624999385549998 ) ) ;
#20981=CARTESIAN_POINT ( 'NONE',  ( 13.56230152254411436, -5.196152422706632912, -2.062499998771005760 ) ) ;
#21001=EDGE_CURVE ( 'NONE', #36330, #32727, #19150, .T. ) ;
#21009=CARTESIAN_POINT ( 'NONE',  ( 10.31873187879411091, 3.604726614523236616, -1.078124999385534410 ) ) ;
#21038=CARTESIAN_POINT ( 'NONE',  ( 19.68408634441910365, -5.407089921784855591, -5.840624999385535254 ) ) ;
#21044=CARTESIAN_POINT ( 'NONE',  ( 19.56230152254411081, 5.196152422706631135, -5.437499998771022192 ) ) ;
#21050=CARTESIAN_POINT ( 'NONE',  ( 10.31873187879410558, 3.604726614523240613, -2.934374999385496618 ) ) ;
#21062=CARTESIAN_POINT ( 'NONE',  ( 13.56230152254411792, -5.196152422706638241, -4.875000000000101252 ) ) ;
#21080=ORIENTED_EDGE ( 'NONE', *, *, #2868, .F. ) ;
#21081=CARTESIAN_POINT ( 'NONE',  ( 22.80587116629411426, 3.604726614523243278, -7.134374999385543425 ) ) ;
#21090=ORIENTED_EDGE ( 'NONE', *, *, #15688, .T. ) ;
#21097=CARTESIAN_POINT ( 'NONE',  ( 19.56230152254412502, -5.196152422706635576, -7.050000000000084199 ) ) ;
#21107=CARTESIAN_POINT ( 'NONE',  ( 13.56230152254410903, 5.196152422706636465, -5.475000000000035172 ) ) ;
#21112=VERTEX_POINT ( 'NONE', #16855 ) ;
#21115=CARTESIAN_POINT ( 'NONE',  ( 16.56230152254411436, -7.209453229046482114, -4.584374999385491201 ) ) ;
#21120=ORIENTED_EDGE ( 'NONE', *, *, #10140, .F. ) ;
#21132=( BOUNDED_CURVE ( )  B_SPLINE_CURVE ( 2, ( #29079, #31564, #5587, #28715, #24350, #837, #10124 ),
 .UNSPECIFIED., .F., .F. ) 
 B_SPLINE_CURVE_WITH_KNOTS ( ( 3, 2, 2, 3 ),
 ( 0.9130434782608737310, 0.9202898550724665228, 0.9275362318840592035, 0.9334794156559244049 ),
 .UNSPECIFIED. ) 
 CURVE ( )  GEOMETRIC_REPRESENTATION_ITEM ( )  RATIONAL_B_SPLINE_CURVE ( ( 0.9999999999999219513, 0.8660254037845167563, 1.000000000000000000, 0.8660254037844387076, 1.000000000000000000, 0.8901194808422465687, 0.9604780343360148631 ) ) 
 REPRESENTATION_ITEM ( '' )  );
#21148=CARTESIAN_POINT ( 'NONE',  ( 22.56230152254351395, 3.464101615138092782, -7.724999998770981868 ) ) ;
#21158=CARTESIAN_POINT ( 'NONE',  ( 16.56230152254411436, -7.209453229046475009, -7.228124999385518556 ) ) ;
#21166=CARTESIAN_POINT ( 'NONE',  ( 22.56230152254410370, 7.347880794884117764E-16, -1.912499998771022280 ) ) ;
#21196=CARTESIAN_POINT ( 'NONE',  ( 19.68408634441911076, 5.407089921784857367, -4.790624999385539873 ) ) ;
#21226=CARTESIAN_POINT ( 'NONE',  ( 22.80587116629411781, 3.604726614523238837, -4.378124999385524241 ) ) ;
#21230=LINE ( 'NONE', #35230, #17017 ) ;
#21231=AXIS2_PLACEMENT_3D ( 'NONE', #3339, #23632, #20794 ) ;
#21234=CARTESIAN_POINT ( 'NONE',  ( 10.56230152254410726, 0.000000000000000000, -6.637499998771001941 ) ) ;
#21238=CARTESIAN_POINT ( 'NONE',  ( 19.68408634441911076, 5.407089921784862696, -3.946874999385563410 ) ) ;
#21241=CARTESIAN_POINT ( 'NONE',  ( 10.31873187879411091, 0.000000000000000000, -0.1406249993855246405 ) ) ;
#21251=CARTESIAN_POINT ( 'NONE',  ( 22.56230152254410370, 7.347880794884117764E-16, -5.062499998771007981 ) ) ;
#21267=ORIENTED_EDGE ( 'NONE', *, *, #3669, .F. ) ;
#21268=CARTESIAN_POINT ( 'NONE',  ( 10.31873187879410736, -3.604726614523244610, -5.109374999385545735 ) ) ;
#21276=CARTESIAN_POINT ( 'NONE',  ( 13.56230152254411614, -5.196152422706632912, -9.712499998771024323 ) ) ;
#21288=CARTESIAN_POINT ( 'NONE',  ( 22.56230152254411436, 3.464101615137759271, -7.387500000000012612 ) ) ;
#21297=CARTESIAN_POINT ( 'NONE',  ( 15.75780091040682862, -6.201764924782260380, -10.00000000000000000 ) ) ;
#21305=CARTESIAN_POINT ( 'NONE',  ( 22.80587116629412137, 7.646167579472024665E-16, -3.571874999385521221 ) ) ;
#21319=EDGE_CURVE ( 'NONE', #29192, #8245, #21465, .T. ) ;
#21322=CARTESIAN_POINT ( 'NONE',  ( 10.56230152254410903, 0.000000000000000000, -7.200000000000040146 ) ) ;
#21347=CARTESIAN_POINT ( 'NONE',  ( 16.56230152254411081, 7.209453229046475009, -6.103124999385545202 ) ) ;
#21353=CARTESIAN_POINT ( 'NONE',  ( 24.56230152254410726, 0.000000000000000000, -10.00000000000000000 ) ) ;
#21382=CARTESIAN_POINT ( 'NONE',  ( 22.80587116629410716, 7.646167579472015790E-16, -5.315624999385537564 ) ) ;
#21388=CARTESIAN_POINT ( 'NONE',  ( 13.56230152254411614, -5.196152422706638241, -8.475000000000093792 ) ) ;
#21397=AXIS2_PLACEMENT_3D ( 'NONE', #1272, #35582, #9438 ) ;
#21401=ORIENTED_EDGE ( 'NONE', *, *, #16877, .T. ) ;
#21412=CARTESIAN_POINT ( 'NONE',  ( 22.80587116629410360, 7.646167579472015790E-16, -8.015624999385517313 ) ) ;
#21418=CARTESIAN_POINT ( 'NONE',  ( 13.56230152254411436, -5.196152422706632912, -6.112499998771031784 ) ) ;
#21423=CARTESIAN_POINT ( 'NONE',  ( 19.68408634441911786, -5.407089921784861808, -4.546874999385525307 ) ) ;
#21436=CARTESIAN_POINT ( 'NONE',  ( 22.56230152254411792, 7.347880794884125653E-16, -4.725000000000035172 ) ) ;
#21455=CARTESIAN_POINT ( 'NONE',  ( 10.31873187879410736, 0.000000000000000000, -5.596874999385520688 ) ) ;
#21465=( BOUNDED_CURVE ( )  B_SPLINE_CURVE ( 2, ( #24123, #19006, #25043, #5135, #25235, #27889, #7809 ),
 .UNSPECIFIED., .F., .F. ) 
 B_SPLINE_CURVE_WITH_KNOTS ( ( 3, 2, 2, 3 ),
 ( 0.3260869565217380805, 0.3333333333333323711, 0.3405797101449267728, 0.3478260869565210633 ),
 .UNSPECIFIED. ) 
 CURVE ( )  GEOMETRIC_REPRESENTATION_ITEM ( )  RATIONAL_B_SPLINE_CURVE ( ( 1.000000000000019540, 0.8660254037844192787, 1.000000000000000000, 0.8660254037844387076, 1.000000000000000000, 0.8660254037844510311, 0.9999999999999876765 ) ) 
 REPRESENTATION_ITEM ( '' )  );
#21473=EDGE_CURVE ( 'NONE', #21578, #16024, #12700, .T. ) ;
#21477=CARTESIAN_POINT ( 'NONE',  ( 16.56230152254411436, 6.928203230275514990, -7.312500000000050626 ) ) ;
#21486=CARTESIAN_POINT ( 'NONE',  ( 20.43890260697799377, -4.778814664990964189, -9.999999999999994671 ) ) ;
#21489=( BOUNDED_CURVE ( )  B_SPLINE_CURVE ( 2, ( #20269, #11167, #22926, #8879, #34290, #34099, #19721 ),
 .UNSPECIFIED., .F., .F. ) 
 B_SPLINE_CURVE_WITH_KNOTS ( ( 3, 2, 2, 3 ),
 ( 0.3913043478260868624, 0.3985507246376802093, 0.4057971014492736672, 0.4130434782608670141 ),
 .UNSPECIFIED. ) 
 CURVE ( )  GEOMETRIC_REPRESENTATION_ITEM ( )  RATIONAL_B_SPLINE_CURVE ( ( 1.000000000000001998, 0.8660254037844367092, 1.000000000000000000, 0.8660254037844387076, 1.000000000000000000, 0.8660254037844858921, 0.9999999999999528155 ) ) 
 REPRESENTATION_ITEM ( '' )  );
#21494=CARTESIAN_POINT ( 'NONE',  ( 10.31873187879410736, 0.000000000000000000, -2.896874999385512517 ) ) ;
#21516=DIRECTION ( 'NONE',  ( 1.000000000000000000, 0.000000000000000000, 0.000000000000000000 ) ) ;
#21526=VECTOR ( 'NONE', #5094, 1000.000000000000000 ) ;
#21534=CARTESIAN_POINT ( 'NONE',  ( 16.56230152254411081, 7.209453229046475009, -6.553124999385508964 ) ) ;
#21556=AXIS2_PLACEMENT_3D ( 'NONE', #15471, #863, #17572 ) ;
#21569=CARTESIAN_POINT ( 'NONE',  ( 22.80587116629411426, -3.604726614523235284, -3.103124999385563410 ) ) ;
#21578=VERTEX_POINT ( 'NONE', #24674 ) ;
#21590=ORIENTED_EDGE ( 'NONE', *, *, #79, .F. ) ;
#21591=ORIENTED_EDGE ( 'NONE', *, *, #31021, .T. ) ;
#21600=CARTESIAN_POINT ( 'NONE',  ( 22.80587116629410360, 7.646167579472015790E-16, -7.565624999385539340 ) ) ;
#21605=CARTESIAN_POINT ( 'NONE',  ( 10.56230152254410903, 3.464101615137752166, -8.474999998771021836 ) ) ;
#21608=CARTESIAN_POINT ( 'NONE',  ( 22.80587116629412847, -3.604726614523238837, -3.159374999385510474 ) ) ;
#21619=LINE ( 'NONE', #7215, #30178 ) ;
#21624=CARTESIAN_POINT ( 'NONE',  ( 13.44051670066911619, -5.407089921784859143, -1.415624999385550753 ) ) ;
#21627=ORIENTED_EDGE ( 'NONE', *, *, #9607, .T. ) ;
#21635=CARTESIAN_POINT ( 'NONE',  ( 10.31873187879410736, 3.604726614523240613, -6.084374999385531169 ) ) ;
#21655=CARTESIAN_POINT ( 'NONE',  ( 10.56230152254411436, -3.464101615137761048, -8.062500000000023093 ) ) ;
#21664=CARTESIAN_POINT ( 'NONE',  ( 19.56230152254412502, 5.196152422706637353, -5.550000000000054889 ) ) ;
#21670=CARTESIAN_POINT ( 'NONE',  ( 13.44051670066911441, -5.407089921784865361, -5.071874999385522997 ) ) ;
#21678=EDGE_CURVE ( 'NONE', #36019, #7808, #30414, .T. ) ;
#21696=CARTESIAN_POINT ( 'NONE',  ( 16.56230152254410726, 0.000000000000000000, -10.00000000000000000 ) ) ;
#21699=VERTEX_POINT ( 'NONE', #25603 ) ;
#21703=CARTESIAN_POINT ( 'NONE',  ( 10.56230152254410903, 0.000000000000000000, -0.7874999987710074034 ) ) ;
#21715=CARTESIAN_POINT ( 'NONE',  ( 22.80587116629410716, 3.604726614523238837, -6.628124999385534899 ) ) ;
#21719=ORIENTED_EDGE ( 'NONE', *, *, #18149, .F. ) ;
#21726=CARTESIAN_POINT ( 'NONE',  ( 19.56230152254412147, -5.196152422706635576, -9.300000000000057554 ) ) ;
#21753=CARTESIAN_POINT ( 'NONE',  ( 19.68408634441910721, -5.407089921784855591, -3.140624999385555061 ) ) ;
#21755=CARTESIAN_POINT ( 'NONE',  ( 19.56230152254412502, -5.196152422706635576, -7.500000000000062172 ) ) ;
#21758=CYLINDRICAL_SURFACE ( 'NONE', #15303, 5.999999999999998224 ) ;
#21763=CARTESIAN_POINT ( 'NONE',  ( 22.80587116629411781, 7.646167579472024665E-16, -0.4218749993855352987 ) ) ;
#21775=VERTEX_POINT ( 'NONE', #8917 ) ;
#21784=CARTESIAN_POINT ( 'NONE',  ( 19.68408634441910721, -5.407089921784855591, -7.640624999385531524 ) ) ;
#21790=CARTESIAN_POINT ( 'NONE',  ( 10.56230152254410903, -3.464101615137757051, -7.499999998771006204 ) ) ;
#21793=CARTESIAN_POINT ( 'NONE',  ( 10.31873187879411091, 3.604726614523240613, -6.534374999385494043 ) ) ;
#21822=CARTESIAN_POINT ( 'NONE',  ( 10.31873187879410736, 0.000000000000000000, -6.046874999385526195 ) ) ;
#21826=CARTESIAN_POINT ( 'NONE',  ( 22.56230152254411792, 7.347880794884125653E-16, -6.525000000000058975 ) ) ;
#21833=CARTESIAN_POINT ( 'NONE',  ( 10.56230152254411436, 3.464101615137752166, -0.8249999987710000537 ) ) ;
#21837=( NAMED_UNIT ( * ) PLANE_ANGLE_UNIT ( ) SI_UNIT ( $, .RADIAN. ) );
#21842=CARTESIAN_POINT ( 'NONE',  ( 22.56230152254412147, 3.464101615137759271, -9.637499999999990408 ) ) ;
#21851=LINE ( 'NONE', #16534, #8943 ) ;
#21857=CARTESIAN_POINT ( 'NONE',  ( 10.31873187879411091, 3.604726614523240613, -5.184374999385507721 ) ) ;
#21879=CARTESIAN_POINT ( 'NONE',  ( 10.56230152254410903, 0.000000000000000000, -2.700000000000063238 ) ) ;
#21885=CARTESIAN_POINT ( 'NONE',  ( 10.56230152254383903, -3.464101615137598067, -0.7499999987710416205 ) ) ;
#21894=EDGE_LOOP ( 'NONE', ( #33366, #34936, #667, #1971 ) ) ;
#21898=CARTESIAN_POINT ( 'NONE',  ( 22.80587116629411071, 3.604726614523238837, -5.728124999385511451 ) ) ;
#21906=ORIENTED_EDGE ( 'NONE', *, *, #195, .F. ) ;
#21914=CARTESIAN_POINT ( 'NONE',  ( 16.56230152254411436, -6.928203230275514990, -5.737500000000049560 ) ) ;
#21940=CARTESIAN_POINT ( 'NONE',  ( 19.68408634441910721, -5.407089921784855591, -3.590624999385533478 ) ) ;
#21947=CARTESIAN_POINT ( 'NONE',  ( 22.56230152254410015, 7.347880794884117764E-16, -7.762499998770988618 ) ) ;
#21949=CARTESIAN_POINT ( 'NONE',  ( 13.44051670066911086, 5.407089921784862696, -0.7218749993855300140 ) ) ;
#21956=CARTESIAN_POINT ( 'NONE',  ( 16.56230152254411081, 6.928203230275506996, -4.049999998770996257 ) ) ;
#21968=( BOUNDED_CURVE ( )  B_SPLINE_CURVE ( 2, ( #12414, #30035, #10316, #16020, #12789, #21148, #30608 ),
 .UNSPECIFIED., .F., .F. ) 
 B_SPLINE_CURVE_WITH_KNOTS ( ( 3, 2, 2, 3 ),
 ( 0.6956521739130446802, 0.7028985507246381381, 0.7101449275362314850, 0.7173913043478248319 ),
 .UNSPECIFIED. ) 
 CURVE ( )  GEOMETRIC_REPRESENTATION_ITEM ( )  RATIONAL_B_SPLINE_CURVE ( ( 0.9999999999999774625, 0.8660254037844612451, 1.000000000000000000, 0.8660254037844387076, 1.000000000000000000, 0.8660254037844612451, 0.9999999999999774625 ) ) 
 REPRESENTATION_ITEM ( '' )  );
#21972=CARTESIAN_POINT ( 'NONE',  ( 22.80587116629410360, 7.646167579472015790E-16, -7.115624999385533833 ) ) ;
#21978=CARTESIAN_POINT ( 'NONE',  ( 16.56230152254411081, -6.928203230275506996, -9.224999998771027165 ) ) ;
#21983=CARTESIAN_POINT ( 'NONE',  ( 13.44051670066911086, 5.407089921784862696, -6.121874999385518379 ) ) ;
#21989=CARTESIAN_POINT ( 'NONE',  ( 10.56230152254410903, 0.000000000000000000, -4.500000000000031974 ) ) ;
#22006=CARTESIAN_POINT ( 'NONE',  ( 11.28998163430637725, -3.344369132205555317, -9.999999999999998224 ) ) ;
#22008=CARTESIAN_POINT ( 'NONE',  ( 13.44051670066910908, 5.407089921784862696, -9.271874999385531169 ) ) ;
#22012=CARTESIAN_POINT ( 'NONE',  ( 19.68408634441910721, 5.407089921784857367, -0.2906249993855358760 ) ) ;
#22018=CARTESIAN_POINT ( 'NONE',  ( 13.56230152254411259, -5.196152422706632912, -2.962499998771017662 ) ) ;
#22021=CARTESIAN_POINT ( 'NONE',  ( 19.56230152254410370, 5.196152422706631135, -2.287499998770980980 ) ) ;
#22028=CARTESIAN_POINT ( 'NONE',  ( 13.56230152254411614, -5.196152422706638241, -9.825000000000056133 ) ) ;
#22033=DIRECTION ( 'NONE',  ( 1.000000000000000000, 0.000000000000000000, 0.000000000000000000 ) ) ;
#22046=CARTESIAN_POINT ( 'NONE',  ( 19.68408634441911431, 5.407089921784862696, -6.646874999385543603 ) ) ;
#22056=CARTESIAN_POINT ( 'NONE',  ( 13.56230152254410548, 5.196152422706636465, -9.525000000000034106 ) ) ;
#22062=CARTESIAN_POINT ( 'NONE',  ( 13.56230152254410548, 5.196152422706630247, -1.762499998771011045 ) ) ;
#22069=CARTESIAN_POINT ( 'NONE',  ( 16.56230152254411436, 6.928203230275514990, -1.462500000000010125 ) ) ;
#22088=CARTESIAN_POINT ( 'NONE',  ( 10.31873187879411091, 3.604726614523236616, -9.628124999385549998 ) ) ;
#22117=VECTOR ( 'NONE', #25705, 1000.000000000000000 ) ;
#22125=CARTESIAN_POINT ( 'NONE',  ( 10.31873187879410914, 0.000000000000000000, -5.540624999385540761 ) ) ;
#22128=CARTESIAN_POINT ( 'NONE',  ( 10.56230152254410726, 0.000000000000000000, -7.650000000000045652 ) ) ;
#22134=CARTESIAN_POINT ( 'NONE',  ( 19.56230152254412147, 5.196152422706637353, -6.900000000000044764 ) ) ;
#22136=CARTESIAN_POINT ( 'NONE',  ( 19.68408634441912142, -5.407089921784861808, -1.846874999385544891 ) ) ;
#22138=ORIENTED_EDGE ( 'NONE', *, *, #23847, .F. ) ;
#22147=ORIENTED_EDGE ( 'NONE', *, *, #30201, .T. ) ;
#22158=CARTESIAN_POINT ( 'NONE',  ( 22.56230152254411792, 7.347880794884125653E-16, -1.575000000000048583 ) ) ;
#22160=CARTESIAN_POINT ( 'NONE',  ( 10.31873187879411091, 3.604726614523236616, -7.378124999385538452 ) ) ;
#22165=CARTESIAN_POINT ( 'NONE',  ( 16.56230152254411436, 6.928203230275506996, -7.649999998770994125 ) ) ;
#22169=CARTESIAN_POINT ( 'NONE',  ( 19.68408634441911431, 5.407089921784862696, -7.096874999385549998 ) ) ;
#22170=DIRECTION ( 'NONE',  ( 0.000000000000000000, 0.000000000000000000, 1.000000000000000000 ) ) ;
#22198=CARTESIAN_POINT ( 'NONE',  ( 16.56230152254411436, 7.209453229046482114, -8.409374999385503813 ) ) ;
#22202=CARTESIAN_POINT ( 'NONE',  ( 10.31873187879410914, 0.000000000000000000, -1.040624999385536542 ) ) ;
#22208=CARTESIAN_POINT ( 'NONE',  ( 13.56230152254411614, -5.196152422706632912, -1.162499998771021614 ) ) ;
#22209=ORIENTED_EDGE ( 'NONE', *, *, #20954, .F. ) ;
#22216=CARTESIAN_POINT ( 'NONE',  ( 10.56230152254410903, 3.464101615137757051, -9.037500000000038725 ) ) ;
#22220=EDGE_CURVE ( 'NONE', #18566, #20367, #37072, .T. ) ;
#22233=CARTESIAN_POINT ( 'NONE',  ( 22.80587116629411781, -3.604726614523238837, -5.859374999385517313 ) ) ;
#22240=CARTESIAN_POINT ( 'NONE',  ( 22.80587116629411426, 3.604726614523243278, -2.184374999385525040 ) ) ;
#22257=CARTESIAN_POINT ( 'NONE',  ( 19.56230152254412502, -5.196152422706635576, -2.100000000000074252 ) ) ;
#22264=CARTESIAN_POINT ( 'NONE',  ( 16.56230152254410726, 0.000000000000000000, -10.00000000000000000 ) ) ;
#22274=CARTESIAN_POINT ( 'NONE',  ( 10.31873187879411091, 3.604726614523236616, -8.728124999385524774 ) ) ;
#22284=DIRECTION ( 'NONE',  ( 0.000000000000000000, 0.000000000000000000, 1.000000000000000000 ) ) ;
#22300=ORIENTED_EDGE ( 'NONE', *, *, #24256, .F. ) ;
#22308=CARTESIAN_POINT ( 'NONE',  ( 19.68408634441910721, 5.407089921784857367, -7.490624999385548044 ) ) ;
#22317=CARTESIAN_POINT ( 'NONE',  ( 22.80587116629411071, -3.604726614523238837, -1.359374999385495775 ) ) ;
#22323=CARTESIAN_POINT ( 'NONE',  ( 13.44051670066911264, 5.407089921784856479, -1.565624999385561988 ) ) ;
#22339=CARTESIAN_POINT ( 'NONE',  ( 13.44051670066911619, -5.407089921784859143, -9.965624999385552130 ) ) ;
#22346=CARTESIAN_POINT ( 'NONE',  ( 13.56230152254410370, 5.196152422706630247, -7.612499998771005139 ) ) ;
#22351=CARTESIAN_POINT ( 'NONE',  ( 22.80587116629411426, 7.646167579472024665E-16, -7.171874999385541294 ) ) ;
#22355=FACE_OUTER_BOUND ( 'NONE', #17096, .T. ) ;
#22358=CARTESIAN_POINT ( 'NONE',  ( 22.56230152254410370, 0.000000000000000000, -10.00000000000000000 ) ) ;
#22360=ORIENTED_EDGE ( 'NONE', *, *, #13190, .F. ) ;
#22367=CYLINDRICAL_SURFACE ( 'NONE', #5316, 5.999999999999998224 ) ;
#22369=CARTESIAN_POINT ( 'NONE',  ( 10.56230152254410726, 0.000000000000000000, -7.087499998771007448 ) ) ;
#22381=CARTESIAN_POINT ( 'NONE',  ( 13.44051670066911264, -5.407089921784865361, -7.771874999385531169 ) ) ;
#22384=CARTESIAN_POINT ( 'NONE',  ( 10.31873187879411091, 0.000000000000000000, -2.390624999385526639 ) ) ;
#22390=CARTESIAN_POINT ( 'NONE',  ( 10.56230152254410726, 3.464101615137752166, -0.3749999987710042615 ) ) ;
#22399=CARTESIAN_POINT ( 'NONE',  ( 16.56230152254411436, -6.928203230275514990, -8.437500000000024869 ) ) ;
#22407=LINE ( 'NONE', #22777, #32280 ) ;
#22413=ORIENTED_EDGE ( 'NONE', *, *, #30266, .F. ) ;
#22417=CARTESIAN_POINT ( 'NONE',  ( 16.56230152254411436, -7.209453229046482114, -5.484374999385515537 ) ) ;
#22421=CARTESIAN_POINT ( 'NONE',  ( 19.68408634441912142, -5.407089921784861808, -2.296874999385551064 ) ) ;
#22432=DIRECTION ( 'NONE',  ( 0.000000000000000000, 0.000000000000000000, 1.000000000000000000 ) ) ;
#22440=CARTESIAN_POINT ( 'NONE',  ( 10.56230152254410548, 3.464101615137757051, -2.287500000000039613 ) ) ;
#22453=VERTEX_POINT ( 'NONE', #26962 ) ;
#22458=CARTESIAN_POINT ( 'NONE',  ( 19.68408634441910721, -5.407089921784855591, -8.090624999385564564 ) ) ;
#22467=CARTESIAN_POINT ( 'NONE',  ( 13.56230152254411792, -5.196152422706638241, -4.425000000000068212 ) ) ;
#22474=( BOUNDED_CURVE ( )  B_SPLINE_CURVE ( 2, ( #25609, #37166, #17092, #17653, #34327, #5508, #28631 ),
 .UNSPECIFIED., .F., .F. ) 
 B_SPLINE_CURVE_WITH_KNOTS ( ( 3, 2, 2, 3 ),
 ( 0.8043478260869593166, 0.8115942028985527745, 0.8188405797101460104, 0.8260869565217394683 ),
 .UNSPECIFIED. ) 
 CURVE ( )  GEOMETRIC_REPRESENTATION_ITEM ( )  RATIONAL_B_SPLINE_CURVE ( ( 0.9999999999999487077, 0.8660254037844899999, 1.000000000000000000, 0.8660254037844387076, 1.000000000000000000, 0.8660254037844326014, 1.000000000000006217 ) ) 
 REPRESENTATION_ITEM ( '' )  );
#22492=CARTESIAN_POINT ( 'NONE',  ( 22.56230152254411792, 7.347880794884125653E-16, -0.6750000000000366818 ) ) ;
#22496=CARTESIAN_POINT ( 'NONE',  ( 10.31873187879411091, -3.604726614523240613, -5.953124999385525307 ) ) ;
#22505=CARTESIAN_POINT ( 'NONE',  ( 22.80587116629411426, 3.604726614523243278, -2.184374999385525040 ) ) ;
#22511=CARTESIAN_POINT ( 'NONE',  ( 10.31873187879411091, -3.604726614523240613, -2.353124999385527882 ) ) ;
#22514=CARTESIAN_POINT ( 'NONE',  ( 16.56230152254410726, 0.000000000000000000, -10.00000000000000000 ) ) ;
#22536=CARTESIAN_POINT ( 'NONE',  ( 15.47811703177229070, 6.148715791637015649, -10.19635138606057367 ) ) ;
#22537=CARTESIAN_POINT ( 'NONE',  ( 13.44051670066911086, 5.407089921784862696, -5.671874999385540406 ) ) ;
#22538=CARTESIAN_POINT ( 'NONE',  ( 10.56230152254410903, 0.000000000000000000, -0.4500000000000614619 ) ) ;
#22564=CARTESIAN_POINT ( 'NONE',  ( 10.31873187879411091, -3.604726614523244610, -7.359374999385524418 ) ) ;
#22568=CARTESIAN_POINT ( 'NONE',  ( 19.68408634441910721, -5.407089921784855591, -2.240624999385543159 ) ) ;
#22573=CARTESIAN_POINT ( 'NONE',  ( 16.56230152254411436, -6.928203230275506996, -7.424999998770979381 ) ) ;
#22576=CARTESIAN_POINT ( 'NONE',  ( 19.56230152254410370, 5.196152422706631135, -4.537499998771011178 ) ) ;
#22586=CARTESIAN_POINT ( 'NONE',  ( 16.56230152254411436, -7.209453229046475009, -0.4781249993855187230 ) ) ;
#22588=DIRECTION ( 'NONE',  ( 1.000000000000000000, 0.000000000000000000, 0.000000000000000000 ) ) ;
#22592=CARTESIAN_POINT ( 'NONE',  ( 19.56230152254410370, 5.196152422706631135, -2.287499998770980980 ) ) ;
#22604=CARTESIAN_POINT ( 'NONE',  ( 16.56230152254411081, 7.209453229046482114, -5.709374999385496530 ) ) ;
#22608=CARTESIAN_POINT ( 'NONE',  ( 19.68408634441911076, 5.407089921784862696, -1.246874999385527705 ) ) ;
#22611=CARTESIAN_POINT ( 'NONE',  ( 22.56230152254595112, 3.464101615136682355, -9.524999998771026100 ) ) ;
#22615=PLANE ( 'NONE',  #8501 ) ;
#22628=CARTESIAN_POINT ( 'NONE',  ( 16.56230152254411436, -6.928203230275514990, -1.687500000000023981 ) ) ;
#22634=CARTESIAN_POINT ( 'NONE',  ( 10.56230152254410726, 0.000000000000000000, -6.637499998771001941 ) ) ;
#22645=EDGE_CURVE ( 'NONE', #10703, #205, #27975, .T. ) ;
#22647=CARTESIAN_POINT ( 'NONE',  ( 14.39393254099747743, 5.957544813848095089, -10.12707777273552523 ) ) ;
#22680=CARTESIAN_POINT ( 'NONE',  ( 16.56230152254411792, -6.928203230275514990, -0.7875000000000323963 ) ) ;
#22685=CARTESIAN_POINT ( 'NONE',  ( 10.31873187879411269, 3.604726614523236616, -6.028124999385552130 ) ) ;
#22694=CARTESIAN_POINT ( 'NONE',  ( 22.80587116629411781, -3.604726614523238837, -2.709374999385515181 ) ) ;
#22701=CARTESIAN_POINT ( 'NONE',  ( 16.56230152254411081, -7.209453229046475009, -2.728124999385529215 ) ) ;
#22709=ORIENTED_EDGE ( 'NONE', *, *, #11948, .F. ) ;
#22727=CARTESIAN_POINT ( 'NONE',  ( 22.80587116629411781, -3.604726614523238837, -9.459374999385547156 ) ) ;
#22743=AXIS2_PLACEMENT_3D ( 'NONE', #4505, #16082, #1661 ) ;
#22755=CARTESIAN_POINT ( 'NONE',  ( 22.80587116629410360, -3.604726614523235284, -4.003124999385554439 ) ) ;
#22761=CARTESIAN_POINT ( 'NONE',  ( 13.56230152254411259, -5.196152422706632912, -2.512499998771011711 ) ) ;
#22770=CARTESIAN_POINT ( 'NONE',  ( 10.31873187879411091, -3.604726614523240613, -1.903124999385531924 ) ) ;
#22771=CARTESIAN_POINT ( 'NONE',  ( 22.56230152254563492, 3.464101615136866652, -9.074999998770993059 ) ) ;
#22777=CARTESIAN_POINT ( 'NONE',  ( 10.56230152254410903, 7.347880794884117764E-16, -10.00000000000000000 ) ) ;
#22783=EDGE_LOOP ( 'NONE', ( #17197, #5035, #13980, #11033 ) ) ;
#22786=CARTESIAN_POINT ( 'NONE',  ( 19.68408634441911786, -5.407089921784861808, -8.596874999385523353 ) ) ;
#22791=CARTESIAN_POINT ( 'NONE',  ( 13.44051670066911086, 5.407089921784862696, -0.7218749993855300140 ) ) ;
#22795=CARTESIAN_POINT ( 'NONE',  ( 13.56230152254410726, 5.196152422706630247, -0.4124999987710209481 ) ) ;
#22797=CARTESIAN_POINT ( 'NONE',  ( 16.56230152254411436, 6.928203230275514990, -2.812500000000029310 ) ) ;
#22809=CARTESIAN_POINT ( 'NONE',  ( 10.56230152254411436, -3.464101615137761048, -4.012500000000060574 ) ) ;
#22810=EDGE_CURVE ( 'NONE', #6605, #22453, #12255, .T. ) ;
#22816=CARTESIAN_POINT ( 'NONE',  ( 16.56230152254411081, 6.928203230275514990, -6.412500000000027178 ) ) ;
#22831=CARTESIAN_POINT ( 'NONE',  ( 13.44051670066911086, 5.407089921784862696, -0.7218749993855300140 ) ) ;
#22854=CARTESIAN_POINT ( 'NONE',  ( 22.56230152254410370, 7.347880794884117764E-16, -4.162499998770996967 ) ) ;
#22865=CARTESIAN_POINT ( 'NONE',  ( 10.31873187879411091, 3.604726614523236616, -6.478124999385515004 ) ) ;
#22878=CARTESIAN_POINT ( 'NONE',  ( 19.68408634441910365, 5.407089921784857367, -2.990624999385543603 ) ) ;
#22883=EDGE_LOOP ( 'NONE', ( #27769, #389, #12480, #13801, #3654, #22147, #11451, #23755, #34799, #8143, #31476, #25294, #20360, #21401, #1522, #4083, #21627, #19123, #21090, #29958, #15560, #29795, #4390, #9027, #8326, #34754, #10786, #30674, #35916, #10597, #10691, #27488, #30169, #3803, #24090, #14105, #34197, #16647, #14195, #10912, #34566, #9526, #5189, #24331, #18445, #7591 ) ) ;
#22888=CIRCLE ( 'NONE', #28929, 1.500000000000001332 ) ;
#22898=CARTESIAN_POINT ( 'NONE',  ( 16.56230152254411081, 7.209453229046475009, -9.703124999385543958 ) ) ;
#22900=LINE ( 'NONE', #5442, #37275 ) ;
#22912=CARTESIAN_POINT ( 'NONE',  ( 22.80587116629412137, 7.646167579472024665E-16, -8.521874999385502747 ) ) ;
#22913=CARTESIAN_POINT ( 'NONE',  ( 22.56230152254421384, 3.464101615137700207, -0.1875000000000502653 ) ) ;
#22919=DIRECTION ( 'NONE',  ( 1.000000000000000000, 0.000000000000000000, 0.000000000000000000 ) ) ;
#22926=CARTESIAN_POINT ( 'NONE',  ( 13.56230152254410726, 5.196152422706636465, -4.125000000000045297 ) ) ;
#22935=CARTESIAN_POINT ( 'NONE',  ( 13.56230152254411614, -5.196152422706638241, -2.175000000000065548 ) ) ;
#22942=CARTESIAN_POINT ( 'NONE',  ( 22.80587116629411071, -3.604726614523235284, -2.653124999385503280 ) ) ;
#22947=CARTESIAN_POINT ( 'NONE',  ( 10.56230152254410903, 0.000000000000000000, -3.937499998770993770 ) ) ;
#22973=CARTESIAN_POINT ( 'NONE',  ( 22.80587116629412847, -3.604726614523238837, -9.009374999385519445 ) ) ;
#22977=CARTESIAN_POINT ( 'NONE',  ( 13.44051670066911264, -5.407089921784865361, -1.921874999385508875 ) ) ;
#22993=CARTESIAN_POINT ( 'NONE',  ( 10.56230152254410903, 3.464101615137757051, -4.537500000000050271 ) ) ;
#22994=EDGE_LOOP ( 'NONE', ( #19069, #4747 ) ) ;
#23001=FACE_OUTER_BOUND ( 'NONE', #30782, .T. ) ;
#23009=VERTEX_POINT ( 'NONE', #13416 ) ;
#23011=CARTESIAN_POINT ( 'NONE',  ( 19.68408634441911431, -5.407089921784861808, -0.4968749993855270386 ) ) ;
#23035=EDGE_CURVE ( 'NONE', #31630, #35189, #36622, .T. ) ;
#23049=CARTESIAN_POINT ( 'NONE',  ( 13.44051670066911264, 5.407089921784856479, -8.765624999385545735 ) ) ;
#23050=CARTESIAN_POINT ( 'NONE',  ( 16.56230152254411081, 6.928203230275514990, -8.662500000000004974 ) ) ;
#23061=CARTESIAN_POINT ( 'NONE',  ( 13.44051670066911264, 5.407089921784856479, -3.365624999385530280 ) ) ;
#23070=EDGE_CURVE ( 'NONE', #37311, #26550, #5609, .T. ) ;
#23074=AXIS2_PLACEMENT_3D ( 'NONE', #4604, #16739, #8207 ) ;
#23076=CARTESIAN_POINT ( 'NONE',  ( 10.56230152254410726, 0.000000000000000000, -9.900000000000048317 ) ) ;
#23092=CARTESIAN_POINT ( 'NONE',  ( 22.80587116629411781, 3.604726614523243278, -8.034374999385502036 ) ) ;
#23107=CARTESIAN_POINT ( 'NONE',  ( 8.562301522544109034, 9.797174393178823685E-16, 2.535898384862258492 ) ) ;
#23117=CARTESIAN_POINT ( 'NONE',  ( 13.56230152254411436, -5.196152422706638241, -3.075000000000049916 ) ) ;
#23124=CARTESIAN_POINT ( 'NONE',  ( 16.56230152254411436, 7.209453229046475009, -2.503124999385547778 ) ) ;
#23129=CYLINDRICAL_SURFACE ( 'NONE', #26093, 5.999999999999998224 ) ;
#23131=CARTESIAN_POINT ( 'NONE',  ( 10.56230152254410726, 3.464101615137752166, -3.074999998770978404 ) ) ;
#23138=CARTESIAN_POINT ( 'NONE',  ( 10.56230152254273058, 3.464101615136960355, -8.137500000000033040 ) ) ;
#23159=CARTESIAN_POINT ( 'NONE',  ( 19.68408634441912142, -5.407089921784861808, -7.696874999385511451 ) ) ;
#23164=CARTESIAN_POINT ( 'NONE',  ( 10.31873187879410736, 0.000000000000000000, -2.896874999385512517 ) ) ;
#23180=CARTESIAN_POINT ( 'NONE',  ( 16.56230152254411436, -6.928203230275514990, -3.487500000000039346 ) ) ;
#23186=CIRCLE ( 'NONE', #21397, 5.999999999999998224 ) ;
#23199=CARTESIAN_POINT ( 'NONE',  ( 19.68408634441911076, 5.407089921784862696, -1.696874999385505900 ) ) ;
#23225=FACE_OUTER_BOUND ( 'NONE', #912, .T. ) ;
#23232=CARTESIAN_POINT ( 'NONE',  ( 10.31873187879411091, 3.604726614523236616, -10.07812499938551198 ) ) ;
#23235=CARTESIAN_POINT ( 'NONE',  ( 10.53852972689264433, -1.498109391770361842, -10.00000000000000355 ) ) ;
#23242=ORIENTED_EDGE ( 'NONE', *, *, #9647, .F. ) ;
#23247=CARTESIAN_POINT ( 'NONE',  ( 10.31873187879411091, 3.604726614523236616, -5.578124999385555505 ) ) ;
#23253=ORIENTED_EDGE ( 'NONE', *, *, #25713, .F. ) ;
#23275=CARTESIAN_POINT ( 'NONE',  ( 16.56230152254411081, -6.928203230275506996, -8.324999998771003717 ) ) ;
#23276=ADVANCED_FACE ( 'NONE', ( #5986 ), #17566, .F. ) ;
#23280=CARTESIAN_POINT ( 'NONE',  ( 13.44051670066910908, 5.407089921784862696, -8.821874999385526550 ) ) ;
#23283=DIRECTION ( 'NONE',  ( 0.000000000000000000, 0.000000000000000000, 1.000000000000000000 ) ) ;
#23286=CYLINDRICAL_SURFACE ( 'NONE', #5753, 5.999999999999998224 ) ;
#23294=CARTESIAN_POINT ( 'NONE',  ( 13.56230152254410548, 5.196152422706636465, -9.075000000000027711 ) ) ;
#23299=ORIENTED_EDGE ( 'NONE', *, *, #31874, .F. ) ;
#23300=EDGE_LOOP ( 'NONE', ( #3441, #20415, #14666, #26353 ) ) ;
#23309=CARTESIAN_POINT ( 'NONE',  ( 19.68408634441910721, 5.407089921784857367, -5.690624999385579308 ) ) ;
#23314=CARTESIAN_POINT ( 'NONE',  ( 22.56230152254410370, 3.464101615137755275, -3.224999998770998744 ) ) ;
#23328=DIRECTION ( 'NONE',  ( 0.000000000000000000, 0.000000000000000000, 1.000000000000000000 ) ) ;
#23333=CARTESIAN_POINT ( 'NONE',  ( 10.56230152254332033, -3.464101615137297419, -5.699999998771033916 ) ) ;
#23340=CARTESIAN_POINT ( 'NONE',  ( 22.80587116629412137, 7.646167579472024665E-16, -8.971874999385509142 ) ) ;
#23344=CARTESIAN_POINT ( 'NONE',  ( 16.56230152254411436, 7.209453229046482114, -4.809374999385505944 ) ) ;
#23348=( BOUNDED_CURVE ( )  B_SPLINE_CURVE ( 2, ( #13406, #14149, #24955, #36513, #22134, #7720, #27990 ),
 .UNSPECIFIED., .F., .F. ) 
 B_SPLINE_CURVE_WITH_KNOTS ( ( 3, 2, 2, 3 ),
 ( 0.6521739130434790477, 0.6594202898550725056, 0.6666666666666657415, 0.6739130434782591994 ),
 .UNSPECIFIED. ) 
 CURVE ( )  GEOMETRIC_REPRESENTATION_ITEM ( )  RATIONAL_B_SPLINE_CURVE ( ( 0.9999999999999856781, 0.8660254037844530295, 1.000000000000000000, 0.8660254037844387076, 1.000000000000000000, 0.8660254037844694608, 0.9999999999999692468 ) ) 
 REPRESENTATION_ITEM ( '' )  );
#23363=CARTESIAN_POINT ( 'NONE',  ( 16.56230152254411081, -6.928203230275514990, -5.287500000000021849 ) ) ;
#23381=CARTESIAN_POINT ( 'NONE',  ( 10.31873187879410558, 0.000000000000000000, -1.546874999385550176 ) ) ;
#23387=VERTEX_POINT ( 'NONE', #23430 ) ;
#23393=AXIS2_PLACEMENT_3D ( 'NONE', #34, #34718, #16743 ) ;
#23407=DIRECTION ( 'NONE',  ( 1.000000000000000000, 0.000000000000000000, 0.000000000000000000 ) ) ;
#23414=LINE ( 'NONE', #8137, #6040 ) ;
#23415=CARTESIAN_POINT ( 'NONE',  ( 16.56230152254411081, 7.209453229046475009, -9.703124999385542182 ) ) ;
#23427=CARTESIAN_POINT ( 'NONE',  ( 16.56230152254411081, 7.209453229046475009, -3.403124999385538807 ) ) ;
#23430=CARTESIAN_POINT ( 'NONE',  ( 22.56230152254410015, 7.347880794884117764E-16, -8.212499998771022547 ) ) ;
#23436=CARTESIAN_POINT ( 'NONE',  ( 10.31873187879411091, 0.000000000000000000, -0.1406249993855246405 ) ) ;
#23443=CARTESIAN_POINT ( 'NONE',  ( 16.56230152254410726, 0.000000000000000000, -10.00000000000000000 ) ) ;
#23459=CARTESIAN_POINT ( 'NONE',  ( 19.68408634441912142, -5.407089921784861808, -7.696874999385511451 ) ) ;
#23461=CARTESIAN_POINT ( 'NONE',  ( 10.31873187879411269, -3.604726614523240613, -1.003124999385540450 ) ) ;
#23490=CARTESIAN_POINT ( 'NONE',  ( 16.56230152254411436, 7.209453229046475009, -4.753124999385526017 ) ) ;
#23495=CARTESIAN_POINT ( 'NONE',  ( 22.56230152254410370, 7.347880794884117764E-16, -1.462499998771016330 ) ) ;
#23497=CARTESIAN_POINT ( 'NONE',  ( 19.56230152254411081, -5.196152422706629359, -5.587499998771034093 ) ) ;
#23498=ADVANCED_FACE ( 'NONE', ( #6635 ), #18396, .F. ) ;
#23518=CARTESIAN_POINT ( 'NONE',  ( 22.46128102716605923, 1.096376214649937619, -10.00000000000000000 ) ) ;
#23531=ORIENTED_EDGE ( 'NONE', *, *, #32387, .F. ) ;
#23532=CARTESIAN_POINT ( 'NONE',  ( 22.80587116629411781, -3.604726614523238837, -4.509374999385530103 ) ) ;
#23535=EDGE_CURVE ( 'NONE', #12454, #29192, #13927, .T. ) ;
#23537=EDGE_CURVE ( 'NONE', #37311, #26963, #26523, .T. ) ;
#23545=ORIENTED_EDGE ( 'NONE', *, *, #12616, .T. ) ;
#23553=CARTESIAN_POINT ( 'NONE',  ( 10.56230152254411259, -3.464101615137761048, -5.362500000000047784 ) ) ;
#23556=CARTESIAN_POINT ( 'NONE',  ( 13.56230152254410370, 5.196152422706630247, -5.362499998771003362 ) ) ;
#23570=CARTESIAN_POINT ( 'NONE',  ( 22.80587116629411426, 7.646167579472024665E-16, -2.221874999385531346 ) ) ;
#23601=CARTESIAN_POINT ( 'NONE',  ( 19.68408634441910721, 5.407089921784857367, -8.390624999385531524 ) ) ;
#23613=B_SPLINE_CURVE_WITH_KNOTS ( 'NONE', 1,
 ( #29561, #21241 ),
 .UNSPECIFIED., .F., .F.,
 ( 2, 2 ),
 ( 0.000000000000000000, 1.000000000000000000 ),
 .UNSPECIFIED. ) ;
#23615=CARTESIAN_POINT ( 'NONE',  ( 10.31873187879411091, 0.000000000000000000, -5.090624999385534366 ) ) ;
#23632=DIRECTION ( 'NONE',  ( 0.000000000000000000, 0.000000000000000000, 1.000000000000000000 ) ) ;
#23652=CARTESIAN_POINT ( 'NONE',  ( 22.80587116629410716, 7.646167579472015790E-16, -0.8156249993855335667 ) ) ;
#23658=CARTESIAN_POINT ( 'NONE',  ( 10.31873187879410914, 0.000000000000000000, -0.1968749993855323233 ) ) ;
#23680=CARTESIAN_POINT ( 'NONE',  ( 10.31873187879410914, 0.000000000000000000, -5.990624999385518734 ) ) ;
#23686=CARTESIAN_POINT ( 'NONE',  ( 22.56230152254410015, 3.464101615137755275, -5.474999998770977427 ) ) ;
#23692=CARTESIAN_POINT ( 'NONE',  ( 19.68408634441911076, 5.407089921784862696, -3.496874999385557459 ) ) ;
#23694=CARTESIAN_POINT ( 'NONE',  ( 19.56230152254410370, 5.196152422706631135, -7.237499998771018461 ) ) ;
#23706=CARTESIAN_POINT ( 'NONE',  ( 22.56230152254505228, -3.464101615137219259, -4.762500000000051692 ) ) ;
#23713=ORIENTED_EDGE ( 'NONE', *, *, #35777, .F. ) ;
#23716=AXIS2_PLACEMENT_3D ( 'NONE', #17502, #34549, #20160 ) ;
#23723=CARTESIAN_POINT ( 'NONE',  ( 19.68408634441911076, 5.407089921784862696, -3.946874999385563410 ) ) ;
#23741=CARTESIAN_POINT ( 'NONE',  ( 13.56230152254410548, 5.196152422706636465, -6.825000000000025935 ) ) ;
#23745=CARTESIAN_POINT ( 'NONE',  ( 10.56230152254411081, 0.000000000000000000, -5.287499998771011178 ) ) ;
#23748=FACE_OUTER_BOUND ( 'NONE', #16819, .T. ) ;
#23749=CARTESIAN_POINT ( 'NONE',  ( 22.17721121674838614, -2.360623836386564811, -10.00000000000000178 ) ) ;
#23755=ORIENTED_EDGE ( 'NONE', *, *, #33797, .T. ) ;
#23758=CARTESIAN_POINT ( 'NONE',  ( 19.68408634441912142, -5.407089921784861808, -3.646874999385540939 ) ) ;
#23766=CARTESIAN_POINT ( 'NONE',  ( 19.56230152254412147, 5.196152422706637353, -1.050000000000023137 ) ) ;
#23778=( BOUNDED_CURVE ( )  B_SPLINE_CURVE ( 2, ( #3709, #35548, #2633, #34480, #22935, #37314, #26833 ),
 .UNSPECIFIED., .F., .F. ) 
 B_SPLINE_CURVE_WITH_KNOTS ( ( 3, 2, 2, 3 ),
 ( 0.1956521739130406834, 0.2028985507246359177, 0.2101449275362311242, 0.2173913043478263585 ),
 .UNSPECIFIED. ) 
 CURVE ( )  GEOMETRIC_REPRESENTATION_ITEM ( )  RATIONAL_B_SPLINE_CURVE ( ( 1.000000000000051736, 0.8660254037843868602, 1.000000000000000000, 0.8660254037844387076, 1.000000000000000000, 0.8660254037844336006, 1.000000000000005107 ) ) 
 REPRESENTATION_ITEM ( '' )  );
#23787=CARTESIAN_POINT ( 'NONE',  ( 19.56230152254412147, -5.196152422706635576, -0.7500000000000839329 ) ) ;
#23791=CARTESIAN_POINT ( 'NONE',  ( 22.80587116629411071, -3.604726614523235284, -9.853124999385531879 ) ) ;
#23794=CARTESIAN_POINT ( 'NONE',  ( 10.74238581874539022, 1.953770193659143395, -10.00000000000000178 ) ) ;
#23804=CARTESIAN_POINT ( 'NONE',  ( 16.56230152254411081, 7.209453229046475009, -4.303124999385498306 ) ) ;
#23841=ADVANCED_FACE ( 'NONE', ( #20261 ), #2248, .T. ) ;
#23842=CARTESIAN_POINT ( 'NONE',  ( 19.68408634441910721, 5.407089921784857367, -0.7406249993855418268 ) ) ;
#23844=DIRECTION ( 'NONE',  ( 0.000000000000000000, 0.000000000000000000, 1.000000000000000000 ) ) ;
#23847=EDGE_CURVE ( 'NONE', #11542, #13979, #31071, .T. ) ;
#23873=CARTESIAN_POINT ( 'NONE',  ( 10.31873187879411269, 3.604726614523236616, -4.228124999385537208 ) ) ;
#23878=CARTESIAN_POINT ( 'NONE',  ( 16.56230152254410726, 0.000000000000000000, -10.00000000000000000 ) ) ;
#23880=CARTESIAN_POINT ( 'NONE',  ( 22.56230152254411081, -3.464101615137751278, -6.899999998771022547 ) ) ;
#23885=CARTESIAN_POINT ( 'NONE',  ( 16.56230152254411081, 7.209453229046482114, -3.909374999385482496 ) ) ;
#23899=CARTESIAN_POINT ( 'NONE',  ( 16.56230152254411081, 6.928203230275506996, -5.849999998771011178 ) ) ;
#23914=CARTESIAN_POINT ( 'NONE',  ( 22.80587116629411781, 3.604726614523243278, -4.434374999385503280 ) ) ;
#23932=CARTESIAN_POINT ( 'NONE',  ( 16.56230152254411081, -6.928203230275514990, -6.187500000000013323 ) ) ;
#23936=CARTESIAN_POINT ( 'NONE',  ( 10.56230152254410903, 0.000000000000000000, -6.187499998771023080 ) ) ;
#23942=CARTESIAN_POINT ( 'NONE',  ( 16.56230152254410726, 0.000000000000000000, -10.00000000000000000 ) ) ;
#23949=CARTESIAN_POINT ( 'NONE',  ( 10.31873187879410558, 3.604726614523240613, -2.934374999385496618 ) ) ;
#23960=EDGE_CURVE ( 'NONE', #31128, #17848, #14916, .T. ) ;
#23962=CARTESIAN_POINT ( 'NONE',  ( 13.44051670066911086, 5.407089921784856479, -0.2156249993855441360 ) ) ;
#23978=CARTESIAN_POINT ( 'NONE',  ( 10.56230152254410726, 0.000000000000000000, -3.150000000000041656 ) ) ;
#23984=CARTESIAN_POINT ( 'NONE',  ( 10.56230152254410726, 0.000000000000000000, -7.650000000000045652 ) ) ;
#23991=ORIENTED_EDGE ( 'NONE', *, *, #12882, .T. ) ;
#23994=CARTESIAN_POINT ( 'NONE',  ( 16.56230152254411081, -7.209453229046475009, -7.678124999385515181 ) ) ;
#23996=CARTESIAN_POINT ( 'NONE',  ( 10.56230152254273413, -3.464101615136960355, -2.549999998771006471 ) ) ;
#23999=VERTEX_POINT ( 'NONE', #28955 ) ;
#24002=CARTESIAN_POINT ( 'NONE',  ( 10.56230152254410548, 0.000000000000000000, -4.050000000000054001 ) ) ;
#24022=ADVANCED_FACE ( 'NONE', ( #29330 ), #23286, .F. ) ;
#24030=CARTESIAN_POINT ( 'NONE',  ( 10.31873187879411091, 0.000000000000000000, -5.090624999385534366 ) ) ;
#24059=CARTESIAN_POINT ( 'NONE',  ( 10.31873187879410736, -3.604726614523240613, -5.053124999385534721 ) ) ;
#24066=CARTESIAN_POINT ( 'NONE',  ( 16.56230152254411081, 6.928203230275506996, -7.199999998770998388 ) ) ;
#24070=CARTESIAN_POINT ( 'NONE',  ( 10.31873187879410736, 0.000000000000000000, -5.146874999385541827 ) ) ;
#24089=ORIENTED_EDGE ( 'NONE', *, *, #35141, .F. ) ;
#24090=ORIENTED_EDGE ( 'NONE', *, *, #16832, .T. ) ;
#24099=CARTESIAN_POINT ( 'NONE',  ( 19.68408634441911431, 5.407089921784862696, -5.296874999385526195 ) ) ;
#24121=CARTESIAN_POINT ( 'NONE',  ( 13.56230152254411792, -5.196152422706638241, -7.125000000000075495 ) ) ;
#24123=CARTESIAN_POINT ( 'NONE',  ( 22.56230152254412502, 7.347880794884125653E-16, -3.375000000000044409 ) ) ;
#24125=CARTESIAN_POINT ( 'NONE',  ( 22.56230152254410370, 8.572527594031469245E-16, 10.00000000000000000 ) ) ;
#24128=DIRECTION ( 'NONE',  ( 1.000000000000000000, 0.000000000000000000, 0.000000000000000000 ) ) ;
#24136=ORIENTED_EDGE ( 'NONE', *, *, #26746, .F. ) ;
#24139=CARTESIAN_POINT ( 'NONE',  ( 19.68408634441912142, -5.407089921784861808, -3.196874999385534988 ) ) ;
#24154=CARTESIAN_POINT ( 'NONE',  ( 13.56230152254410726, 5.196152422706630247, -0.8624999987709991434 ) ) ;
#24160=CARTESIAN_POINT ( 'NONE',  ( 10.56230152254410726, 3.464101615137757051, -0.9375000000000204281 ) ) ;
#24178=CARTESIAN_POINT ( 'NONE',  ( 19.68408634441910721, 5.407089921784857367, -7.040624999385541649 ) ) ;
#24214=CARTESIAN_POINT ( 'NONE',  ( 16.56230152254410726, 7.209453229046475009, -5.203124999385489780 ) ) ;
#24218=CARTESIAN_POINT ( 'NONE',  ( 16.56230152254411436, -7.209453229046482114, -9.534374999385541116 ) ) ;
#24227=CARTESIAN_POINT ( 'NONE',  ( 10.56230152254410548, 0.000000000000000000, -6.750000000000061284 ) ) ;
#24235=ORIENTED_EDGE ( 'NONE', *, *, #28917, .F. ) ;
#24248=CARTESIAN_POINT ( 'NONE',  ( 13.44051670066911441, -5.407089921784859143, -8.165624999385528326 ) ) ;
#24252=DIRECTION ( 'NONE',  ( 0.000000000000000000, 0.000000000000000000, 1.000000000000000000 ) ) ;
#24253=VECTOR ( 'NONE', #9678, 1000.000000000000000 ) ;
#24255=CARTESIAN_POINT ( 'NONE',  ( 10.56230152254411081, 0.000000000000000000, -5.287499998771011178 ) ) ;
#24256=EDGE_CURVE ( 'NONE', #17042, #31449, #6159, .T. ) ;
#24257=LINE ( 'NONE', #1119, #19561 ) ;
#24259=CARTESIAN_POINT ( 'NONE',  ( 16.56230152254411436, -7.209453229046482114, -4.134374999385496352 ) ) ;
#24276=CARTESIAN_POINT ( 'NONE',  ( 10.31873187879410736, 3.604726614523236616, -0.1781249993854788494 ) ) ;
#24288=CARTESIAN_POINT ( 'NONE',  ( 22.80587116629411781, -3.604726614523238837, -7.209374999385536498 ) ) ;
#24309=CARTESIAN_POINT ( 'NONE',  ( 22.56230152254412147, -3.464101615137755275, -7.462500000000038547 ) ) ;
#24313=CARTESIAN_POINT ( 'NONE',  ( 13.56230152254411436, -5.196152422706632912, -6.112499998771031784 ) ) ;
#24318=CARTESIAN_POINT ( 'NONE',  ( 10.56230152254410726, 0.000000000000000000, -5.400000000000043876 ) ) ;
#24326=CARTESIAN_POINT ( 'NONE',  ( 19.68408634441911786, -5.407089921784861808, -4.546874999385525307 ) ) ;
#24331=ORIENTED_EDGE ( 'NONE', *, *, #15931, .T. ) ;
#24350=CARTESIAN_POINT ( 'NONE',  ( 19.56230152254410370, 5.196152422706631135, -9.937499998770999099 ) ) ;
#24353=EDGE_LOOP ( 'NONE', ( #26012, #8405, #5065, #2582 ) ) ;
#24356=DIRECTION ( 'NONE',  ( -0.000000000000000000, -0.000000000000000000, -1.000000000000000000 ) ) ;
#24363=ORIENTED_EDGE ( 'NONE', *, *, #23535, .F. ) ;
#24366=CARTESIAN_POINT ( 'NONE',  ( 19.68408634441910721, -5.407089921784855591, -7.190624999385525129 ) ) ;
#24372=ORIENTED_EDGE ( 'NONE', *, *, #10112, .F. ) ;
#24376=CARTESIAN_POINT ( 'NONE',  ( 22.56230152254412147, 7.347880794884125653E-16, -9.225000000000010303 ) ) ;
#24401=CARTESIAN_POINT ( 'NONE',  ( 16.56230152254411436, 7.209453229046475009, -4.753124999385526017 ) ) ;
#24403=CARTESIAN_POINT ( 'NONE',  ( 16.56230152254410726, 0.000000000000000000, -10.00000000000000000 ) ) ;
#24415=CARTESIAN_POINT ( 'NONE',  ( 13.56230152254411792, -5.196152422706638241, -6.675000000000069988 ) ) ;
#24433=CARTESIAN_POINT ( 'NONE',  ( 22.80587116629410716, 3.604726614523238837, -6.628124999385534899 ) ) ;
#24439=CARTESIAN_POINT ( 'NONE',  ( 22.56230152254412147, -3.464101615137751278, -8.249999998771009757 ) ) ;
#24443=CARTESIAN_POINT ( 'NONE',  ( 19.68408634441911786, -5.407089921784861808, -4.096874999385518912 ) ) ;
#24460=CARTESIAN_POINT ( 'NONE',  ( 22.80587116629410716, 3.604726614523238837, -1.678124999385518068 ) ) ;
#24466=( GEOMETRIC_REPRESENTATION_CONTEXT ( 3 ) GLOBAL_UNCERTAINTY_ASSIGNED_CONTEXT ( ( #29713 ) ) GLOBAL_UNIT_ASSIGNED_CONTEXT ( ( #36211, #1721, #36586 ) ) REPRESENTATION_CONTEXT ( 'NONE', 'WORKASPACE' ) );
#24474=CARTESIAN_POINT ( 'NONE',  ( 10.31873187879410736, -3.604726614523244610, -6.009374999385536320 ) ) ;
#24494=CARTESIAN_POINT ( 'NONE',  ( 19.56230152254412147, 5.196152422706637353, -6.900000000000044764 ) ) ;
#24509=CARTESIAN_POINT ( 'NONE',  ( 22.80587116629411781, 7.646167579472024665E-16, -4.921874999385511984 ) ) ;
#24513=ORIENTED_EDGE ( 'NONE', *, *, #26495, .F. ) ;
#24531=CARTESIAN_POINT ( 'NONE',  ( 10.56230152254410726, 3.464101615137757051, -0.4875000000000247469 ) ) ;
#24548=CARTESIAN_POINT ( 'NONE',  ( 13.44051670066911086, 5.407089921784856479, -6.515624999385543958 ) ) ;
#24550=( BOUNDED_CURVE ( )  B_SPLINE_CURVE ( 2, ( #18993, #5122, #31101, #22573, #33937, #25028, #4755 ),
 .UNSPECIFIED., .F., .F. ) 
 B_SPLINE_CURVE_WITH_KNOTS ( ( 3, 2, 2, 3 ),
 ( 0.6739130434782617529, 0.6811594202898560990, 0.6884057971014503341, 0.6956521739130446802 ),
 .UNSPECIFIED. ) 
 CURVE ( )  GEOMETRIC_REPRESENTATION_ITEM ( )  RATIONAL_B_SPLINE_CURVE ( ( 0.9999999999999835687, 0.8660254037844551389, 1.000000000000000000, 0.8660254037844387076, 1.000000000000000000, 0.8660254037844161701, 1.000000000000022649 ) ) 
 REPRESENTATION_ITEM ( '' )  );
#24570=ADVANCED_FACE ( 'NONE', ( #32978 ), #9676, .F. ) ;
#24577=ORIENTED_EDGE ( 'NONE', *, *, #19662, .F. ) ;
#24584=CARTESIAN_POINT ( 'NONE',  ( 19.68408634441910721, 5.407089921784857367, -3.890624999385555505 ) ) ;
#24593=CARTESIAN_POINT ( 'NONE',  ( 22.56230152254277499, 3.464101615138533763, -1.987500000000047118 ) ) ;
#24617=CARTESIAN_POINT ( 'NONE',  ( 22.80587116629410360, 7.646167579472015790E-16, -6.665624999385527438 ) ) ;
#24622=CARTESIAN_POINT ( 'NONE',  ( 13.56230152254410548, 5.196152422706630247, -8.962499998770995902 ) ) ;
#24625=CARTESIAN_POINT ( 'NONE',  ( 22.80587116629411426, 7.646167579472024665E-16, -6.271874999385529392 ) ) ;
#24651=CARTESIAN_POINT ( 'NONE',  ( 10.31873187879410736, -3.604726614523244610, -5.559374999385508609 ) ) ;
#24655=CARTESIAN_POINT ( 'NONE',  ( 10.31873187879410914, 0.000000000000000000, -1.490624999385542493 ) ) ;
#24663=CARTESIAN_POINT ( 'NONE',  ( 10.56230152254410903, -3.464101615137757051, -2.099999998770993415 ) ) ;
#24665=VERTEX_POINT ( 'NONE', #15366 ) ;
#24672=CARTESIAN_POINT ( 'NONE',  ( 10.56230152254410903, -3.464101615137761048, -8.512500000000050804 ) ) ;
#24674=CARTESIAN_POINT ( 'NONE',  ( 22.56230152254411792, 7.347880794884125653E-16, -7.875000000000048850 ) ) ;
#24679=DIRECTION ( 'NONE',  ( 0.000000000000000000, 0.000000000000000000, 1.000000000000000000 ) ) ;
#24681=LINE ( 'NONE', #16165, #28310 ) ;
#24682=CARTESIAN_POINT ( 'NONE',  ( 22.56230152254412147, 7.347880794884125653E-16, -3.825000000000050804 ) ) ;
#24687=EDGE_CURVE ( 'NONE', #28127, #13088, #30333, .T. ) ;
#24688=CARTESIAN_POINT ( 'NONE',  ( 10.31873187879410736, 3.604726614523240613, -7.434374999385486404 ) ) ;
#24704=VECTOR ( 'NONE', #23328, 1000.000000000000000 ) ;
#24712=CARTESIAN_POINT ( 'NONE',  ( 22.56230152254412147, -3.464101615137755275, -2.962500000000017675 ) ) ;
#24730=CARTESIAN_POINT ( 'NONE',  ( 10.31873187879410736, 0.000000000000000000, -6.440624999385525129 ) ) ;
#24738=EDGE_LOOP ( 'NONE', ( #17801, #15277, #9639, #26592 ) ) ;
#24749=LINE ( 'NONE', #5025, #16003 ) ;
#24766=CARTESIAN_POINT ( 'NONE',  ( 22.80587116629410360, 3.604726614523238837, -4.828124999385519978 ) ) ;
#24777=CARTESIAN_POINT ( 'NONE',  ( 22.80587116629411781, 7.646167579472024665E-16, -1.321874999385519445 ) ) ;
#24799=CARTESIAN_POINT ( 'NONE',  ( 16.56230152254410726, -7.209453229046475009, -6.778124999385522820 ) ) ;
#24804=CARTESIAN_POINT ( 'NONE',  ( 13.56230152254411259, -5.196152422706632912, -8.812499998771039955 ) ) ;
#24808=CARTESIAN_POINT ( 'NONE',  ( 22.80587116629411426, 3.604726614523243278, -7.134374999385543425 ) ) ;
#24824=CARTESIAN_POINT ( 'NONE',  ( 22.56230152254410370, 7.347880794884117764E-16, -6.862499998771004250 ) ) ;
#24827=VERTEX_POINT ( 'NONE', #29049 ) ;
#24828=EDGE_LOOP ( 'NONE', ( #19124, #3634, #4267, #29221 ) ) ;
#24837=CARTESIAN_POINT ( 'NONE',  ( 13.44051670066911264, -5.407089921784865361, -5.971874999385562433 ) ) ;
#24842=CARTESIAN_POINT ( 'NONE',  ( 10.31873187879411091, 3.604726614523236616, -1.078124999385534410 ) ) ;
#24846=FILL_AREA_STYLE ('',( #19879 ) ) ;
#24851=CARTESIAN_POINT ( 'NONE',  ( 13.56230152254410726, 5.196152422706630247, -0.8624999987709991434 ) ) ;
#24860=CARTESIAN_POINT ( 'NONE',  ( 22.56230152254411792, 7.347880794884125653E-16, -9.675000000000045119 ) ) ;
#24861=ORIENTED_EDGE ( 'NONE', *, *, #19120, .T. ) ;
#24862=CARTESIAN_POINT ( 'NONE',  ( 10.56230152254549104, -3.464101615138557300, -8.062500000000003553 ) ) ;
#24876=CARTESIAN_POINT ( 'NONE',  ( 19.68408634441911431, 5.407089921784862696, -7.096874999385549998 ) ) ;
#24882=ORIENTED_EDGE ( 'NONE', *, *, #128, .F. ) ;
#24888=CARTESIAN_POINT ( 'NONE',  ( 16.56230152254411792, 6.928203230275514990, -9.562500000000060396 ) ) ;
#24893=CARTESIAN_POINT ( 'NONE',  ( 16.56230152254411081, 6.928203230275506996, -1.799999998770985377 ) ) ;
#24894=CARTESIAN_POINT ( 'NONE',  ( 10.56230152254410726, 0.000000000000000000, -6.300000000000055778 ) ) ;
#24899=CARTESIAN_POINT ( 'NONE',  ( 22.56230152254412147, 3.464101615137759271, -1.087500000000040323 ) ) ;
#24911=ORIENTED_EDGE ( 'NONE', *, *, #1847, .F. ) ;
#24915=CARTESIAN_POINT ( 'NONE',  ( 19.68408634441910365, 5.407089921784857367, -9.290624999385570959 ) ) ;
#24948=CARTESIAN_POINT ( 'NONE',  ( 22.80587116629410716, 3.604726614523238837, -6.628124999385534899 ) ) ;
#24954=CARTESIAN_POINT ( 'NONE',  ( 19.56230152254412502, -5.196152422706635576, -8.400000000000073186 ) ) ;
#24955=CARTESIAN_POINT ( 'NONE',  ( 13.56230152254410548, 5.196152422706636465, -6.825000000000025935 ) ) ;
#24957=CARTESIAN_POINT ( 'NONE',  ( 19.68408634441911431, 5.407089921784862696, -0.7968749993855217539 ) ) ;
#24977=CARTESIAN_POINT ( 'NONE',  ( 22.80587116629410716, 3.604726614523238837, -7.978124999385491023 ) ) ;
#24983=( BOUNDED_CURVE ( )  B_SPLINE_CURVE ( 2, ( #27253, #12472, #32369, #32747, #24415, #901, #24227 ),
 .UNSPECIFIED., .F., .F. ) 
 B_SPLINE_CURVE_WITH_KNOTS ( ( 3, 2, 2, 3 ),
 ( 0.6304347826086960094, 0.6376811594202902445, 0.6449275362318847016, 0.6521739130434790477 ),
 .UNSPECIFIED. ) 
 CURVE ( )  GEOMETRIC_REPRESENTATION_ITEM ( )  RATIONAL_B_SPLINE_CURVE ( ( 0.9999999999999938938, 0.8660254037844448138, 1.000000000000000000, 0.8660254037844387076, 1.000000000000000000, 0.8660254037844243857, 1.000000000000014433 ) ) 
 REPRESENTATION_ITEM ( '' )  );
#24985=CARTESIAN_POINT ( 'NONE',  ( 22.56230152254410370, 3.464101615137755275, -8.174999998770983822 ) ) ;
#24987=DIRECTION ( 'NONE',  ( 0.000000000000000000, 0.000000000000000000, 1.000000000000000000 ) ) ;
#24991=CARTESIAN_POINT ( 'NONE',  ( 10.31873187879411091, -3.604726614523244610, -7.359374999385524418 ) ) ;
#24993=DIRECTION ( 'NONE',  ( 0.000000000000000000, 0.000000000000000000, 1.000000000000000000 ) ) ;
#24995=CARTESIAN_POINT ( 'NONE',  ( 13.56230152254410726, 5.196152422706636465, -5.925000000000041567 ) ) ;
#25009=( BOUNDED_CURVE ( )  B_SPLINE_CURVE ( 2, ( #6196, #11881, #29311, #14919, #26468, #501, #12449 ),
 .UNSPECIFIED., .F., .F. ) 
 B_SPLINE_CURVE_WITH_KNOTS ( ( 3, 2, 2, 3 ),
 ( 0.3913043478260868069, 0.3985507246376819857, 0.4057971014492771644, 0.4130434782608723432 ),
 .UNSPECIFIED. ) 
 CURVE ( )  GEOMETRIC_REPRESENTATION_ITEM ( )  RATIONAL_B_SPLINE_CURVE ( ( 1.000000000000003109, 0.8660254037844357100, 1.000000000000000000, 0.8660254037844387076, 1.000000000000000000, 0.8660254037843874153, 1.000000000000051292 ) ) 
 REPRESENTATION_ITEM ( '' )  );
#25019=CARTESIAN_POINT ( 'NONE',  ( 16.56230152254411436, 6.928203230275514990, -2.362500000000002043 ) ) ;
#25021=CARTESIAN_POINT ( 'NONE',  ( 10.31873187879410736, 3.604726614523240613, -8.334374999385541827 ) ) ;
#25025=CARTESIAN_POINT ( 'NONE',  ( 19.68408634441911076, -5.407089921784855591, -1.340624999385559013 ) ) ;
#25028=CARTESIAN_POINT ( 'NONE',  ( 10.56230152254352461, -3.464101615137419543, -7.499999998771012422 ) ) ;
#25031=CARTESIAN_POINT ( 'NONE',  ( 19.56230152254411081, -5.196152422706629359, -0.6374999987710516791 ) ) ;
#25041=CARTESIAN_POINT ( 'NONE',  ( 10.56230152254410726, 3.464101615137757051, -9.937500000000000000 ) ) ;
#25043=CARTESIAN_POINT ( 'NONE',  ( 19.56230152254412502, -5.196152422706635576, -3.450000000000091660 ) ) ;
#25060=CARTESIAN_POINT ( 'NONE',  ( 10.31873187879410736, 0.000000000000000000, -7.396874999385516958 ) ) ;
#25065=CARTESIAN_POINT ( 'NONE',  ( 10.31873187879410736, 3.604726614523240613, -1.584374999385509630 ) ) ;
#25072=CARTESIAN_POINT ( 'NONE',  ( 22.56230152254411792, 7.347880794884125653E-16, -9.675000000000045119 ) ) ;
#25076=CARTESIAN_POINT ( 'NONE',  ( 22.56230152254410370, 7.347880794884117764E-16, -1.912499998771022280 ) ) ;
#25077=CARTESIAN_POINT ( 'NONE',  ( 16.56230152254411081, -6.928203230275514990, -6.187500000000013323 ) ) ;
#25081=CARTESIAN_POINT ( 'NONE',  ( 16.56230152254411436, 6.928203230275514990, -8.212500000000009237 ) ) ;
#25084=CARTESIAN_POINT ( 'NONE',  ( 16.56230152254411436, 6.928203230275514990, -1.012500000000046585 ) ) ;
#25101=CARTESIAN_POINT ( 'NONE',  ( 13.44051670066911264, 5.407089921784856479, -8.765624999385545735 ) ) ;
#25113=CARTESIAN_POINT ( 'NONE',  ( 10.56230152254410903, 7.347880794884117764E-16, -10.00000000000000000 ) ) ;
#25131=ADVANCED_FACE ( 'NONE', ( #6182 ), #9778, .F. ) ;
#25141=CARTESIAN_POINT ( 'NONE',  ( 10.31873187879411091, 3.604726614523236616, -7.378124999385539340 ) ) ;
#25143=CARTESIAN_POINT ( 'NONE',  ( 16.56230152254411436, -6.928203230275514990, -7.537500000000000533 ) ) ;
#25150=CARTESIAN_POINT ( 'NONE',  ( 10.31873187879410736, -3.604726614523244610, -1.959374999385511407 ) ) ;
#25156=CARTESIAN_POINT ( 'NONE',  ( 16.56230152254411436, -7.209453229046475009, -1.378124999385542226 ) ) ;
#25181=CARTESIAN_POINT ( 'NONE',  ( 22.56230152254411436, -3.464101615137751278, -9.599999998771028942 ) ) ;
#25184=CARTESIAN_POINT ( 'NONE',  ( 10.31873187879410558, -3.604726614523244610, -10.05937499938549884 ) ) ;
#25185=CARTESIAN_POINT ( 'NONE',  ( 10.31873187879410558, 3.604726614523240613, -5.634374999385534544 ) ) ;
#25190=AXIS2_PLACEMENT_3D ( 'NONE', #8136, #36916, #28213 ) ;
#25202=CARTESIAN_POINT ( 'NONE',  ( 10.56230152254379817, -3.464101615137573198, -7.049999998771014909 ) ) ;
#25205=ORIENTED_EDGE ( 'NONE', *, *, #33134, .T. ) ;
#25209=DIRECTION ( 'NONE',  ( 0.000000000000000000, 0.000000000000000000, 1.000000000000000000 ) ) ;
#25215=CARTESIAN_POINT ( 'NONE',  ( 22.80587116629411426, 7.646167579472024665E-16, -8.071874999385524774 ) ) ;
#25219=( BOUNDED_CURVE ( )  B_SPLINE_CURVE ( 2, ( #27002, #4250, #18300, #27565, #9571, #21885, #21703 ),
 .UNSPECIFIED., .F., .F. ) 
 B_SPLINE_CURVE_WITH_KNOTS ( ( 3, 2, 2, 3 ),
 ( 0.02173913043478281626, 0.02898550724637714154, 0.03623188405797146683, 0.04347826086956579211 ),
 .UNSPECIFIED. ) 
 CURVE ( )  GEOMETRIC_REPRESENTATION_ITEM ( )  RATIONAL_B_SPLINE_CURVE ( ( 0.9999999999999961142, 0.8660254037844425934, 1.000000000000000000, 0.8660254037844387076, 1.000000000000000000, 0.8660254037844280495, 1.000000000000010658 ) ) 
 REPRESENTATION_ITEM ( '' )  );
#25222=CARTESIAN_POINT ( 'NONE',  ( 10.56230152254548926, 3.464101615138548862, -2.624999998770999543 ) ) ;
#25225=CARTESIAN_POINT ( 'NONE',  ( 22.56230152254410370, 7.347880794884117764E-16, -0.5624999987710044280 ) ) ;
#25233=CARTESIAN_POINT ( 'NONE',  ( 16.56230152254411081, 6.928203230275514990, -8.662500000000004974 ) ) ;
#25235=CARTESIAN_POINT ( 'NONE',  ( 13.56230152254411969, -5.196152422706638241, -3.525000000000083844 ) ) ;
#25249=CARTESIAN_POINT ( 'NONE',  ( 22.80587116629412847, -3.604726614523238837, -5.409374999385520688 ) ) ;
#25256=CARTESIAN_POINT ( 'NONE',  ( 19.68408634441911431, 5.407089921784862696, -0.3468749993855158031 ) ) ;
#25273=CARTESIAN_POINT ( 'NONE',  ( 13.56230152254410726, 5.196152422706636465, -1.425000000000037348 ) ) ;
#25279=FACE_OUTER_BOUND ( 'NONE', #21894, .T. ) ;
#25290=CARTESIAN_POINT ( 'NONE',  ( 10.31873187879410914, 0.000000000000000000, -9.590624999385537919 ) ) ;
#25294=ORIENTED_EDGE ( 'NONE', *, *, #20289, .T. ) ;
#25313=AXIS2_PLACEMENT_3D ( 'NONE', #12475, #4446, #36278 ) ;
#25326=CARTESIAN_POINT ( 'NONE',  ( 10.31873187879410914, 0.000000000000000000, -5.990624999385518734 ) ) ;
#25336=CARTESIAN_POINT ( 'NONE',  ( 19.56230152254411792, 5.196152422706637353, -1.950000000000035039 ) ) ;
#25342=CARTESIAN_POINT ( 'NONE',  ( 22.80587116629410716, -3.604726614523235284, -2.203124999385539962 ) ) ;
#25345=CARTESIAN_POINT ( 'NONE',  ( 13.56230152254410548, 5.196152422706630247, -4.012499998771012599 ) ) ;
#25359=CARTESIAN_POINT ( 'NONE',  ( 22.80587116629410716, 7.646167579472015790E-16, -9.815624999385569538 ) ) ;
#25367=CARTESIAN_POINT ( 'NONE',  ( 10.31873187879410381, 0.000000000000000000, -9.646874999385518734 ) ) ;
#25368=CARTESIAN_POINT ( 'NONE',  ( 22.80587116629412847, 3.604726614523243278, -6.234374999385518201 ) ) ;
#25389=ORIENTED_EDGE ( 'NONE', *, *, #4615, .F. ) ;
#25395=CARTESIAN_POINT ( 'NONE',  ( 16.56230152254411436, -6.928203230275514990, -9.787500000000042277 ) ) ;
#25397=CARTESIAN_POINT ( 'NONE',  ( 10.31873187879410203, -3.604726614523244610, -7.809374999385487293 ) ) ;
#25400=CARTESIAN_POINT ( 'NONE',  ( 10.31873187879411269, 3.604726614523236616, -3.778124999385508609 ) ) ;
#25401=EDGE_CURVE ( 'NONE', #1340, #25502, #26436, .T. ) ;
#25407=CARTESIAN_POINT ( 'NONE',  ( 22.56230152254410370, 3.464101615137755275, -0.9749999987710199489 ) ) ;
#25409=FACE_OUTER_BOUND ( 'NONE', #6744, .T. ) ;
#25416=CARTESIAN_POINT ( 'NONE',  ( 22.80587116629410716, 7.646167579472015790E-16, -0.3656249993855553715 ) ) ;
#25417=CARTESIAN_POINT ( 'NONE',  ( 16.56230152254410726, 0.000000000000000000, -10.00000000000000000 ) ) ;
#25422=CARTESIAN_POINT ( 'NONE',  ( 10.56230152254411081, 0.000000000000000000, -2.137499998771025034 ) ) ;
#25427=CARTESIAN_POINT ( 'NONE',  ( 22.56230152254421739, 3.464101615137694878, -6.824999998770996612 ) ) ;
#25434=CARTESIAN_POINT ( 'NONE',  ( 22.80587116629411426, 7.646167579472024665E-16, -6.271874999385529392 ) ) ;
#25438=CARTESIAN_POINT ( 'NONE',  ( 10.31873187879411091, 3.604726614523240613, -0.6843749993854860714 ) ) ;
#25440=AXIS2_PLACEMENT_3D ( 'NONE', #28026, #22170, #27469 ) ;
#25457=CARTESIAN_POINT ( 'NONE',  ( 22.56230152254411436, 3.464101615137759271, -1.987500000000063993 ) ) ;
#25475=CARTESIAN_POINT ( 'NONE',  ( 13.44051670066911619, -5.407089921784859143, -9.965624999385552130 ) ) ;
#25492=( BOUNDED_CURVE ( )  B_SPLINE_CURVE ( 2, ( #31789, #5825, #8862, #23275, #14368, #34819, #10959 ),
 .UNSPECIFIED., .F., .F. ) 
 B_SPLINE_CURVE_WITH_KNOTS ( ( 3, 2, 2, 3 ),
 ( 0.7608695652173934620, 0.7681159420289876971, 0.7753623188405820432, 0.7826086956521763893 ),
 .UNSPECIFIED. ) 
 CURVE ( )  GEOMETRIC_REPRESENTATION_ITEM ( )  RATIONAL_B_SPLINE_CURVE ( ( 0.9999999999999610312, 0.8660254037844776764, 1.000000000000000000, 0.8660254037844387076, 1.000000000000000000, 0.8660254037843935215, 1.000000000000045075 ) ) 
 REPRESENTATION_ITEM ( '' )  );
#25502=VERTEX_POINT ( 'NONE', #33458 ) ;
#25509=CARTESIAN_POINT ( 'NONE',  ( 16.56230152254411081, 7.209453229046475009, -5.653124999385517491 ) ) ;
#25518=CARTESIAN_POINT ( 'NONE',  ( 10.31873187879410914, 0.000000000000000000, -2.446874999385534544 ) ) ;
#25525=CARTESIAN_POINT ( 'NONE',  ( 22.80587116629411071, -3.604726614523235284, -2.653124999385503724 ) ) ;
#25532=AXIS2_PLACEMENT_3D ( 'NONE', #24403, #9990, #4301 ) ;
#25542=CARTESIAN_POINT ( 'NONE',  ( 16.56230152254411081, -7.209453229046475009, -9.028124999385502392 ) ) ;
#25547=AXIS2_PLACEMENT_3D ( 'NONE', #10224, #33351, #18780 ) ;
#25552=CARTESIAN_POINT ( 'NONE',  ( 13.44051670066911441, -5.407089921784865361, -9.571874999385554972 ) ) ;
#25553=CARTESIAN_POINT ( 'NONE',  ( 19.68408634441911786, -5.407089921784861808, -9.046874999385529748 ) ) ;
#25557=( BOUNDED_CURVE ( )  B_SPLINE_CURVE ( 2, ( #19411, #16189, #19043, #25077, #7464, #27740, #24894 ),
 .UNSPECIFIED., .F., .F. ) 
 B_SPLINE_CURVE_WITH_KNOTS ( ( 3, 2, 2, 3 ),
 ( 0.5869565217391301548, 0.5942028985507243899, 0.6014492753623188470, 0.6086956521739131931 ),
 .UNSPECIFIED. ) 
 CURVE ( )  GEOMETRIC_REPRESENTATION_ITEM ( )  RATIONAL_B_SPLINE_CURVE ( ( 1.000000000000006217, 0.8660254037844326014, 1.000000000000000000, 0.8660254037844387076, 1.000000000000000000, 0.8660254037844367092, 1.000000000000001998 ) ) 
 REPRESENTATION_ITEM ( '' )  );
#25567=CARTESIAN_POINT ( 'NONE',  ( 22.56230152254221011, 3.464101615138862389, -9.187500000000003553 ) ) ;
#25573=ORIENTED_EDGE ( 'NONE', *, *, #26449, .F. ) ;
#25581=CARTESIAN_POINT ( 'NONE',  ( 19.68408634441911076, 5.407089921784862696, -7.996874999385533478 ) ) ;
#25584=CARTESIAN_POINT ( 'NONE',  ( 22.80587116629410360, 7.646167579472015790E-16, -2.165624999385551419 ) ) ;
#25587=CARTESIAN_POINT ( 'NONE',  ( 16.56230152254411081, -6.928203230275506996, -1.574999998771003495 ) ) ;
#25590=CARTESIAN_POINT ( 'NONE',  ( 10.56230152254411436, -3.464101615137757051, -4.349999998771036047 ) ) ;
#25600=CARTESIAN_POINT ( 'NONE',  ( 19.68408634441910721, 5.407089921784857367, -1.640624999385525973 ) ) ;
#25603=CARTESIAN_POINT ( 'NONE',  ( 11.28998163430637725, -3.344369132205555317, -9.999999999999998224 ) ) ;
#25605=CARTESIAN_POINT ( 'NONE',  ( 22.56230152254410370, 7.347880794884117764E-16, -2.362499998771028231 ) ) ;
#25609=CARTESIAN_POINT ( 'NONE',  ( 22.56230152254410370, 7.347880794884117764E-16, -8.662499998771028942 ) ) ;
#25616=CARTESIAN_POINT ( 'NONE',  ( 13.44051670066910908, 5.407089921784862696, -9.271874999385531169 ) ) ;
#25619=VERTEX_POINT ( 'NONE', #16779 ) ;
#25620=CARTESIAN_POINT ( 'NONE',  ( 16.56230152254411436, 7.209453229046482114, -1.209374999385475657 ) ) ;
#25640=CARTESIAN_POINT ( 'NONE',  ( 19.56230152254411792, 5.196152422706637353, -3.750000000000031086 ) ) ;
#25659=CARTESIAN_POINT ( 'NONE',  ( 13.44051670066911441, -5.407089921784859143, -8.165624999385528326 ) ) ;
#25696=CARTESIAN_POINT ( 'NONE',  ( 16.56230152254411436, -7.209453229046475009, -7.228124999385518556 ) ) ;
#25698=LINE ( 'NONE', #14695, #18290 ) ;
#25705=DIRECTION ( 'NONE',  ( 0.000000000000000000, 0.000000000000000000, 1.000000000000000000 ) ) ;
#25706=ORIENTED_EDGE ( 'NONE', *, *, #17252, .F. ) ;
#25710=CARTESIAN_POINT ( 'NONE',  ( 10.31873187879411091, -3.604726614523240613, -1.453124999385536187 ) ) ;
#25713=EDGE_CURVE ( 'NONE', #15610, #37311, #20932, .T. ) ;
#25728=CARTESIAN_POINT ( 'NONE',  ( 19.68408634441910365, 5.407089921784857367, -9.290624999385570959 ) ) ;
#25734=ORIENTED_EDGE ( 'NONE', *, *, #15285, .F. ) ;
#25740=CARTESIAN_POINT ( 'NONE',  ( 19.68408634441910721, 5.407089921784862696, -9.796874999385529748 ) ) ;
#25759=VERTEX_POINT ( 'NONE', #2171 ) ;
#25761=CARTESIAN_POINT ( 'NONE',  ( 10.56230152254411081, 0.000000000000000000, -2.137499998771025034 ) ) ;
#25768=CARTESIAN_POINT ( 'NONE',  ( 13.44051670066911797, -5.407089921784859143, -4.115624999385558702 ) ) ;
#25773=CARTESIAN_POINT ( 'NONE',  ( 10.56230152254411436, -3.464101615137757051, -2.999999998771016418 ) ) ;
#25775=( BOUNDED_CURVE ( )  B_SPLINE_CURVE ( 2, ( #22854, #11467, #2561, #14131, #26053, #26419, #81 ),
 .UNSPECIFIED., .F., .F. ) 
 B_SPLINE_CURVE_WITH_KNOTS ( ( 3, 2, 2, 3 ),
 ( 0.3695652173913038241, 0.3768115942028981702, 0.3840579710144924608, 0.3913043478260868069 ),
 .UNSPECIFIED. ) 
 CURVE ( )  GEOMETRIC_REPRESENTATION_ITEM ( )  RATIONAL_B_SPLINE_CURVE ( ( 1.000000000000009104, 0.8660254037844293817, 1.000000000000000000, 0.8660254037844387076, 1.000000000000000000, 0.8660254037844418162, 0.9999999999999968914 ) ) 
 REPRESENTATION_ITEM ( '' )  );
#25777=DIRECTION ( 'NONE',  ( 1.000000000000000000, 0.000000000000000000, 0.000000000000000000 ) ) ;
#25789=AXIS2_PLACEMENT_3D ( 'NONE', #31146, #8397, #28472 ) ;
#25790=CARTESIAN_POINT ( 'NONE',  ( 22.56230152254410370, 7.347880794884117764E-16, -5.962499998771020771 ) ) ;
#25797=ORIENTED_EDGE ( 'NONE', *, *, #1154, .F. ) ;
#25801=CARTESIAN_POINT ( 'NONE',  ( 13.44051670066910731, 5.407089921784862696, -7.921874999385513760 ) ) ;
#25807=CARTESIAN_POINT ( 'NONE',  ( 16.56230152254411792, -7.209453229046482114, -0.5343749993854981506 ) ) ;
#25826=CARTESIAN_POINT ( 'NONE',  ( 19.56230152254412502, -5.196152422706635576, -3.450000000000091660 ) ) ;
#25831=CARTESIAN_POINT ( 'NONE',  ( 13.56230152254411614, -5.196152422706632912, -6.562499998771037291 ) ) ;
#25833=DIRECTION ( 'NONE',  ( 1.000000000000000000, 0.000000000000000000, 0.000000000000000000 ) ) ;
#25845=EDGE_CURVE ( 'NONE', #19865, #11078, #34199, .T. ) ;
#25846=CARTESIAN_POINT ( 'NONE',  ( 16.56230152254412147, -7.209453229046482114, -0.9843749993855260838 ) ) ;
#25872=AXIS2_PLACEMENT_3D ( 'NONE', #19343, #1877, #22919 ) ;
#25873=ORIENTED_EDGE ( 'NONE', *, *, #33185, .T. ) ;
#25881=CARTESIAN_POINT ( 'NONE',  ( 19.68408634441910365, 5.407089921784857367, -9.740624999385548932 ) ) ;
#25889=CARTESIAN_POINT ( 'NONE',  ( 22.56230152254410370, 0.000000000000000000, -10.00000000000000000 ) ) ;
#25895=CARTESIAN_POINT ( 'NONE',  ( 22.80587116629410716, 7.646167579472015790E-16, -4.865624999385531169 ) ) ;
#25921=ADVANCED_FACE ( 'NONE', ( #6327 ), #12194, .F. ) ;
#25923=CARTESIAN_POINT ( 'NONE',  ( 13.56230152254410370, 5.196152422706630247, -10.31249999877101331 ) ) ;
#25928=CARTESIAN_POINT ( 'NONE',  ( 19.68408634441911076, 5.407089921784862696, -7.996874999385533478 ) ) ;
#25931=DIRECTION ( 'NONE',  ( 1.000000000000000000, 0.000000000000000000, -0.000000000000000000 ) ) ;
#25934=CARTESIAN_POINT ( 'NONE',  ( 16.56230152254410726, 0.000000000000000000, -10.00000000000000000 ) ) ;
#25947=EDGE_LOOP ( 'NONE', ( #9028, #23991, #25573, #35678 ) ) ;
#25957=CARTESIAN_POINT ( 'NONE',  ( 22.80587116629410716, 3.604726614523238837, -3.028124999385537031 ) ) ;
#25962=CARTESIAN_POINT ( 'NONE',  ( 10.56230152254411436, -3.464101615137757051, -2.549999998770989151 ) ) ;
#25977=DIRECTION ( 'NONE',  ( 0.000000000000000000, 0.000000000000000000, -1.000000000000000000 ) ) ;
#25981=EDGE_CURVE ( 'NONE', #11631, #11055, #537, .T. ) ;
#25988=CARTESIAN_POINT ( 'NONE',  ( 16.56230152254411436, -7.209453229046482114, -9.534374999385541116 ) ) ;
#25992=CARTESIAN_POINT ( 'NONE',  ( 22.80587116629411781, -3.604726614523238837, -3.609374999385538185 ) ) ;
#26011=CARTESIAN_POINT ( 'NONE',  ( 10.56230152254410903, 3.464101615137757051, -4.087500000000054534 ) ) ;
#26012=ORIENTED_EDGE ( 'NONE', *, *, #21001, .T. ) ;
#26029=CARTESIAN_POINT ( 'NONE',  ( 22.80587116629412492, -3.604726614523238837, -0.4593749993855362757 ) ) ;
#26053=CARTESIAN_POINT ( 'NONE',  ( 13.56230152254411614, -5.196152422706632912, -4.312499998771063048 ) ) ;
#26066=CARTESIAN_POINT ( 'NONE',  ( 22.80587116629410716, 7.646167579472015790E-16, -9.815624999385569538 ) ) ;
#26069=CARTESIAN_POINT ( 'NONE',  ( 13.62844269029146638, 5.304656780843813202, -10.00000000000000000 ) ) ;
#26078=DIRECTION ( 'NONE',  ( 1.000000000000000000, 0.000000000000000000, 0.000000000000000000 ) ) ;
#26079=CARTESIAN_POINT ( 'NONE',  ( 19.68408634441910365, -5.407089921784855591, -5.390624999385557281 ) ) ;
#26085=VERTEX_POINT ( 'NONE', #8728 ) ;
#26093=AXIS2_PLACEMENT_3D ( 'NONE', #14591, #28794, #37142 ) ;
#26105=CARTESIAN_POINT ( 'NONE',  ( 15.52041685288908823, 5.908847293266075162, -10.33697644040032060 ) ) ;
#26109=CARTESIAN_POINT ( 'NONE',  ( 10.31873187879410381, 0.000000000000000000, -9.646874999385518734 ) ) ;
#26123=CARTESIAN_POINT ( 'NONE',  ( 10.56230152254410903, 7.347880794884117764E-16, -10.00000000000000000 ) ) ;
#26137=ADVANCED_FACE ( 'NONE', ( #28991 ), #2293, .F. ) ;
#26139=CARTESIAN_POINT ( 'NONE',  ( 16.56230152254411436, 7.209453229046475009, -2.053124999385520066 ) ) ;
#26140=EDGE_CURVE ( 'NONE', #32302, #34717, #18728, .T. ) ;
#26145=CARTESIAN_POINT ( 'NONE',  ( 10.56230152254411081, 0.000000000000000000, -4.837499998771033205 ) ) ;
#26153=DIRECTION ( 'NONE',  ( 0.000000000000000000, 0.000000000000000000, 1.000000000000000000 ) ) ;
#26172=CARTESIAN_POINT ( 'NONE',  ( 16.56230152254411436, 7.209453229046482114, -7.959374999385476102 ) ) ;
#26176=CARTESIAN_POINT ( 'NONE',  ( 16.56230152254411436, -7.209453229046482114, -2.784374999385508698 ) ) ;
#26193=CARTESIAN_POINT ( 'NONE',  ( 16.56230152254411436, -6.928203230275514990, -4.837499999999994138 ) ) ;
#26198=CARTESIAN_POINT ( 'NONE',  ( 13.56230152254410726, 5.196152422706636465, -6.375000000000019540 ) ) ;
#26211=CARTESIAN_POINT ( 'NONE',  ( 10.31873187879410736, -3.604726614523244610, -1.509374999385515670 ) ) ;
#26216=VERTEX_POINT ( 'NONE', #16898 ) ;
#26217=( BOUNDED_CURVE ( )  B_SPLINE_CURVE ( 2, ( #5713, #11225, #22795, #34346, #8015, #33975, #17108 ),
 .UNSPECIFIED., .F., .F. ) 
 B_SPLINE_CURVE_WITH_KNOTS ( ( 3, 2, 2, 3 ),
 ( 0.000000000000000000, 0.007246376811594271508, 0.01449275362318854302, 0.02173913043478281626 ),
 .UNSPECIFIED. ) 
 CURVE ( )  GEOMETRIC_REPRESENTATION_ITEM ( )  RATIONAL_B_SPLINE_CURVE ( ( 1.000000000000000000, 0.8660254037844387076, 1.000000000000000000, 0.8660254037844387076, 1.000000000000000000, 0.8660254037844348218, 1.000000000000003775 ) ) 
 REPRESENTATION_ITEM ( '' )  );
#26235=DIRECTION ( 'NONE',  ( 0.000000000000000000, 0.000000000000000000, 1.000000000000000000 ) ) ;
#26243=DIRECTION ( 'NONE',  ( 0.000000000000000000, 0.000000000000000000, 1.000000000000000000 ) ) ;
#26244=CARTESIAN_POINT ( 'NONE',  ( 19.68408634441910365, 5.407089921784857367, -9.290624999385570959 ) ) ;
#26257=CARTESIAN_POINT ( 'NONE',  ( 22.80587116629410716, 7.646167579472015790E-16, -5.315624999385537564 ) ) ;
#26261=VECTOR ( 'NONE', #20940, 1000.000000000000000 ) ;
#26267=CARTESIAN_POINT ( 'NONE',  ( 22.56230152254412147, 7.347880794884125653E-16, -3.825000000000050804 ) ) ;
#26271=CARTESIAN_POINT ( 'NONE',  ( 22.56230152254412147, 7.347880794884125653E-16, -4.275000000000028777 ) ) ;
#26286=ORIENTED_EDGE ( 'NONE', *, *, #33781, .F. ) ;
#26291=CARTESIAN_POINT ( 'NONE',  ( 16.56230152254411436, -7.209453229046482114, -9.984374999385536853 ) ) ;
#26292=CARTESIAN_POINT ( 'NONE',  ( 19.68408634441910721, -5.407089921784855591, -2.690624999385549110 ) ) ;
#26302=EDGE_CURVE ( 'NONE', #8245, #26216, #22900, .T. ) ;
#26322=CARTESIAN_POINT ( 'NONE',  ( 16.56230152254411081, -7.209453229046475009, -6.328124999385527083 ) ) ;
#26328=CARTESIAN_POINT ( 'NONE',  ( 22.56230152254410370, 7.347880794884117764E-16, -3.712499998771018106 ) ) ;
#26341=ORIENTED_EDGE ( 'NONE', *, *, #10195, .T. ) ;
#26347=CARTESIAN_POINT ( 'NONE',  ( 22.56230152254411792, 7.347880794884125653E-16, -7.875000000000048850 ) ) ;
#26350=CARTESIAN_POINT ( 'NONE',  ( 10.56230152254410903, 0.000000000000000000, -8.437499998771025744 ) ) ;
#26353=ORIENTED_EDGE ( 'NONE', *, *, #19875, .F. ) ;
#26360=CARTESIAN_POINT ( 'NONE',  ( 13.44051670066911086, 5.407089921784862696, -2.971874999385532234 ) ) ;
#26361=CONICAL_SURFACE ( 'NONE', #932, 5.999999999999998224, 0.2617993877991499074 ) ;
#26378=EDGE_CURVE ( 'NONE', #26550, #36019, #25009, .T. ) ;
#26380=CARTESIAN_POINT ( 'NONE',  ( 13.56230152254411614, -5.196152422706638241, -5.325000000000079226 ) ) ;
#26396=ORIENTED_EDGE ( 'NONE', *, *, #10179, .T. ) ;
#26401=CARTESIAN_POINT ( 'NONE',  ( 13.44051670066911264, -5.407089921784865361, -1.471874999385502925 ) ) ;
#26406=EDGE_LOOP ( 'NONE', ( #5151, #27533, #8003, #12290 ) ) ;
#26419=CARTESIAN_POINT ( 'NONE',  ( 10.56230152254419430, -3.464101615137802348, -4.349999998771035159 ) ) ;
#26430=CYLINDRICAL_SURFACE ( 'NONE', #15143, 5.999999999999998224 ) ;
#26431=CARTESIAN_POINT ( 'NONE',  ( 10.31873187879410736, -3.604726614523240613, -8.203124999385503102 ) ) ;
#26432=CARTESIAN_POINT ( 'NONE',  ( 19.56230152254412502, -5.196152422706635576, -2.550000000000052225 ) ) ;
#26436=( BOUNDED_CURVE ( )  B_SPLINE_CURVE ( 2, ( #24376, #16038, #21726, #27587, #33276, #18888, #35920 ),
 .UNSPECIFIED., .F., .F. ) 
 B_SPLINE_CURVE_WITH_KNOTS ( ( 3, 2, 2, 3 ),
 ( 0.8913043478260829211, 0.8985507246376781554, 0.9057971014492732786, 0.9130434782608684019 ),
 .UNSPECIFIED. ) 
 CURVE ( )  GEOMETRIC_REPRESENTATION_ITEM ( )  RATIONAL_B_SPLINE_CURVE ( ( 1.000000000000073941, 0.8660254037843647668, 1.000000000000000000, 0.8660254037844387076, 1.000000000000000000, 0.8660254037844592467, 0.9999999999999794609 ) ) 
 REPRESENTATION_ITEM ( '' )  );
#26444=CARTESIAN_POINT ( 'NONE',  ( 10.56230152254345001, -3.464101615137374246, -3.449999998771020593 ) ) ;
#26445=CARTESIAN_POINT ( 'NONE',  ( 16.56230152254411436, -7.209453229046475009, -4.978124999385539873 ) ) ;
#26449=EDGE_CURVE ( 'NONE', #13344, #21775, #37285, .T. ) ;
#26461=CYLINDRICAL_SURFACE ( 'NONE', #4631, 5.999999999999998224 ) ;
#26468=CARTESIAN_POINT ( 'NONE',  ( 19.56230152254410370, 5.196152422706631135, -4.537499998771011178 ) ) ;
#26479=CARTESIAN_POINT ( 'NONE',  ( 10.31873187879411091, -3.604726614523240613, -1.453124999385536187 ) ) ;
#26495=EDGE_CURVE ( 'NONE', #24827, #7868, #18531, .T. ) ;
#26510=CARTESIAN_POINT ( 'NONE',  ( 19.68408634441910365, 5.407089921784857367, -4.340624999385561900 ) ) ;
#26516=CARTESIAN_POINT ( 'NONE',  ( 22.56230152254409660, 3.464101615137755275, -7.274999998771023435 ) ) ;
#26523=( BOUNDED_CURVE ( )  B_SPLINE_CURVE ( 2, ( #21989, #33536, #4536, #19152, #15926, #27475, #30881 ),
 .UNSPECIFIED., .F., .F. ) 
 B_SPLINE_CURVE_WITH_KNOTS ( ( 3, 2, 2, 3 ),
 ( 0.4347826086956499969, 0.4420289855072442875, 0.4492753623188385781, 0.4565217391304328132 ),
 .UNSPECIFIED. ) 
 CURVE ( )  GEOMETRIC_REPRESENTATION_ITEM ( )  RATIONAL_B_SPLINE_CURVE ( ( 1.000000000000039968, 0.8660254037843986286, 1.000000000000000000, 0.8660254037844387076, 1.000000000000000000, 0.8660254037844746788, 0.9999999999999640288 ) ) 
 REPRESENTATION_ITEM ( '' )  );
#26524=LINE ( 'NONE', #12509, #5441 ) ;
#26538=CARTESIAN_POINT ( 'NONE',  ( 19.68408634441910721, 5.407089921784857367, -0.7406249993855418268 ) ) ;
#26550=VERTEX_POINT ( 'NONE', #29690 ) ;
#26551=CARTESIAN_POINT ( 'NONE',  ( 13.44051670066911264, -5.407089921784865361, -3.271874999385554261 ) ) ;
#26569=CARTESIAN_POINT ( 'NONE',  ( 16.56230152254411436, 6.928203230275514990, -5.962500000000031442 ) ) ;
#26587=CARTESIAN_POINT ( 'NONE',  ( 22.80587116629412847, 3.604726614523243278, -1.734374999385497551 ) ) ;
#26592=ORIENTED_EDGE ( 'NONE', *, *, #23035, .T. ) ;
#26593=ORIENTED_EDGE ( 'NONE', *, *, #10840, .F. ) ;
#26605=ADVANCED_FACE ( 'NONE', ( #33801 ), #19410, .F. ) ;
#26610=CARTESIAN_POINT ( 'NONE',  ( 16.56230152254412147, 6.928203230275514990, -0.5625000000000507372 ) ) ;
#26613=CARTESIAN_POINT ( 'NONE',  ( 10.56230152254410726, 0.000000000000000000, -9.900000000000048317 ) ) ;
#26620=CARTESIAN_POINT ( 'NONE',  ( 13.44051670066911619, -5.407089921784859143, -9.515624999385547511 ) ) ;
#26631=CARTESIAN_POINT ( 'NONE',  ( 10.56230152254410903, 0.000000000000000000, -3.487499998771015353 ) ) ;
#26632=CARTESIAN_POINT ( 'NONE',  ( 22.80587116629410716, 7.646167579472015790E-16, -4.415624999385525662 ) ) ;
#26638=ORIENTED_EDGE ( 'NONE', *, *, #34155, .T. ) ;
#26644=VECTOR ( 'NONE', #8229, 1000.000000000000000 ) ;
#26647=DIRECTION ( 'NONE',  ( 0.000000000000000000, 0.000000000000000000, 1.000000000000000000 ) ) ;
#26668=CARTESIAN_POINT ( 'NONE',  ( 16.56230152254411436, 7.209453229046475009, -1.603124999385524108 ) ) ;
#26680=PRODUCT_DEFINITION_CONTEXT ( 'detailed design', #9320, 'design' ) ;
#26695=LINE ( 'NONE', #18188, #18596 ) ;
#26697=CARTESIAN_POINT ( 'NONE',  ( 22.80587116629411071, 3.604726614523238837, -6.178124999385540050 ) ) ;
#26701=( BOUNDED_SURFACE ( )  B_SPLINE_SURFACE ( 1, 2, ( 
 ( #31211, #1654, #16635, #36705, #27992, #5240, #21763, #4867, #33682, #33494, #33313, #28177, #7353, #19672, #21949, #10744, #24957, #4498, #2395, #16075, #5052, #36515, #36327, #18926, #30477, #27624, #13228, #7540, #10559, #19112, #24777, #22317, #10374, #7722, #30843, #2207, #13788, #30662, #16447, #33869, #4679, #36884, #2022, #13600, #22136, #7911, #10186, #25150, #16261, #27811, #1839, #19484, #16817, #22505, #34052, #28359, #13408, #31031, #19305, #13969, #25518, #16997, #5416, #37071, #11117, #28537, #8281, #22694, #34238, #19854, #31397, #6627, #18013, #21050, #7016, #32964, #18584, #35426, #30126, #21608, #27468, #30315, #27278, #9287, #1121, #29938, #15539, #29743, #23692, #18203, #32777, #32588, #29557, #12311, #27097, #18776, #10028, #6440, #4158, #23885, #21238, #3776, #9474, #12687, #24443, #24259, #15350, #26904, #35802, #20861, #32400, #7203, #12875, #9845, #3965, #1308, #21423, #15728, #33157, #35992, #4339, #15919, #12118, #933, #35237, #3596, #15160, #26709, #740, #6813, #12506, #9661, #24070, #35616, #18388, #4712, #7383, #5274, #36360, #1494, #19336, #7754, #1683, #36548, #36173, #25185, #22537, #16106, #19706, #33528, #30875, #10409, #10219, #2242, #1870, #30510, #16854, #4530, #21983, #13821, #13069, #25368, #24625, #16292, #7942, #7570, #27657, #19145, #28212, #21793, #31245, #27839, #36738, #13258, #36915, #4898, #33346, #28025, #10963, #10590, #34084, #18955, #19518, #10777, #22169, #24808, #22351, #2058, #30695, #13441, #8135, #24991, #33713, #31064, #16479, #13636, #33900, #5088, #16666, #20253, #23459, #20627, #14745, #17598, #34458, #34636, #31612, #31793, #25928, #23092, #34823, #11705, #11891, #28573, #11154, #6014, #14556, #32169, #35013, #34274, #31986, #8499, #22912, #20067, #5830, #17409, #14372, #14001, #17035, #11340, #23280, #2800, #5639, #8317, #6207, #28391, #25553, #19889, #17223, #28761, #37472, #11522, #9056, #8866, #28950, #2428, #37106, #22727, #20443, #2987, #31431, #5452, #26109, #29130, #142, #2612, #25740, #3171, #14188, #37292, #8682, #26291, #326, #16517, #7427, #15959, #27513, #36215, #30358 ),
 ( #10819, #22390, #27697, #1910, #30916, #1725, #25225, #36590, #25031, #30735, #28064, #33200, #10629, #21833, #24851, #10258, #19374, #25407, #36774, #33940, #13859, #31104, #22208, #33757, #1536, #2282, #2099, #7797, #5125, #36958, #4935, #18996, #33574, #13479, #7982, #4382, #13294, #13108, #4570, #13677, #19555, #16705, #30553, #28253, #11004, #7240, #18815, #24663, #33387, #16147, #36400, #10445, #22021, #7610, #19186, #16330, #4757, #27878, #22761, #25962, #29166, #20478, #16890, #28982, #34310, #31649, #31465, #8354, #19636, #34861, #11557, #25773, #28610, #23131, #31284, #5312, #17634, #23314, #34674, #14406, #11745, #8719, #5487, #11187, #17070, #5865, #34493, #2647, #2467, #14784, #26328, #19747, #14041, #14223, #37325, #11375, #22947, #20291, #6048, #37145, #3210, #8534, #31831, #19927, #28426, #8901, #20100, #25590, #364, #5676, #17257, #32017, #22576, #34122, #8172, #28796, #3023, #2834, #17443, #14593, #26145, #179, #4154, #26704, #9656, #14968, #35799, #3771, #9094, #929, #12684, #9469, #24255, #32209, #18384, #35612, #21044, #23686, #32773, #12499, #23497, #735, #9841, #12113, #29552, #3962, #546, #3591, #17823, #35046, #29360, #15345, #7012, #15725, #21418, #1118, #18008, #18198, #15153, #26899, #32581, #6622, #29934, #6808, #32961, #35232, #6246, #27093, #21234, #27275, #18581, #3399, #15536, #12306, #6434, #23880, #30123, #29737, #35418, #20855, #9282, #32394, #11928, #24066, #20663, #26516, #31060, #5084, #35988, #30312, #18952, #21790, #7381, #30506, #22346, #22165, #27835, #16662, #1303, #36543, #16475, #13436, #19514, #36170, #10586, #12872, #4336, #10024, #27464, #24985, #1865, #24439, #13255, #19141, #7938, #4526, #7199, #21605, #10216, #33154, #30690, #7566, #1491, #36356, #18771, #15915, #24804, #4708, #13065, #16102, #24622, #33342, #27654, #1680, #16288, #33709, #10403, #21978, #33523, #7749, #33896, #19332, #30871, #4894, #28020, #2053, #13631, #25181, #36733, #10773, #31981, #31241, #11149, #28945, #28208, #14552, #6010, #5448, #34632, #37100, #5270, #34269, #17405, #2238, #20438, #17030, #25923, #16849, #26105 ) ),
 .UNSPECIFIED., .F., .F., .F. ) 
 B_SPLINE_SURFACE_WITH_KNOTS ( ( 2, 2 ),
 ( 3, 2, 2, 2, 2, 2, 2, 2, 2, 2, 2, 2, 2, 2, 2, 2, 2, 2, 2, 2, 2, 2, 2, 2, 2, 2, 2, 2, 2, 2, 2, 2, 2, 2, 2, 2, 2, 2, 2, 2, 2, 2, 2, 2, 2, 2, 2, 2, 2, 2, 2, 2, 2, 2, 2, 2, 2, 2, 2, 2, 2, 2, 2, 2, 2, 2, 2, 2, 2, 2, 2, 2, 2, 2, 2, 2, 2, 2, 2, 2, 2, 2, 2, 2, 2, 2, 2, 2, 2, 2, 2, 2, 2, 2, 2, 2, 2, 2, 2, 2, 2, 2, 2, 2, 2, 2, 2, 2, 2, 2, 2, 2, 2, 2, 2, 2, 2, 2, 2, 2, 2, 2, 2, 2, 2, 2, 2, 2, 2, 2, 2, 2, 2, 2, 3 ),
 ( 0.000000000000000000, 1.000000000000000000 ),
 ( 0.000000000000000000, 0.007246376811594202987, 0.01449275362318840597, 0.02173913043478260809, 0.02898550724637681195, 0.03623188405797101580, 0.04347826086956521618, 0.05072463768115942351, 0.05797101449275362389, 0.06521739130434782428, 0.07246376811594203160, 0.07971014492753622505, 0.08695652173913043237, 0.09420289855072463969, 0.1014492753623188470, 0.1086956521739130405, 0.1159420289855072478, 0.1231884057971014551, 0.1304347826086956486, 0.1376811594202898559, 0.1449275362318840632, 0.1521739130434782705, 0.1594202898550724501, 0.1666666666666666574, 0.1739130434782608647, 0.1811594202898550721, 0.1884057971014492794, 0.1956521739130434867, 0.2028985507246376940, 0.2101449275362318736, 0.2173913043478260809, 0.2246376811594202882, 0.2318840579710144956, 0.2391304347826087029, 0.2463768115942029102, 0.2536231884057971175, 0.2608695652173912971, 0.2681159420289855322, 0.2753623188405797118, 0.2826086956521738913, 0.2898550724637681264, 0.2971014492753623060, 0.3043478260869565410, 0.3115942028985507206, 0.3188405797101449002, 0.3260869565217391353, 0.3333333333333333148, 0.3405797101449275499, 0.3478260869565217295, 0.3550724637681159646, 0.3623188405797101441, 0.3695652173913043237, 0.3768115942028985588, 0.3840579710144927383, 0.3913043478260869734, 0.3985507246376811530, 0.4057971014492753881, 0.4130434782608695676, 0.4202898550724637472, 0.4275362318840579823, 0.4347826086956521618, 0.4420289855072463969, 0.4492753623188405765, 0.4565217391304347561, 0.4637681159420289911, 0.4710144927536231707, 0.4782608695652174058, 0.4855072463768115854, 0.4927536231884058204, 0.5000000000000000000, 0.5072463768115942351, 0.5144927536231883591, 0.5217391304347825942, 0.5289855072463768293, 0.5362318840579710644, 0.5434782608695651884, 0.5507246376811594235, 0.5579710144927536586, 0.5652173913043477826, 0.5724637681159420177, 0.5797101449275362528, 0.5869565217391304879, 0.5942028985507246119, 0.6014492753623188470, 0.6086956521739130821, 0.6159420289855072062, 0.6231884057971014412, 0.6304347826086956763, 0.6376811594202898004, 0.6449275362318840354, 0.6521739130434782705, 0.6594202898550725056, 0.6666666666666666297, 0.6739130434782608647, 0.6811594202898550998, 0.6884057971014492239, 0.6956521739130434590, 0.7028985507246376940, 0.7101449275362319291, 0.7173913043478260532, 0.7246376811594202882, 0.7318840579710145233, 0.7391304347826086474, 0.7463768115942028825, 0.7536231884057971175, 0.7608695652173913526, 0.7681159420289854767, 0.7753623188405797118, 0.7826086956521739468, 0.7898550724637680709, 0.7971014492753623060, 0.8043478260869565410, 0.8115942028985507761, 0.8188405797101449002, 0.8260869565217391353, 0.8333333333333333703, 0.8405797101449274944, 0.8478260869565217295, 0.8550724637681159646, 0.8623188405797101996, 0.8695652173913043237, 0.8768115942028985588, 0.8840579710144927938, 0.8913043478260869179, 0.8985507246376811530, 0.9057971014492753881, 0.9130434782608695121, 0.9202898550724637472, 0.9275362318840579823, 0.9347826086956522174, 0.9420289855072463414, 0.9492753623188405765, 0.9565217391304348116, 0.9637681159420289356, 0.9662082944262200268 ),
 .UNSPECIFIED. ) 
 GEOMETRIC_REPRESENTATION_ITEM ( )  RATIONAL_B_SPLINE_SURFACE ( (
 ( 1.000000000000000000, 0.8660254037844387076, 1.000000000000000000, 0.8660254037844387076, 1.000000000000000000, 0.8660254037844387076, 1.000000000000000000, 0.8660254037844387076, 1.000000000000000000, 0.8660254037844387076, 1.000000000000000000, 0.8660254037844387076, 1.000000000000000000, 0.8660254037844387076, 1.000000000000000000, 0.8660254037844387076, 1.000000000000000000, 0.8660254037844387076, 1.000000000000000000, 0.8660254037844387076, 1.000000000000000000, 0.8660254037844387076, 1.000000000000000000, 0.8660254037844387076, 1.000000000000000000, 0.8660254037844387076, 1.000000000000000000, 0.8660254037844387076, 1.000000000000000000, 0.8660254037844387076, 1.000000000000000000, 0.8660254037844387076, 1.000000000000000000, 0.8660254037844387076, 1.000000000000000000, 0.8660254037844387076, 1.000000000000000000, 0.8660254037844387076, 1.000000000000000000, 0.8660254037844387076, 1.000000000000000000, 0.8660254037844387076, 1.000000000000000000, 0.8660254037844387076, 1.000000000000000000, 0.8660254037844387076, 1.000000000000000000, 0.8660254037844387076, 1.000000000000000000, 0.8660254037844387076, 1.000000000000000000, 0.8660254037844387076, 1.000000000000000000, 0.8660254037844387076, 1.000000000000000000, 0.8660254037844387076, 1.000000000000000000, 0.8660254037844387076, 1.000000000000000000, 0.8660254037844387076, 1.000000000000000000, 0.8660254037844387076, 1.000000000000000000, 0.8660254037844387076, 1.000000000000000000, 0.8660254037844387076, 1.000000000000000000, 0.8660254037844387076, 1.000000000000000000, 0.8660254037844387076, 1.000000000000000000, 0.8660254037844387076, 1.000000000000000000, 0.8660254037844387076, 1.000000000000000000, 0.8660254037844387076, 1.000000000000000000, 0.8660254037844387076, 1.000000000000000000, 0.8660254037844387076, 1.000000000000000000, 0.8660254037844387076, 1.000000000000000000, 0.8660254037844387076, 1.000000000000000000, 0.8660254037844387076, 1.000000000000000000, 0.8660254037844387076, 1.000000000000000000, 0.8660254037844387076, 1.000000000000000000, 0.8660254037844387076, 1.000000000000000000, 0.8660254037844387076, 1.000000000000000000, 0.8660254037844387076, 1.000000000000000000, 0.8660254037844387076, 1.000000000000000000, 0.8660254037844387076, 1.000000000000000000, 0.8660254037844387076, 1.000000000000000000, 0.8660254037844387076, 1.000000000000000000, 0.8660254037844387076, 1.000000000000000000, 0.8660254037844387076, 1.000000000000000000, 0.8660254037844387076, 1.000000000000000000, 0.8660254037844387076, 1.000000000000000000, 0.8660254037844387076, 1.000000000000000000, 0.8660254037844387076, 1.000000000000000000, 0.8660254037844387076, 1.000000000000000000, 0.8660254037844387076, 1.000000000000000000, 0.8660254037844387076, 1.000000000000000000, 0.8660254037844387076, 1.000000000000000000, 0.8660254037844387076, 1.000000000000000000, 0.8660254037844387076, 1.000000000000000000, 0.8660254037844387076, 1.000000000000000000, 0.8660254037844387076, 1.000000000000000000, 0.8660254037844387076, 1.000000000000000000, 0.8660254037844387076, 1.000000000000000000, 0.8660254037844387076, 1.000000000000000000, 0.8660254037844387076, 1.000000000000000000, 0.8660254037844387076, 1.000000000000000000, 0.8660254037844387076, 1.000000000000000000, 0.8660254037844387076, 1.000000000000000000, 0.8660254037844387076, 1.000000000000000000, 0.8660254037844387076, 1.000000000000000000, 0.8660254037844387076, 1.000000000000000000, 0.8660254037844387076, 1.000000000000000000, 0.8660254037844387076, 1.000000000000000000, 0.8660254037844387076, 1.000000000000000000, 0.8660254037844387076, 1.000000000000000000, 0.8660254037844387076, 1.000000000000000000, 0.8660254037844387076, 1.000000000000000000, 0.8660254037844387076, 1.000000000000000000, 0.8660254037844387076, 1.000000000000000000, 0.8660254037844387076, 1.000000000000000000, 0.8660254037844387076, 1.000000000000000000, 0.8660254037844387076, 1.000000000000000000, 0.8660254037844387076, 1.000000000000000000, 0.8660254037844387076, 1.000000000000000000, 0.8660254037844387076, 1.000000000000000000, 0.8660254037844387076, 1.000000000000000000, 0.8660254037844387076, 1.000000000000000000, 0.8660254037844387076, 1.000000000000000000, 0.8660254037844387076, 1.000000000000000000, 0.8660254037844387076, 1.000000000000000000, 0.8660254037844387076, 1.000000000000000000, 0.8660254037844387076, 1.000000000000000000, 0.8660254037844387076, 1.000000000000000000, 0.8660254037844387076, 1.000000000000000000, 0.8660254037844387076, 1.000000000000000000, 0.8660254037844387076, 1.000000000000000000, 0.8660254037844387076, 1.000000000000000000, 0.8660254037844387076, 1.000000000000000000, 0.8660254037844387076, 1.000000000000000000, 0.8660254037844387076, 1.000000000000000000, 0.8660254037844387076, 1.000000000000000000, 0.8660254037844387076, 1.000000000000000000, 0.8660254037844387076, 1.000000000000000000, 0.8660254037844387076, 1.000000000000000000, 0.8660254037844387076, 1.000000000000000000, 0.8660254037844387076, 1.000000000000000000, 0.8660254037844387076, 1.000000000000000000, 0.8660254037844387076, 1.000000000000000000, 0.8660254037844387076, 1.000000000000000000, 0.8660254037844387076, 1.000000000000000000, 0.8660254037844387076, 1.000000000000000000, 0.8660254037844387076, 1.000000000000000000, 0.8660254037844387076, 1.000000000000000000, 0.8660254037844387076, 1.000000000000000000, 0.8660254037844387076, 1.000000000000000000, 0.8660254037844387076, 1.000000000000000000, 0.8660254037844387076, 1.000000000000000000, 0.8660254037844387076, 1.000000000000000000, 0.8660254037844387076, 1.000000000000000000, 0.8660254037844387076, 1.000000000000000000, 0.8660254037844387076, 1.000000000000000000, 0.8660254037844387076, 1.000000000000000000, 0.8660254037844387076, 1.000000000000000000, 0.8660254037844387076, 1.000000000000000000, 0.8660254037844387076, 1.000000000000000000, 0.8660254037844387076, 1.000000000000000000, 0.8660254037844387076, 1.000000000000000000, 0.8660254037844387076, 1.000000000000000000, 0.9548847740583508159, 0.9401541683247176540),
 ( 1.000000000000000000, 0.8660254037844387076, 1.000000000000000000, 0.8660254037844387076, 1.000000000000000000, 0.8660254037844387076, 1.000000000000000000, 0.8660254037844387076, 1.000000000000000000, 0.8660254037844387076, 1.000000000000000000, 0.8660254037844387076, 1.000000000000000000, 0.8660254037844387076, 1.000000000000000000, 0.8660254037844387076, 1.000000000000000000, 0.8660254037844387076, 1.000000000000000000, 0.8660254037844387076, 1.000000000000000000, 0.8660254037844387076, 1.000000000000000000, 0.8660254037844387076, 1.000000000000000000, 0.8660254037844387076, 1.000000000000000000, 0.8660254037844387076, 1.000000000000000000, 0.8660254037844387076, 1.000000000000000000, 0.8660254037844387076, 1.000000000000000000, 0.8660254037844387076, 1.000000000000000000, 0.8660254037844387076, 1.000000000000000000, 0.8660254037844387076, 1.000000000000000000, 0.8660254037844387076, 1.000000000000000000, 0.8660254037844387076, 1.000000000000000000, 0.8660254037844387076, 1.000000000000000000, 0.8660254037844387076, 1.000000000000000000, 0.8660254037844387076, 1.000000000000000000, 0.8660254037844387076, 1.000000000000000000, 0.8660254037844387076, 1.000000000000000000, 0.8660254037844387076, 1.000000000000000000, 0.8660254037844387076, 1.000000000000000000, 0.8660254037844387076, 1.000000000000000000, 0.8660254037844387076, 1.000000000000000000, 0.8660254037844387076, 1.000000000000000000, 0.8660254037844387076, 1.000000000000000000, 0.8660254037844387076, 1.000000000000000000, 0.8660254037844387076, 1.000000000000000000, 0.8660254037844387076, 1.000000000000000000, 0.8660254037844387076, 1.000000000000000000, 0.8660254037844387076, 1.000000000000000000, 0.8660254037844387076, 1.000000000000000000, 0.8660254037844387076, 1.000000000000000000, 0.8660254037844387076, 1.000000000000000000, 0.8660254037844387076, 1.000000000000000000, 0.8660254037844387076, 1.000000000000000000, 0.8660254037844387076, 1.000000000000000000, 0.8660254037844387076, 1.000000000000000000, 0.8660254037844387076, 1.000000000000000000, 0.8660254037844387076, 1.000000000000000000, 0.8660254037844387076, 1.000000000000000000, 0.8660254037844387076, 1.000000000000000000, 0.8660254037844387076, 1.000000000000000000, 0.8660254037844387076, 1.000000000000000000, 0.8660254037844387076, 1.000000000000000000, 0.8660254037844387076, 1.000000000000000000, 0.8660254037844387076, 1.000000000000000000, 0.8660254037844387076, 1.000000000000000000, 0.8660254037844387076, 1.000000000000000000, 0.8660254037844387076, 1.000000000000000000, 0.8660254037844387076, 1.000000000000000000, 0.8660254037844387076, 1.000000000000000000, 0.8660254037844387076, 1.000000000000000000, 0.8660254037844387076, 1.000000000000000000, 0.8660254037844387076, 1.000000000000000000, 0.8660254037844387076, 1.000000000000000000, 0.8660254037844387076, 1.000000000000000000, 0.8660254037844387076, 1.000000000000000000, 0.8660254037844387076, 1.000000000000000000, 0.8660254037844387076, 1.000000000000000000, 0.8660254037844387076, 1.000000000000000000, 0.8660254037844387076, 1.000000000000000000, 0.8660254037844387076, 1.000000000000000000, 0.8660254037844387076, 1.000000000000000000, 0.8660254037844387076, 1.000000000000000000, 0.8660254037844387076, 1.000000000000000000, 0.8660254037844387076, 1.000000000000000000, 0.8660254037844387076, 1.000000000000000000, 0.8660254037844387076, 1.000000000000000000, 0.8660254037844387076, 1.000000000000000000, 0.8660254037844387076, 1.000000000000000000, 0.8660254037844387076, 1.000000000000000000, 0.8660254037844387076, 1.000000000000000000, 0.8660254037844387076, 1.000000000000000000, 0.8660254037844387076, 1.000000000000000000, 0.8660254037844387076, 1.000000000000000000, 0.8660254037844387076, 1.000000000000000000, 0.8660254037844387076, 1.000000000000000000, 0.8660254037844387076, 1.000000000000000000, 0.8660254037844387076, 1.000000000000000000, 0.8660254037844387076, 1.000000000000000000, 0.8660254037844387076, 1.000000000000000000, 0.8660254037844387076, 1.000000000000000000, 0.8660254037844387076, 1.000000000000000000, 0.8660254037844387076, 1.000000000000000000, 0.8660254037844387076, 1.000000000000000000, 0.8660254037844387076, 1.000000000000000000, 0.8660254037844387076, 1.000000000000000000, 0.8660254037844387076, 1.000000000000000000, 0.8660254037844387076, 1.000000000000000000, 0.8660254037844387076, 1.000000000000000000, 0.8660254037844387076, 1.000000000000000000, 0.8660254037844387076, 1.000000000000000000, 0.8660254037844387076, 1.000000000000000000, 0.8660254037844387076, 1.000000000000000000, 0.8660254037844387076, 1.000000000000000000, 0.8660254037844387076, 1.000000000000000000, 0.8660254037844387076, 1.000000000000000000, 0.8660254037844387076, 1.000000000000000000, 0.8660254037844387076, 1.000000000000000000, 0.8660254037844387076, 1.000000000000000000, 0.8660254037844387076, 1.000000000000000000, 0.8660254037844387076, 1.000000000000000000, 0.8660254037844387076, 1.000000000000000000, 0.8660254037844387076, 1.000000000000000000, 0.8660254037844387076, 1.000000000000000000, 0.8660254037844387076, 1.000000000000000000, 0.8660254037844387076, 1.000000000000000000, 0.8660254037844387076, 1.000000000000000000, 0.8660254037844387076, 1.000000000000000000, 0.8660254037844387076, 1.000000000000000000, 0.8660254037844387076, 1.000000000000000000, 0.8660254037844387076, 1.000000000000000000, 0.8660254037844387076, 1.000000000000000000, 0.8660254037844387076, 1.000000000000000000, 0.8660254037844387076, 1.000000000000000000, 0.8660254037844387076, 1.000000000000000000, 0.8660254037844387076, 1.000000000000000000, 0.8660254037844387076, 1.000000000000000000, 0.8660254037844387076, 1.000000000000000000, 0.8660254037844387076, 1.000000000000000000, 0.8660254037844387076, 1.000000000000000000, 0.8660254037844387076, 1.000000000000000000, 0.8660254037844387076, 1.000000000000000000, 0.8660254037844387076, 1.000000000000000000, 0.8660254037844387076, 1.000000000000000000, 0.8660254037844387076, 1.000000000000000000, 0.9548847740583508159, 0.9401541683247176540) ) ) 
 REPRESENTATION_ITEM ( '' )  SURFACE ( )  );
#26704=CARTESIAN_POINT ( 'NONE',  ( 16.56230152254411436, 6.928203230275506996, -4.949999998771019705 ) ) ;
#26709=CARTESIAN_POINT ( 'NONE',  ( 22.80587116629411781, -3.604726614523238837, -4.959374999385524951 ) ) ;
#26738=CARTESIAN_POINT ( 'NONE',  ( 19.68408634441912142, -5.407089921784861808, -2.746874999385529037 ) ) ;
#26746=EDGE_CURVE ( 'NONE', #18743, #20463, #19935, .T. ) ;
#26756=VECTOR ( 'NONE', #23844, 1000.000000000000000 ) ;
#26760=CARTESIAN_POINT ( 'NONE',  ( 10.56230152254411259, -3.464101615137761048, -6.262500000000039257 ) ) ;
#26768=CARTESIAN_POINT ( 'NONE',  ( 20.03537803801927808, -5.091549871530747673, -10.00000000000000000 ) ) ;
#26778=CARTESIAN_POINT ( 'NONE',  ( 16.56230152254411436, 7.209453229046482114, -4.359374999385510208 ) ) ;
#26786=CARTESIAN_POINT ( 'NONE',  ( 16.56230152254411792, 6.928203230275514990, -1.012500000000046585 ) ) ;
#26791=CARTESIAN_POINT ( 'NONE',  ( 10.31873187879411091, 0.000000000000000000, -0.1406249993855246405 ) ) ;
#26799=CARTESIAN_POINT ( 'NONE',  ( 10.56230152254438615, 3.464101615137917811, -0.4875000000000282441 ) ) ;
#26822=EDGE_CURVE ( 'NONE', #10334, #2700, #14923, .T. ) ;
#26824=CARTESIAN_POINT ( 'NONE',  ( 19.68408634441910721, -5.407089921784855591, -7.640624999385531524 ) ) ;
#26830=ADVANCED_FACE ( 'NONE', ( #36817 ), #10859, .F. ) ;
#26833=CARTESIAN_POINT ( 'NONE',  ( 10.56230152254410903, 0.000000000000000000, -2.250000000000057732 ) ) ;
#26839=CARTESIAN_POINT ( 'NONE',  ( 16.56230152254411081, -6.928203230275506996, -3.824999998771014376 ) ) ;
#26860=CARTESIAN_POINT ( 'NONE',  ( 16.56230152254411081, -7.209453229046475009, -2.728124999385529215 ) ) ;
#26867=CARTESIAN_POINT ( 'NONE',  ( 10.56230152254410903, 0.000000000000000000, -7.987499998771019349 ) ) ;
#26874=CYLINDRICAL_SURFACE ( 'NONE', #25313, 5.999999999999998224 ) ;
#26893=CARTESIAN_POINT ( 'NONE',  ( 13.44051670066911086, 5.407089921784856479, -4.265624999385542182 ) ) ;
#26899=CARTESIAN_POINT ( 'NONE',  ( 16.56230152254411081, 6.928203230275506996, -6.299999998771006915 ) ) ;
#26904=CARTESIAN_POINT ( 'NONE',  ( 10.31873187879410558, -3.604726614523244610, -4.209374999385490312 ) ) ;
#26905=CARTESIAN_POINT ( 'NONE',  ( 13.56230152254410726, 5.196152422706630247, -3.112499998771029119 ) ) ;
#26921=ORIENTED_EDGE ( 'NONE', *, *, #11433, .T. ) ;
#26922=VERTEX_POINT ( 'NONE', #8952 ) ;
#26929=ORIENTED_EDGE ( 'NONE', *, *, #4742, .T. ) ;
#26930=CARTESIAN_POINT ( 'NONE',  ( 19.68408634441911431, 5.407089921784862696, -5.746874999385531702 ) ) ;
#26947=CARTESIAN_POINT ( 'NONE',  ( 22.56230152254410015, 7.347880794884117764E-16, -7.312499998771010645 ) ) ;
#26949=CARTESIAN_POINT ( 'NONE',  ( 22.56230152254411792, 7.347880794884125653E-16, -6.975000000000036948 ) ) ;
#26953=CARTESIAN_POINT ( 'NONE',  ( 22.56230152254320842, -3.464101615138272638, -5.999999998771010645 ) ) ;
#26957=CARTESIAN_POINT ( 'NONE',  ( 16.56230152254411436, 6.928203230275514990, -5.512500000000034817 ) ) ;
#26962=CARTESIAN_POINT ( 'NONE',  ( 22.56230152254410370, 7.347880794884117764E-16, -4.162499998770996967 ) ) ;
#26963=VERTEX_POINT ( 'NONE', #2693 ) ;
#26967=CARTESIAN_POINT ( 'NONE',  ( 19.68408634441911076, 5.407089921784862696, -3.946874999385563410 ) ) ;
#26981=CARTESIAN_POINT ( 'NONE',  ( 22.80587116629410716, 7.646167579472015790E-16, -0.8156249993855335667 ) ) ;
#26995=CARTESIAN_POINT ( 'NONE',  ( 22.56230152254412857, -3.464101615137755275, -0.2625000000000429212 ) ) ;
#26996=( BOUNDED_CURVE ( )  B_SPLINE_CURVE ( 2, ( #29872, #27401, #1055, #12813, #13009, #10157, #33095 ),
 .UNSPECIFIED., .F., .F. ) 
 B_SPLINE_CURVE_WITH_KNOTS ( ( 3, 2, 2, 3 ),
 ( 0.4347826086956553260, 0.4420289855072487284, 0.4492753623188421308, 0.4565217391304354777 ),
 .UNSPECIFIED. ) 
 CURVE ( )  GEOMETRIC_REPRESENTATION_ITEM ( )  RATIONAL_B_SPLINE_CURVE ( ( 0.9999999999999414912, 0.8660254037844972164, 1.000000000000000000, 0.8660254037844387076, 1.000000000000000000, 0.8660254037844253849, 1.000000000000013323 ) ) 
 REPRESENTATION_ITEM ( '' )  );
#27001=ADVANCED_FACE ( 'NONE', ( #2876 ), #5909, .F. ) ;
#27002=CARTESIAN_POINT ( 'NONE',  ( 22.56230152254410370, 7.347880794884117764E-16, -0.5624999987710044280 ) ) ;
#27016=CARTESIAN_POINT ( 'NONE',  ( 10.31873187879411091, -3.604726614523240613, -5.953124999385525307 ) ) ;
#27031=ADVANCED_FACE ( 'NONE', ( #28842 ), #14635, .F. ) ;
#27053=CARTESIAN_POINT ( 'NONE',  ( 10.31873187879411269, 3.604726614523236616, -3.778124999385508609 ) ) ;
#27057=CARTESIAN_POINT ( 'NONE',  ( 22.80587116629411781, 7.646167579472024665E-16, -9.871874999385521932 ) ) ;
#27078=AXIS2_PLACEMENT_3D ( 'NONE', #9749, #12208, #30021 ) ;
#27086=CARTESIAN_POINT ( 'NONE',  ( 10.31873187879410914, 0.000000000000000000, -7.790624999385542537 ) ) ;
#27093=CARTESIAN_POINT ( 'NONE',  ( 10.56230152254411259, -3.464101615137757051, -6.599999998771014731 ) ) ;
#27097=CARTESIAN_POINT ( 'NONE',  ( 13.44051670066911619, -5.407089921784865361, -3.721874999385532679 ) ) ;
#27113=CARTESIAN_POINT ( 'NONE',  ( 22.80587116629410360, -3.604726614523235284, -0.4031249993855248182 ) ) ;
#27124=CARTESIAN_POINT ( 'NONE',  ( 19.68408634441911431, -5.407089921784861808, -5.896874999385542715 ) ) ;
#27125=ORIENTED_EDGE ( 'NONE', *, *, #21473, .F. ) ;
#27142=CARTESIAN_POINT ( 'NONE',  ( 16.56230152254411436, 6.928203230275514990, -6.862500000000055778 ) ) ;
#27161=CARTESIAN_POINT ( 'NONE',  ( 22.80587116629411781, 3.604726614523243278, -4.434374999385503280 ) ) ;
#27177=CARTESIAN_POINT ( 'NONE',  ( 19.56230152254410370, 5.196152422706631135, -0.9374999987709908833 ) ) ;
#27199=CARTESIAN_POINT ( 'NONE',  ( 10.31873187879410914, 0.000000000000000000, -5.990624999385518734 ) ) ;
#27217=CARTESIAN_POINT ( 'NONE',  ( 22.56230152254410370, 0.000000000000000000, -10.00000000000000000 ) ) ;
#27220=CARTESIAN_POINT ( 'NONE',  ( 10.56230152254410548, 0.000000000000000000, -4.050000000000054001 ) ) ;
#27237=VECTOR ( 'NONE', #24993, 1000.000000000000000 ) ;
#27240=CARTESIAN_POINT ( 'NONE',  ( 19.68408634441910721, -5.407089921784855591, -4.040624999385538985 ) ) ;
#27242=CYLINDRICAL_SURFACE ( 'NONE', #25532, 5.999999999999998224 ) ;
#27247=CARTESIAN_POINT ( 'NONE',  ( 19.56230152254411792, -5.196152422706629359, -7.837499998771035870 ) ) ;
#27253=CARTESIAN_POINT ( 'NONE',  ( 22.56230152254411792, 7.347880794884125653E-16, -6.525000000000058975 ) ) ;
#27270=CARTESIAN_POINT ( 'NONE',  ( 19.68408634441910721, 5.407089921784857367, -7.040624999385541649 ) ) ;
#27275=CARTESIAN_POINT ( 'NONE',  ( 10.56230152254411436, 3.464101615137752166, -6.674999998771008691 ) ) ;
#27278=CARTESIAN_POINT ( 'NONE',  ( 13.44051670066911264, -5.407089921784865361, -3.271874999385554261 ) ) ;
#27291=CARTESIAN_POINT ( 'NONE',  ( 10.56230152254411081, 0.000000000000000000, -5.287499998771011178 ) ) ;
#27296=CARTESIAN_POINT ( 'NONE',  ( 19.68408634441910721, -5.407089921784855591, -3.140624999385555061 ) ) ;
#27309=CARTESIAN_POINT ( 'NONE',  ( 13.44051670066911441, -5.407089921784865361, -7.321874999385524774 ) ) ;
#27331=CARTESIAN_POINT ( 'NONE',  ( 19.56230152254412502, -5.196152422706635576, -7.950000000000068567 ) ) ;
#27340=CARTESIAN_POINT ( 'NONE',  ( 10.56230152254363119, 3.464101615137481716, -5.437500000000037303 ) ) ;
#27341=CARTESIAN_POINT ( 'NONE',  ( 22.56230152254410370, 0.000000000000000000, -10.00000000000000000 ) ) ;
#27347=CARTESIAN_POINT ( 'NONE',  ( 16.56230152254411436, 7.209453229046482114, -4.809374999385505944 ) ) ;
#27369=CARTESIAN_POINT ( 'NONE',  ( 10.56230152254410903, 0.000000000000000000, -0.4500000000000614619 ) ) ;
#27371=ORIENTED_EDGE ( 'NONE', *, *, #26140, .F. ) ;
#27374=LINE ( 'NONE', #36086, #36200 ) ;
#27385=CARTESIAN_POINT ( 'NONE',  ( 16.56230152254411081, 7.209453229046475009, -7.903124999385497063 ) ) ;
#27394=LINE ( 'NONE', #30626, #10451 ) ;
#27400=CARTESIAN_POINT ( 'NONE',  ( 19.56230152254411436, -5.196152422706629359, -3.787499998771037824 ) ) ;
#27401=CARTESIAN_POINT ( 'NONE',  ( 10.56230152254562604, 3.464101615138625689, -4.874999998771045284 ) ) ;
#27409=CARTESIAN_POINT ( 'NONE',  ( 10.56230152254410903, 7.347880794884117764E-16, -10.00000000000000000 ) ) ;
#27413=ORIENTED_EDGE ( 'NONE', *, *, #10539, .T. ) ;
#27421=CARTESIAN_POINT ( 'NONE',  ( 22.80587116629410716, 3.604726614523238837, -3.028124999385537475 ) ) ;
#27440=CARTESIAN_POINT ( 'NONE',  ( 22.56230152254410370, 7.347880794884117764E-16, -4.162499998770996967 ) ) ;
#27454=AXIS2_PLACEMENT_3D ( 'NONE', #35671, #3649, #24128 ) ;
#27458=CARTESIAN_POINT ( 'NONE',  ( 22.80587116629410716, 3.604726614523238837, -8.878124999385546445 ) ) ;
#27464=CARTESIAN_POINT ( 'NONE',  ( 19.56230152254410370, 5.196152422706631135, -8.137499998771001941 ) ) ;
#27468=CARTESIAN_POINT ( 'NONE',  ( 19.68408634441912142, -5.407089921784861808, -3.196874999385534988 ) ) ;
#27469=DIRECTION ( 'NONE',  ( 1.000000000000000000, 0.000000000000000000, 0.000000000000000000 ) ) ;
#27475=CARTESIAN_POINT ( 'NONE',  ( 22.56230152254319421, 3.464101615138294843, -4.687500000000025757 ) ) ;
#27485=CARTESIAN_POINT ( 'NONE',  ( 16.56230152254411436, -7.209453229046475009, -0.9281249993855145153 ) ) ;
#27488=ORIENTED_EDGE ( 'NONE', *, *, #14751, .T. ) ;
#27489=ORIENTED_EDGE ( 'NONE', *, *, #32635, .F. ) ;
#27502=CARTESIAN_POINT ( 'NONE',  ( 13.44051670066911441, -5.407089921784865361, -6.871874999385546801 ) ) ;
#27509=PRESENTATION_STYLE_ASSIGNMENT (( #4378 ) ) ;
#27513=CARTESIAN_POINT ( 'NONE',  ( 13.44051670066910731, 5.407089921784862696, -10.17187499938551554 ) ) ;
#27521=CARTESIAN_POINT ( 'NONE',  ( 22.56230152254412147, 3.464101615137759271, -9.187500000000026645 ) ) ;
#27522=VERTEX_POINT ( 'NONE', #7059 ) ;
#27531=CARTESIAN_POINT ( 'NONE',  ( 10.56230152254410726, 0.000000000000000000, -3.600000000000047606 ) ) ;
#27533=ORIENTED_EDGE ( 'NONE', *, *, #26302, .T. ) ;
#27536=CARTESIAN_POINT ( 'NONE',  ( 19.68408634441911076, 5.407089921784862696, -3.496874999385557459 ) ) ;
#27555=EDGE_CURVE ( 'NONE', #18752, #11631, #10447, .T. ) ;
#27565=CARTESIAN_POINT ( 'NONE',  ( 16.56230152254411081, -6.928203230275506996, -0.6749999987709801585 ) ) ;
#27570=CARTESIAN_POINT ( 'NONE',  ( 10.56230152254410726, 0.000000000000000000, -8.887499998771003717 ) ) ;
#27577=CARTESIAN_POINT ( 'NONE',  ( 16.56230152254411436, 7.209453229046475009, -7.003124999385537564 ) ) ;
#27583=ORIENTED_EDGE ( 'NONE', *, *, #10140, .T. ) ;
#27587=CARTESIAN_POINT ( 'NONE',  ( 16.56230152254411436, -6.928203230275514990, -9.337500000000018119 ) ) ;
#27614=CARTESIAN_POINT ( 'NONE',  ( 13.44051670066911797, -5.407089921784859143, -4.115624999385558702 ) ) ;
#27624=CARTESIAN_POINT ( 'NONE',  ( 10.31873187879410381, 3.604726614523240613, -1.134374999385481697 ) ) ;
#27635=ORIENTED_EDGE ( 'NONE', *, *, #28917, .T. ) ;
#27645=AXIS2_PLACEMENT_3D ( 'NONE', #125, #5813, #495 ) ;
#27648=CARTESIAN_POINT ( 'NONE',  ( 22.80587116629410360, -3.604726614523235284, -8.953124999385538629 ) ) ;
#27654=CARTESIAN_POINT ( 'NONE',  ( 19.56230152254410370, 5.196152422706631135, -9.037499998771014731 ) ) ;
#27657=CARTESIAN_POINT ( 'NONE',  ( 13.44051670066911441, -5.407089921784865361, -6.421874999385540406 ) ) ;
#27677=ORIENTED_EDGE ( 'NONE', *, *, #2165, .F. ) ;
#27682=CARTESIAN_POINT ( 'NONE',  ( 13.56230152254411614, -5.196152422706638241, -9.825000000000056133 ) ) ;
#27683=ADVANCED_FACE ( 'NONE', ( #25409 ), #17073, .F. ) ;
#27685=CARTESIAN_POINT ( 'NONE',  ( 22.80587116629411781, 3.604726614523243278, -6.684374999385513938 ) ) ;
#27686=VERTEX_POINT ( 'NONE', #33942 ) ;
#27697=CARTESIAN_POINT ( 'NONE',  ( 13.56230152254410726, 5.196152422706630247, -0.4124999987710209481 ) ) ;
#27705=CARTESIAN_POINT ( 'NONE',  ( 10.56230152254410548, -3.464101615137761048, -9.412500000000042277 ) ) ;
#27722=CARTESIAN_POINT ( 'NONE',  ( 10.31873187879410736, 3.604726614523240613, -6.084374999385531169 ) ) ;
#27740=CARTESIAN_POINT ( 'NONE',  ( 10.56230152254405752, -3.464101615137729961, -6.262500000000040146 ) ) ;
#27746=CARTESIAN_POINT ( 'NONE',  ( 13.56230152254411614, -5.196152422706638241, -1.275000000000053868 ) ) ;
#27763=CARTESIAN_POINT ( 'NONE',  ( 13.44051670066911264, 5.407089921784856479, -8.315624999385541116 ) ) ;
#27767=ORIENTED_EDGE ( 'NONE', *, *, #4409, .F. ) ;
#27769=ORIENTED_EDGE ( 'NONE', *, *, #33781, .T. ) ;
#27802=CARTESIAN_POINT ( 'NONE',  ( 16.56230152254411436, -7.209453229046475009, -4.528124999385512162 ) ) ;
#27811=CARTESIAN_POINT ( 'NONE',  ( 10.31873187879410736, 3.604726614523240613, -2.034374999385505145 ) ) ;
#27830=CARTESIAN_POINT ( 'NONE',  ( 13.44051670066911441, -5.407089921784859143, -8.615624999385563143 ) ) ;
#27835=CARTESIAN_POINT ( 'NONE',  ( 19.56230152254410370, 5.196152422706631135, -7.687499998771024856 ) ) ;
#27838=CARTESIAN_POINT ( 'NONE',  ( 14.39393254099748276, 5.957544813848101306, -10.18332777273551848 ) ) ;
#27839=CARTESIAN_POINT ( 'NONE',  ( 16.56230152254411436, 7.209453229046482114, -6.609374999385519978 ) ) ;
#27858=ORIENTED_EDGE ( 'NONE', *, *, #32161, .T. ) ;
#27864=CARTESIAN_POINT ( 'NONE',  ( 16.56230152254411792, -6.928203230275514990, -0.3375000000000368816 ) ) ;
#27866=CARTESIAN_POINT ( 'NONE',  ( 16.56230152254411436, -7.209453229046482114, -7.734374999385494220 ) ) ;
#27878=CARTESIAN_POINT ( 'NONE',  ( 16.56230152254411081, -6.928203230275506996, -2.474999998771027165 ) ) ;
#27887=CARTESIAN_POINT ( 'NONE',  ( 10.56230152254410903, 3.464101615137757051, -8.587500000000074962 ) ) ;
#27889=CARTESIAN_POINT ( 'NONE',  ( 10.56230152254443055, -3.464101615137944457, -3.562500000000028422 ) ) ;
#27894=FACE_OUTER_BOUND ( 'NONE', #20491, .T. ) ;
#27903=CARTESIAN_POINT ( 'NONE',  ( 10.31873187879411091, -3.604726614523244610, -6.009374999385537208 ) ) ;
#27909=CARTESIAN_POINT ( 'NONE',  ( 16.56230152254411436, 7.209453229046482114, -0.3093749993854842395 ) ) ;
#27912=CARTESIAN_POINT ( 'NONE',  ( 16.56230152254411081, 6.928203230275506996, -9.449999998771041021 ) ) ;
#27914=CARTESIAN_POINT ( 'NONE',  ( 22.56230152254369514, 3.464101615138004409, -9.637499999999985079 ) ) ;
#27927=CARTESIAN_POINT ( 'NONE',  ( 13.56230152254410903, 5.196152422706636465, -2.775000000000027445 ) ) ;
#27942=CARTESIAN_POINT ( 'NONE',  ( 10.56230152254410903, 0.000000000000000000, -7.200000000000040146 ) ) ;
#27946=CARTESIAN_POINT ( 'NONE',  ( 22.80587116629410360, -3.604726614523235284, -8.953124999385540406 ) ) ;
#27975=( BOUNDED_CURVE ( )  B_SPLINE_CURVE ( 2, ( #24824, #13649, #19352, #16495, #36377, #25202, #22369 ),
 .UNSPECIFIED., .F., .F. ) 
 B_SPLINE_CURVE_WITH_KNOTS ( ( 3, 2, 2, 3 ),
 ( 0.6304347826086958984, 0.6376811594202901334, 0.6449275362318845906, 0.6521739130434789367 ),
 .UNSPECIFIED. ) 
 CURVE ( )  GEOMETRIC_REPRESENTATION_ITEM ( )  RATIONAL_B_SPLINE_CURVE ( ( 0.9999999999999958922, 0.8660254037844428154, 1.000000000000000000, 0.8660254037844387076, 1.000000000000000000, 0.8660254037844263841, 1.000000000000012212 ) ) 
 REPRESENTATION_ITEM ( '' )  );
#27984=CARTESIAN_POINT ( 'NONE',  ( 16.56230152254411436, 7.209453229046475009, -7.003124999385537564 ) ) ;
#27990=CARTESIAN_POINT ( 'NONE',  ( 22.56230152254411792, 7.347880794884125653E-16, -6.975000000000036948 ) ) ;
#27992=CARTESIAN_POINT ( 'NONE',  ( 19.68408634441911431, 5.407089921784862696, -0.3468749993855158031 ) ) ;
#28013=CARTESIAN_POINT ( 'NONE',  ( 13.44051670066911619, -5.407089921784859143, -9.065624999385569538 ) ) ;
#28020=CARTESIAN_POINT ( 'NONE',  ( 19.56230152254410370, 5.196152422706631135, -9.487499998770992704 ) ) ;
#28025=CARTESIAN_POINT ( 'NONE',  ( 16.56230152254411081, -7.209453229046482114, -6.834374999385502747 ) ) ;
#28026=CARTESIAN_POINT ( 'NONE',  ( 16.56230152254410726, 0.000000000000000000, 10.00000000000000000 ) ) ;
#28034=CARTESIAN_POINT ( 'NONE',  ( 13.56230152254411436, -5.196152422706638241, -0.3750000000000419664 ) ) ;
#28054=CARTESIAN_POINT ( 'NONE',  ( 10.31873187879410736, 0.000000000000000000, -8.296874999385501326 ) ) ;
#28058=CARTESIAN_POINT ( 'NONE',  ( 13.44051670066911264, 5.407089921784856479, -1.115624999385556038 ) ) ;
#28064=CARTESIAN_POINT ( 'NONE',  ( 13.56230152254411259, -5.196152422706632912, -0.7124999987710434191 ) ) ;
#28072=CARTESIAN_POINT ( 'NONE',  ( 22.56230152254412147, 7.347880794884125653E-16, -8.775000000000032330 ) ) ;
#28074=CARTESIAN_POINT ( 'NONE',  ( 13.56230152254411614, -5.196152422706638241, -8.025000000000058975 ) ) ;
#28089=CARTESIAN_POINT ( 'NONE',  ( 22.80587116629411426, 7.646167579472024665E-16, -6.721874999385535787 ) ) ;
#28094=CARTESIAN_POINT ( 'NONE',  ( 13.44051670066911086, -5.407089921784865361, -0.5718749993855187785 ) ) ;
#28114=CARTESIAN_POINT ( 'NONE',  ( 16.56230152254411436, -6.928203230275514990, -2.137500000000051692 ) ) ;
#28127=VERTEX_POINT ( 'NONE', #2128 ) ;
#28132=CARTESIAN_POINT ( 'NONE',  ( 10.31873187879410736, -3.604726614523240613, -8.203124999385503102 ) ) ;
#28141=CARTESIAN_POINT ( 'NONE',  ( 10.56230152254514643, -3.464101615138358792, -4.462500000000011013 ) ) ;
#28142=LINE ( 'NONE', #25113, #11147 ) ;
#28157=EDGE_CURVE ( 'NONE', #17042, #23387, #19587, .T. ) ;
#28168=CARTESIAN_POINT ( 'NONE',  ( 13.44051670066911619, -5.407089921784859143, -7.715624999385550353 ) ) ;
#28177=CARTESIAN_POINT ( 'NONE',  ( 10.31873187879411091, -3.604726614523244610, -0.6093749993855241964 ) ) ;
#28182=CARTESIAN_POINT ( 'NONE',  ( 22.80587116629411071, -3.604726614523235284, -1.303124999385484095 ) ) ;
#28208=CARTESIAN_POINT ( 'NONE',  ( 13.56230152254410370, 5.196152422706630247, -9.862499998771006915 ) ) ;
#28209=CARTESIAN_POINT ( 'NONE',  ( 16.56230152254410726, 0.000000000000000000, -10.00000000000000000 ) ) ;
#28212=CARTESIAN_POINT ( 'NONE',  ( 10.31873187879410558, 0.000000000000000000, -6.496874999385504168 ) ) ;
#28213=DIRECTION ( 'NONE',  ( 1.000000000000000000, 0.000000000000000000, 0.000000000000000000 ) ) ;
#28243=CARTESIAN_POINT ( 'NONE',  ( 10.31873187879410736, 3.604726614523240613, -7.884374999385513227 ) ) ;
#28246=CARTESIAN_POINT ( 'NONE',  ( 19.68408634441910365, 5.407089921784857367, -3.440624999385522020 ) ) ;
#28253=CARTESIAN_POINT ( 'NONE',  ( 22.56230152254410370, -3.464101615137751278, -1.949999998771005272 ) ) ;
#28256=( LENGTH_UNIT ( ) NAMED_UNIT ( * ) SI_UNIT ( .MILLI., .METRE. ) );
#28260=CARTESIAN_POINT ( 'NONE',  ( 16.56230152254411436, 7.209453229046475009, -0.2531249993855048674 ) ) ;
#28275=CARTESIAN_POINT ( 'NONE',  ( 19.68408634441911431, -5.407089921784861808, -5.446874999385537208 ) ) ;
#28278=EDGE_LOOP ( 'NONE', ( #34567, #32597, #13750, #23531 ) ) ;
#28279=CARTESIAN_POINT ( 'NONE',  ( 22.80587116629411071, -3.604726614523238837, -1.359374999385495775 ) ) ;
#28298=CARTESIAN_POINT ( 'NONE',  ( 19.56230152254412502, -5.196152422706635576, -1.200000000000062128 ) ) ;
#28299=CARTESIAN_POINT ( 'NONE',  ( 10.56230152254410903, 0.000000000000000000, -5.551115123125782702E-14 ) ) ;
#28310=VECTOR ( 'NONE', #36606, 1000.000000000000227 ) ;
#28315=CARTESIAN_POINT ( 'NONE',  ( 22.80587116629411071, -3.604726614523235284, -8.503124999385544669 ) ) ;
#28343=ORIENTED_EDGE ( 'NONE', *, *, #13033, .F. ) ;
#28349=CARTESIAN_POINT ( 'NONE',  ( 10.31873187879410914, 0.000000000000000000, -7.790624999385542537 ) ) ;
#28351=CARTESIAN_POINT ( 'NONE',  ( 22.56230152254411792, 7.347880794884125653E-16, -7.425000000000042455 ) ) ;
#28353=EDGE_CURVE ( 'NONE', #28711, #17872, #26695, .T. ) ;
#28359=CARTESIAN_POINT ( 'NONE',  ( 22.80587116629412847, -3.604726614523238837, -2.259374999385487026 ) ) ;
#28365=CARTESIAN_POINT ( 'NONE',  ( 13.44051670066911619, -5.407089921784859143, -0.9656249993855170466 ) ) ;
#28368=CARTESIAN_POINT ( 'NONE',  ( 10.56230152254410903, 7.347880794884117764E-16, -10.00000000000000000 ) ) ;
#28382=CARTESIAN_POINT ( 'NONE',  ( 16.56230152254411081, -7.209453229046475009, -9.478124999385530103 ) ) ;
#28390=CARTESIAN_POINT ( 'NONE',  ( 13.44051670066911264, -5.407089921784865361, -10.02187499938553294 ) ) ;
#28391=CARTESIAN_POINT ( 'NONE',  ( 22.80587116629412847, -3.604726614523238837, -9.009374999385519445 ) ) ;
#28397=CARTESIAN_POINT ( 'NONE',  ( 10.56230152254477339, 3.464101615138135415, -3.524999998771014109 ) ) ;
#28398=VERTEX_POINT ( 'NONE', #18574 ) ;
#28404=CARTESIAN_POINT ( 'NONE',  ( 19.56230152254411792, 5.196152422706637353, -9.150000000000046541 ) ) ;
#28410=EDGE_LOOP ( 'NONE', ( #30644, #13641, #37218, #15394 ) ) ;
#28415=CARTESIAN_POINT ( 'NONE',  ( 10.56230152254437726, -3.464101615137914703, -9.862500000000036238 ) ) ;
#28417=CARTESIAN_POINT ( 'NONE',  ( 10.31873187879410736, -3.604726614523244610, -8.709374999385509852 ) ) ;
#28420=CARTESIAN_POINT ( 'NONE',  ( 16.56230152254411081, -7.209453229046475009, -1.828124999385505989 ) ) ;
#28423=CARTESIAN_POINT ( 'NONE',  ( 16.56230152254411081, 6.928203230275506996, -2.699999998771041021 ) ) ;
#28426=CARTESIAN_POINT ( 'NONE',  ( 19.56230152254411436, -5.196152422706629359, -4.237499998771044218 ) ) ;
#28428=( BOUNDED_CURVE ( )  B_SPLINE_CURVE ( 2, ( #19895, #28397, #5459, #31437, #2435, #37298, #14008 ),
 .UNSPECIFIED., .F., .F. ) 
 B_SPLINE_CURVE_WITH_KNOTS ( ( 3, 2, 2, 3 ),
 ( 0.3043478260869579288, 0.3115942028985521639, 0.3188405797101463990, 0.3260869565217406896 ),
 .UNSPECIFIED. ) 
 CURVE ( )  GEOMETRIC_REPRESENTATION_ITEM ( )  RATIONAL_B_SPLINE_CURVE ( ( 0.9999999999999743538, 0.8660254037844643538, 1.000000000000000000, 0.8660254037844387076, 1.000000000000000000, 0.8660254037844099528, 1.000000000000028644 ) ) 
 REPRESENTATION_ITEM ( '' )  );
#28434=CARTESIAN_POINT ( 'NONE',  ( 10.56230152254410726, 0.000000000000000000, -6.300000000000055778 ) ) ;
#28436=CARTESIAN_POINT ( 'NONE',  ( 10.31873187879410736, 3.604726614523236616, -1.978124999385525662 ) ) ;
#28442=FACE_OUTER_BOUND ( 'NONE', #17428, .T. ) ;
#28456=CARTESIAN_POINT ( 'NONE',  ( 19.68408634441911076, 5.407089921784862696, -8.446874999385538985 ) ) ;
#28461=CARTESIAN_POINT ( 'NONE',  ( 13.44051670066911441, -5.407089921784865361, -1.021874999385524729 ) ) ;
#28467=CARTESIAN_POINT ( 'NONE',  ( 22.56230152254462240, 3.464101615137467949, -2.887500000000029932 ) ) ;
#28472=DIRECTION ( 'NONE',  ( 1.000000000000000000, 0.000000000000000000, 0.000000000000000000 ) ) ;
#28479=CARTESIAN_POINT ( 'NONE',  ( 22.56230152254411792, 7.347880794884125653E-16, -5.625000000000018652 ) ) ;
#28484=CARTESIAN_POINT ( 'NONE',  ( 10.56230152254410726, 0.000000000000000000, -6.300000000000055778 ) ) ;
#28491=AXIS2_PLACEMENT_3D ( 'NONE', #28980, #19924, #11555 ) ;
#28497=CARTESIAN_POINT ( 'NONE',  ( 10.31873187879410914, 0.000000000000000000, -0.1968749993855323233 ) ) ;
#28522=ORIENTED_EDGE ( 'NONE', *, *, #17122, .F. ) ;
#28526=CARTESIAN_POINT ( 'NONE',  ( 10.56230152254482846, -3.464101615138174051, -0.8625000000000174749 ) ) ;
#28529=CARTESIAN_POINT ( 'NONE',  ( 19.68408634441910721, 5.407089921784857367, -6.590624999385563676 ) ) ;
#28537=CARTESIAN_POINT ( 'NONE',  ( 22.80587116629411426, 3.604726614523243278, -2.634374999385520777 ) ) ;
#28544=CARTESIAN_POINT ( 'NONE',  ( 22.80587116629410360, -3.604726614523235284, -1.753124999385512028 ) ) ;
#28561=CARTESIAN_POINT ( 'NONE',  ( 13.44051670066911086, 5.407089921784856479, -9.215624999385523708 ) ) ;
#28573=CARTESIAN_POINT ( 'NONE',  ( 16.56230152254411081, -7.209453229046482114, -8.184374999385489957 ) ) ;
#28596=CARTESIAN_POINT ( 'NONE',  ( 22.56230152254317645, -3.464101615138286849, -1.949999998771017262 ) ) ;
#28604=CARTESIAN_POINT ( 'NONE',  ( 13.44051670066911797, -5.407089921784859143, -3.665624999385552751 ) ) ;
#28610=CARTESIAN_POINT ( 'NONE',  ( 10.56230152254411081, 0.000000000000000000, -3.037499998771009402 ) ) ;
#28612=CARTESIAN_POINT ( 'NONE',  ( 16.56230152254410726, 0.000000000000000000, -10.00000000000000000 ) ) ;
#28620=CARTESIAN_POINT ( 'NONE',  ( 10.31873187879411091, 3.604726614523236616, -2.428124999385521399 ) ) ;
#28622=VERTEX_POINT ( 'NONE', #22158 ) ;
#28631=CARTESIAN_POINT ( 'NONE',  ( 10.56230152254410726, 0.000000000000000000, -8.887499998771003717 ) ) ;
#28639=CARTESIAN_POINT ( 'NONE',  ( 10.31873187879410736, 3.604726614523240613, -7.884374999385513227 ) ) ;
#28644=CARTESIAN_POINT ( 'NONE',  ( 19.68408634441911431, -5.407089921784861808, -0.9468749993855329894 ) ) ;
#28648=CIRCLE ( 'NONE', #6890, 1.500000000000001332 ) ;
#28662=CARTESIAN_POINT ( 'NONE',  ( 16.56230152254411436, -6.928203230275514990, -4.387500000000030376 ) ) ;
#28663=ORIENTED_EDGE ( 'NONE', *, *, #28157, .F. ) ;
#28679=CARTESIAN_POINT ( 'NONE',  ( 19.68408634441911431, 5.407089921784862696, -0.3468749993855158031 ) ) ;
#28691=( BOUNDED_CURVE ( )  B_SPLINE_CURVE ( 2, ( #30984, #1972, #31168, #8046, #10324, #36277, #27942 ),
 .UNSPECIFIED., .F., .F. ) 
 B_SPLINE_CURVE_WITH_KNOTS ( ( 3, 2, 2, 3 ),
 ( 0.6739130434782591994, 0.6811594202898535455, 0.6884057971014477806, 0.6956521739130421267 ),
 .UNSPECIFIED. ) 
 CURVE ( )  GEOMETRIC_REPRESENTATION_ITEM ( )  RATIONAL_B_SPLINE_CURVE ( ( 1.000000000000030864, 0.8660254037844079544, 1.000000000000000000, 0.8660254037844387076, 1.000000000000000000, 0.8660254037844633546, 0.9999999999999753530 ) ) 
 REPRESENTATION_ITEM ( '' )  );
#28705=ADVANCED_FACE ( 'NONE', ( #32151 ), #26461, .F. ) ;
#28711=VERTEX_POINT ( 'NONE', #23076 ) ;
#28715=CARTESIAN_POINT ( 'NONE',  ( 16.56230152254411081, 6.928203230275506996, -9.899999998771034981 ) ) ;
#28718=CARTESIAN_POINT ( 'NONE',  ( 13.44051670066911264, 5.407089921784856479, -6.065624999385538452 ) ) ;
#28730=CARTESIAN_POINT ( 'NONE',  ( 13.44051670066911264, 5.407089921784856479, -3.815624999385564209 ) ) ;
#28744=FACE_OUTER_BOUND ( 'NONE', #2218, .T. ) ;
#28754=EDGE_LOOP ( 'NONE', ( #4086, #25797, #15928, #11102, #2168, #24089, #15300, #27767, #22300, #24911, #27125, #395, #13470, #792, #8772, #23299, #33822, #35634, #22413, #18784, #20505, #2856, #1900, #34093, #16776, #30995, #23253, #30325, #33871, #34536, #2522, #24363, #21120, #19497, #3616, #10200, #32380, #24882, #17520, #14578, #17854, #15233, #22709, #15447, #6743, #22209, #29042, #25873 ) ) ;
#28758=CARTESIAN_POINT ( 'NONE',  ( 10.56230152254410903, 0.000000000000000000, -6.187499998771023080 ) ) ;
#28761=CARTESIAN_POINT ( 'NONE',  ( 10.31873187879410558, -3.604726614523244610, -9.159374999385507365 ) ) ;
#28764=CARTESIAN_POINT ( 'NONE',  ( 22.56230152254244814, -3.464101615138709178, -1.049999998771002474 ) ) ;
#28767=CARTESIAN_POINT ( 'NONE',  ( 10.31873187879411091, 0.000000000000000000, -0.1406249993855246405 ) ) ;
#28777=ADVANCED_FACE ( 'NONE', ( #6191 ), #14358, .F. ) ;
#28791=CARTESIAN_POINT ( 'NONE',  ( 16.56230152254410726, -7.209453229046475009, -3.178124999385525395 ) ) ;
#28794=DIRECTION ( 'NONE',  ( 0.000000000000000000, 0.000000000000000000, 1.000000000000000000 ) ) ;
#28796=CARTESIAN_POINT ( 'NONE',  ( 22.56230152254411081, -3.464101615137751278, -4.649999998770979914 ) ) ;
#28797=ADVANCED_FACE ( 'NONE', ( #28744 ), #31417, .F. ) ;
#28804=CARTESIAN_POINT ( 'NONE',  ( 19.56230152254411792, 5.196152422706637353, -8.250000000000062172 ) ) ;
#28808=VERTEX_POINT ( 'NONE', #17580 ) ;
#28812=AXIS2_PLACEMENT_3D ( 'NONE', #35936, #32533, #9609 ) ;
#28818=CARTESIAN_POINT ( 'NONE',  ( 16.56230152254410726, -6.928203230275506996, -5.624999998770996434 ) ) ;
#28825=CARTESIAN_POINT ( 'NONE',  ( 22.80587116629412492, 3.604726614523243278, -8.484374999385497773 ) ) ;
#28830=CARTESIAN_POINT ( 'NONE',  ( 22.80587116629411426, 7.646167579472024665E-16, -2.671874999385509319 ) ) ;
#28835=AXIS2_PLACEMENT_3D ( 'NONE', #28612, #14226, #25777 ) ;
#28841=VERTEX_POINT ( 'NONE', #8666 ) ;
#28842=FACE_OUTER_BOUND ( 'NONE', #319, .T. ) ;
#28843=CARTESIAN_POINT ( 'NONE',  ( 10.56230152254410726, 0.000000000000000000, -1.350000000000045608 ) ) ;
#28849=CARTESIAN_POINT ( 'NONE',  ( 10.56230152254410903, 0.000000000000000000, -4.950000000000037481 ) ) ;
#28869=CARTESIAN_POINT ( 'NONE',  ( 13.44051670066911264, -5.407089921784865361, -2.371874999385514826 ) ) ;
#28877=VERTEX_POINT ( 'NONE', #31778 ) ;
#28893=DIRECTION ( 'NONE',  ( 0.000000000000000000, 0.000000000000000000, 1.000000000000000000 ) ) ;
#28904=CARTESIAN_POINT ( 'NONE',  ( 10.31873187879410914, 0.000000000000000000, -8.690624999385526905 ) ) ;
#28907=CARTESIAN_POINT ( 'NONE',  ( 15.52041717089296213, 5.908847349338256727, -9.999738233010948107 ) ) ;
#28917=EDGE_CURVE ( 'NONE', #32942, #10334, #34807, .T. ) ;
#28919=CARTESIAN_POINT ( 'NONE',  ( 22.80587116629410360, 3.604726614523238837, -4.828124999385519978 ) ) ;
#28929=AXIS2_PLACEMENT_3D ( 'NONE', #29076, #26235, #9001 ) ;
#28945=CARTESIAN_POINT ( 'NONE',  ( 10.56230152254411259, 3.464101615137752166, -9.824999998771010823 ) ) ;
#28947=AXIS2_PLACEMENT_3D ( 'NONE', #21696, #20956, #21516 ) ;
#28950=CARTESIAN_POINT ( 'NONE',  ( 19.68408634441910721, 5.407089921784862696, -9.346874999385523353 ) ) ;
#28955=CARTESIAN_POINT ( 'NONE',  ( 18.06230152254410726, 1.836970198721029441E-16, 10.00000000000000000 ) ) ;
#28976=CARTESIAN_POINT ( 'NONE',  ( 13.44051670066911264, -5.407089921784859143, -3.215624999385519267 ) ) ;
#28980=CARTESIAN_POINT ( 'NONE',  ( 16.56230152254410726, 0.000000000000000000, 0.000000000000000000 ) ) ;
#28982=CARTESIAN_POINT ( 'NONE',  ( 16.56230152254411081, 6.928203230275506996, -2.699999998771040577 ) ) ;
#28989=CARTESIAN_POINT ( 'NONE',  ( 16.56230152254410726, 0.000000000000000000, -10.00000000000000000 ) ) ;
#28991=FACE_OUTER_BOUND ( 'NONE', #28410, .T. ) ;
#29007=CARTESIAN_POINT ( 'NONE',  ( 13.44051670066911264, -5.407089921784865361, -7.771874999385531169 ) ) ;
#29011=CARTESIAN_POINT ( 'NONE',  ( 22.80587116629412137, 7.646167579472024665E-16, -3.121874999385543248 ) ) ;
#29029=CARTESIAN_POINT ( 'NONE',  ( 13.56230152254411792, -5.196152422706638241, -4.425000000000068212 ) ) ;
#29042=ORIENTED_EDGE ( 'NONE', *, *, #18881, .T. ) ;
#29048=CARTESIAN_POINT ( 'NONE',  ( 22.80587116629411781, 3.604726614523243278, -0.3843749993855423153 ) ) ;
#29049=CARTESIAN_POINT ( 'NONE',  ( 10.56230152254410726, 0.000000000000000000, -1.350000000000045608 ) ) ;
#29075=ORIENTED_EDGE ( 'NONE', *, *, #17007, .T. ) ;
#29076=CARTESIAN_POINT ( 'NONE',  ( 16.56230152254410726, 0.000000000000000000, 0.000000000000000000 ) ) ;
#29079=CARTESIAN_POINT ( 'NONE',  ( 10.56230152254410903, 0.000000000000000000, -9.787499998771043153 ) ) ;
#29085=CARTESIAN_POINT ( 'NONE',  ( 10.31873187879410914, 0.000000000000000000, -8.240624999385548932 ) ) ;
#29086=CARTESIAN_POINT ( 'NONE',  ( 19.56230152254411792, 5.196152422706637353, -8.700000000000041922 ) ) ;
#29098=CARTESIAN_POINT ( 'NONE',  ( 10.31873187879411269, -3.604726614523240613, -4.603124999385506122 ) ) ;
#29103=ORIENTED_EDGE ( 'NONE', *, *, #34155, .F. ) ;
#29113=CARTESIAN_POINT ( 'NONE',  ( 22.56230152254410370, 0.000000000000000000, -10.00000000000000000 ) ) ;
#29123=ORIENTED_EDGE ( 'NONE', *, *, #15018, .F. ) ;
#29130=CARTESIAN_POINT ( 'NONE',  ( 10.31873187879411091, 3.604726614523240613, -9.684374999385527261 ) ) ;
#29150=ORIENTED_EDGE ( 'NONE', *, *, #32161, .F. ) ;
#29159=CARTESIAN_POINT ( 'NONE',  ( 19.68408634441910365, -5.407089921784855591, -6.290624999385540761 ) ) ;
#29166=CARTESIAN_POINT ( 'NONE',  ( 10.56230152254411081, 0.000000000000000000, -2.587499998771031429 ) ) ;
#29177=DIRECTION ( 'NONE',  ( 0.000000000000000000, 0.000000000000000000, 1.000000000000000000 ) ) ;
#29181=VERTEX_POINT ( 'NONE', #27220 ) ;
#29192=VERTEX_POINT ( 'NONE', #34531 ) ;
#29196=CARTESIAN_POINT ( 'NONE',  ( 19.68408634441912142, -5.407089921784861808, -8.146874999385516958 ) ) ;
#29202=CARTESIAN_POINT ( 'NONE',  ( 13.44051670066911086, -5.407089921784865361, -2.821874999385520777 ) ) ;
#29203=ORIENTED_EDGE ( 'NONE', *, *, #33700, .T. ) ;
#29220=CARTESIAN_POINT ( 'NONE',  ( 10.56230152254411436, -3.464101615137761048, -3.562500000000032863 ) ) ;
#29221=ORIENTED_EDGE ( 'NONE', *, *, #29782, .F. ) ;
#29239=CARTESIAN_POINT ( 'NONE',  ( 22.80587116629411426, 3.604726614523243278, -2.634374999385520777 ) ) ;
#29257=VECTOR ( 'NONE', #13362, 1000.000000000000000 ) ;
#29273=CARTESIAN_POINT ( 'NONE',  ( 19.68408634441910721, -5.407089921784855591, -8.540624999385542537 ) ) ;
#29287=CARTESIAN_POINT ( 'NONE',  ( 19.68408634441911076, 5.407089921784857367, -4.790624999385539873 ) ) ;
#29311=CARTESIAN_POINT ( 'NONE',  ( 13.56230152254410548, 5.196152422706630247, -4.462499998771018994 ) ) ;
#29324=CARTESIAN_POINT ( 'NONE',  ( 10.31873187879410914, 0.000000000000000000, -1.040624999385536542 ) ) ;
#29330=FACE_OUTER_BOUND ( 'NONE', #6941, .T. ) ;
#29354=CARTESIAN_POINT ( 'NONE',  ( 16.56230152254411081, 7.209453229046475009, -6.553124999385508964 ) ) ;
#29357=( BOUNDED_CURVE ( )  B_SPLINE_CURVE ( 2, ( #26613, #457, #31930, #17724, #6343 ),
 .UNSPECIFIED., .F., .F. ) 
 B_SPLINE_CURVE_WITH_KNOTS ( ( 3, 2, 3 ),
 ( 0.9565217391304342565, 0.9637681159420288246, 0.9662082966761268432 ),
 .UNSPECIFIED. ) 
 CURVE ( )  GEOMETRIC_REPRESENTATION_ITEM ( )  RATIONAL_B_SPLINE_CURVE ( ( 1.000000000000010214, 0.8660254037844284936, 1.000000000000000000, 0.9548847324609615050, 0.9401541411607547971 ) ) 
 REPRESENTATION_ITEM ( '' )  );
#29360=CARTESIAN_POINT ( 'NONE',  ( 22.56230152254410370, 7.347880794884117764E-16, -5.962499998771020771 ) ) ;
#29389=EDGE_CURVE ( 'NONE', #12997, #29586, #26217, .T. ) ;
#29395=CARTESIAN_POINT ( 'NONE',  ( 22.80587116629412137, 7.646167579472024665E-16, -4.021874999385527616 ) ) ;
#29416=CARTESIAN_POINT ( 'NONE',  ( 10.56230152254410903, 3.464101615137757051, -8.137500000000047251 ) ) ;
#29417=VERTEX_POINT ( 'NONE', #7323 ) ;
#29426=( BOUNDED_CURVE ( )  B_SPLINE_CURVE ( 2, ( #13847, #19543, #31091, #25395, #27682, #28415, #36945 ),
 .UNSPECIFIED., .F., .F. ) 
 B_SPLINE_CURVE_WITH_KNOTS ( ( 3, 2, 2, 3 ),
 ( 0.9347826086956513292, 0.9420289855072455643, 0.9492753623188399104, 0.9565217391304342565 ),
 .UNSPECIFIED. ) 
 CURVE ( )  GEOMETRIC_REPRESENTATION_ITEM ( )  RATIONAL_B_SPLINE_CURVE ( ( 1.000000000000016431, 0.8660254037844222763, 1.000000000000000000, 0.8660254037844387076, 1.000000000000000000, 0.8660254037844489217, 0.9999999999999897859 ) ) 
 REPRESENTATION_ITEM ( '' )  );
#29434=CARTESIAN_POINT ( 'NONE',  ( 19.68408634441912142, -5.407089921784861808, -1.846874999385544891 ) ) ;
#29454=CARTESIAN_POINT ( 'NONE',  ( 10.56230152254347487, 3.464101615137389345, -7.237500000000049560 ) ) ;
#29466=CARTESIAN_POINT ( 'NONE',  ( 22.80587116629411426, -3.604726614523235284, -8.053124999385516958 ) ) ;
#29478=CARTESIAN_POINT ( 'NONE',  ( 22.80587116629410716, 3.604726614523238837, -5.278124999385515714 ) ) ;
#29514=CARTESIAN_POINT ( 'NONE',  ( 22.80587116629410360, -3.604726614523235284, -1.753124999385512028 ) ) ;
#29520=CARTESIAN_POINT ( 'NONE',  ( 10.56230152254336474, 3.464101615137328505, -4.987500000000038014 ) ) ;
#29546=CARTESIAN_POINT ( 'NONE',  ( 13.44051670066911619, -5.407089921784859143, -5.465624999385548577 ) ) ;
#29552=CARTESIAN_POINT ( 'NONE',  ( 10.56230152254410903, 0.000000000000000000, -5.737499998771017573 ) ) ;
#29557=CARTESIAN_POINT ( 'NONE',  ( 19.68408634441912142, -5.407089921784861808, -3.646874999385540939 ) ) ;
#29561=CARTESIAN_POINT ( 'NONE',  ( 10.56230152254410903, 0.000000000000000000, -5.551115123125782702E-14 ) ) ;
#29570=CARTESIAN_POINT ( 'NONE',  ( 22.56230152254376975, -3.464101615137950230, -5.099999998771011178 ) ) ;
#29574=CARTESIAN_POINT ( 'NONE',  ( 22.80587116629410716, 7.646167579472015790E-16, -0.3656249993855553715 ) ) ;
#29585=CARTESIAN_POINT ( 'NONE',  ( 10.31873187879410558, 0.000000000000000000, -4.246874999385502392 ) ) ;
#29586=VERTEX_POINT ( 'NONE', #18578 ) ;
#29605=CARTESIAN_POINT ( 'NONE',  ( 13.56230152254410726, 5.196152422706636465, -5.925000000000041567 ) ) ;
#29614=CARTESIAN_POINT ( 'NONE',  ( 10.56230152254410903, 0.000000000000000000, -1.237499998771041110 ) ) ;
#29619=VERTEX_POINT ( 'NONE', #35414 ) ;
#29622=CARTESIAN_POINT ( 'NONE',  ( 10.31873187879411091, -3.604726614523244610, -3.759374999385526106 ) ) ;
#29630=CARTESIAN_POINT ( 'NONE',  ( 22.56230152254411792, 7.347880794884125653E-16, -1.125000000000042633 ) ) ;
#29635=CARTESIAN_POINT ( 'NONE',  ( 22.80587116629410360, 7.646167579472015790E-16, -1.715624999385545468 ) ) ;
#29650=CARTESIAN_POINT ( 'NONE',  ( 10.56230152254410903, 7.347880794884117764E-16, -10.00000000000000000 ) ) ;
#29667=CARTESIAN_POINT ( 'NONE',  ( 19.68408634441910721, 5.407089921784857367, -7.490624999385548044 ) ) ;
#29690=CARTESIAN_POINT ( 'NONE',  ( 10.56230152254410726, 0.000000000000000000, -4.387499998770999277 ) ) ;
#29701=CARTESIAN_POINT ( 'NONE',  ( 22.80587116629410360, 7.646167579472015790E-16, -2.615624999385557370 ) ) ;
#29713=UNCERTAINTY_MEASURE_WITH_UNIT (LENGTH_MEASURE( 1.000000000000000082E-05 ), #36211, 'distance_accuracy_value', 'NONE');
#29731=CARTESIAN_POINT ( 'NONE',  ( 22.80587116629411071, -3.604726614523235284, -4.453124999385550176 ) ) ;
#29737=CARTESIAN_POINT ( 'NONE',  ( 16.56230152254410015, -6.928203230275506996, -6.974999998770984533 ) ) ;
#29743=CARTESIAN_POINT ( 'NONE',  ( 16.56230152254411436, 7.209453229046482114, -3.459374999385518290 ) ) ;
#29749=EDGE_CURVE ( 'NONE', #17848, #26085, #6189, .T. ) ;
#29772=CARTESIAN_POINT ( 'NONE',  ( 10.31873187879410381, 3.604726614523240613, -5.634374999385534544 ) ) ;
#29782=EDGE_CURVE ( 'NONE', #35280, #13088, #453, .T. ) ;
#29792=LINE ( 'NONE', #3824, #30866 ) ;
#29794=CARTESIAN_POINT ( 'NONE',  ( 10.56230152254411614, -3.464101615137761048, -5.812500000000043521 ) ) ;
#29795=ORIENTED_EDGE ( 'NONE', *, *, #26378, .T. ) ;
#29810=CARTESIAN_POINT ( 'NONE',  ( 22.80587116629412847, 3.604726614523243278, -4.884374999385531879 ) ) ;
#29822=CARTESIAN_POINT ( 'NONE',  ( 19.68408634441910721, -5.407089921784855591, -1.790624999385564964 ) ) ;
#29829=CARTESIAN_POINT ( 'NONE',  ( 22.56230152254576637, 3.464101615136798262, -0.9749999987710404881 ) ) ;
#29836=CARTESIAN_POINT ( 'NONE',  ( 22.56230152254411792, 7.347880794884125653E-16, -0.6750000000000366818 ) ) ;
#29853=CARTESIAN_POINT ( 'NONE',  ( 10.31873187879411091, -3.604726614523240613, -7.753124999385540228 ) ) ;
#29857=EDGE_CURVE ( 'NONE', #22453, #26550, #25775, .T. ) ;
#29871=LINE ( 'NONE', #27217, #17599 ) ;
#29872=CARTESIAN_POINT ( 'NONE',  ( 10.56230152254411081, 0.000000000000000000, -4.837499998771033205 ) ) ;
#29894=CARTESIAN_POINT ( 'NONE',  ( 16.56230152254411081, -7.209453229046475009, -3.628124999385552663 ) ) ;
#29898=VECTOR ( 'NONE', #20771, 1000.000000000000000 ) ;
#29899=CARTESIAN_POINT ( 'NONE',  ( 10.31873187879410736, -3.604726614523244610, -9.609374999385535077 ) ) ;
#29923=AXIS2_PLACEMENT_3D ( 'NONE', #2892, #32080, #17503 ) ;
#29927=CARTESIAN_POINT ( 'NONE',  ( 10.31873187879410736, 3.604726614523236616, -5.578124999385555505 ) ) ;
#29928=ADVANCED_FACE ( 'NONE', ( #35319 ), #9374, .F. ) ;
#29932=DIRECTION ( 'NONE',  ( 1.000000000000000000, 0.000000000000000000, 0.000000000000000000 ) ) ;
#29934=CARTESIAN_POINT ( 'NONE',  ( 22.56230152254410370, 7.347880794884117764E-16, -6.412499998770998744 ) ) ;
#29938=CARTESIAN_POINT ( 'NONE',  ( 10.31873187879410558, 3.604726614523240613, -3.384374999385492355 ) ) ;
#29954=CARTESIAN_POINT ( 'NONE',  ( 16.56230152254411436, 7.209453229046475009, -0.2531249993855048674 ) ) ;
#29958=ORIENTED_EDGE ( 'NONE', *, *, #22810, .T. ) ;
#29964=CARTESIAN_POINT ( 'NONE',  ( 22.56230152254511268, 3.464101615137172629, -8.174999998770994480 ) ) ;
#29965=ORIENTED_EDGE ( 'NONE', *, *, #21678, .F. ) ;
#29966=CARTESIAN_POINT ( 'NONE',  ( 19.68408634441911431, 5.407089921784862696, -6.646874999385543603 ) ) ;
#29984=EDGE_CURVE ( 'NONE', #8243, #28841, #31105, .T. ) ;
#29985=CARTESIAN_POINT ( 'NONE',  ( 22.56230152254412502, -3.464101615137755275, -6.562500000000047073 ) ) ;
#29987=ORIENTED_EDGE ( 'NONE', *, *, #22220, .F. ) ;
#30004=CARTESIAN_POINT ( 'NONE',  ( 22.80587116629412847, 3.604726614523243278, -3.984374999385507987 ) ) ;
#30021=DIRECTION ( 'NONE',  ( 1.000000000000000000, 0.000000000000000000, 0.000000000000000000 ) ) ;
#30035=CARTESIAN_POINT ( 'NONE',  ( 10.56230152254470056, 3.464101615138089674, -7.574999998771039245 ) ) ;
#30045=CARTESIAN_POINT ( 'NONE',  ( 10.31873187879411446, 3.604726614523236616, -6.928124999385510741 ) ) ;
#30060=CARTESIAN_POINT ( 'NONE',  ( 22.56230152254410370, 7.347880794884117764E-16, -3.712499998771018106 ) ) ;
#30077=CARTESIAN_POINT ( 'NONE',  ( 22.56230152254411792, 7.347880794884125653E-16, -6.975000000000036948 ) ) ;
#30082=CARTESIAN_POINT ( 'NONE',  ( 22.80587116629410716, 7.646167579472015790E-16, -3.515624999385541294 ) ) ;
#30083=( BOUNDED_CURVE ( )  B_SPLINE_CURVE ( 2, ( #30764, #19777, #5520, #27909, #25256, #36619, #2127, #8385, #1939, #25807, #28094, #17104, #13890, #25438, #22791, #33790, #16920, #37178, #36991, #5342, #28644, #16733, #28461, #11034, #14071, #2497, #13704, #25620, #22608, #34154, #11219, #28279, #34339, #19955, #8200, #2681, #31313, #25065, #10661, #14256, #4968, #19404, #37354, #36806, #11407, #16550, #22977, #30950, #34526, #8566, #10848, #4787, #13509, #22240, #16360, #7828, #22421, #33970, #8010, #19585, #2318, #31135, #5152, #14998, #20324, #6279, #28830, #32239, #26738, #26176, #29202, #32051, #23164, #14438, #26360, #9128, #6081, #2865, #29011, #3055, #12147, #17855, #26551, #771, #20887, #9317, #20133, #20694, #32428, #17288, #14625, #25992, #213, #35262, #22, #15190, #17478, #6473, #3244, #14817, #23723, #578, #29395, #8752, #11588, #3430, #18042, #17666, #29585, #396, #3623, #12340, #11778, #23914, #11963, #23532, #35455, #35078, #31679, #5709, #34705, #5898, #31864, #23344, #34896, #8936, #20513, #35645, #10060, #6844, #33187, #21268, #36020, #13282, #7047, #12535, #24099, #30541, #13096, #7230, #18615, #1149, #18983, #24651, #21455, #29772, #1712, #1339, #26930, #4558, #16133, #15568, #27124, #12909, #24837, #24474, #21822, #21635, #36202, #18803, #9873, #10246, #15948, #3804, #32995, #32806, #3994, #18422, #18232, #9690, #32618, #30157, #29966, #27685, #960, #30345, #4370, #33374, #27502, #15381, #4186, #12719, #1523, #7412, #9505, #21081, #6656, #24288, #15758, #35833, #27309, #22564, #7599, #4746, #5116, #33930, #33562, #14030, #2457, #1899, #13663, #27866, #22381, #25397, #13469, #28243, #19174, #16695, #25581, #7786, #25215, #2089, #16318, #30723, #7971, #31094, #28054, #25021, #10619, #22198, #34111, #19737, #2272, #8163, #37134, #31275, #36766, #28417, #5301, #13850, #16881, #36578, #36947, #10993, #11179, #30904, #33746, #36389, #10435, #10809, #19364, #4925, #22008, #16507, #19545, #7348, #33489, #4493, #1649, #24218, #4673, #29899, #16070, #13221, #18736, #36140, #35763, #10181, #27057, #6978, #30277, #18921, #1460 ),
 .UNSPECIFIED., .F., .F. ) 
 B_SPLINE_CURVE_WITH_KNOTS ( ( 3, 2, 2, 2, 2, 2, 2, 2, 2, 2, 2, 2, 2, 2, 2, 2, 2, 2, 2, 2, 2, 2, 2, 2, 2, 2, 2, 2, 2, 2, 2, 2, 2, 2, 2, 2, 2, 2, 2, 2, 2, 2, 2, 2, 2, 2, 2, 2, 2, 2, 2, 2, 2, 2, 2, 2, 2, 2, 2, 2, 2, 2, 2, 2, 2, 2, 2, 2, 2, 2, 2, 2, 2, 2, 2, 2, 2, 2, 2, 2, 2, 2, 2, 2, 2, 2, 2, 2, 2, 2, 2, 2, 2, 2, 2, 2, 2, 2, 2, 2, 2, 2, 2, 2, 2, 2, 2, 2, 2, 2, 2, 2, 2, 2, 2, 2, 2, 2, 2, 2, 2, 2, 2, 2, 2, 2, 2, 2, 2, 2, 2, 3 ),
 ( 0.000000000000000000, 0.007246376811594202987, 0.01449275362318840597, 0.02173913043478260809, 0.02898550724637681195, 0.03623188405797101580, 0.04347826086956521618, 0.05072463768115942351, 0.05797101449275362389, 0.06521739130434782428, 0.07246376811594203160, 0.07971014492753622505, 0.08695652173913043237, 0.09420289855072463969, 0.1014492753623188470, 0.1086956521739130405, 0.1159420289855072478, 0.1231884057971014551, 0.1304347826086956486, 0.1376811594202898559, 0.1449275362318840632, 0.1521739130434782705, 0.1594202898550724501, 0.1666666666666666574, 0.1739130434782608647, 0.1811594202898550721, 0.1884057971014492794, 0.1956521739130434867, 0.2028985507246376940, 0.2101449275362318736, 0.2173913043478260809, 0.2246376811594202882, 0.2318840579710144956, 0.2391304347826087029, 0.2463768115942029102, 0.2536231884057971175, 0.2608695652173912971, 0.2681159420289855322, 0.2753623188405797118, 0.2826086956521738358, 0.2898550724637681264, 0.2971014492753623060, 0.3043478260869565410, 0.3115942028985507206, 0.3188405797101449002, 0.3260869565217391353, 0.3333333333333333148, 0.3405797101449275499, 0.3478260869565217295, 0.3550724637681159646, 0.3623188405797101441, 0.3695652173913043237, 0.3768115942028985588, 0.3840579710144927383, 0.3913043478260869734, 0.3985507246376811530, 0.4057971014492753881, 0.4130434782608695676, 0.4202898550724637472, 0.4275362318840579268, 0.4347826086956521618, 0.4420289855072463969, 0.4492753623188405765, 0.4565217391304347561, 0.4637681159420289911, 0.4710144927536231707, 0.4782608695652174058, 0.4855072463768115854, 0.4927536231884058204, 0.5000000000000000000, 0.5072463768115942351, 0.5144927536231883591, 0.5217391304347825942, 0.5289855072463768293, 0.5362318840579710644, 0.5434782608695651884, 0.5507246376811594235, 0.5579710144927536586, 0.5652173913043476716, 0.5724637681159420177, 0.5797101449275362528, 0.5869565217391304879, 0.5942028985507246119, 0.6014492753623188470, 0.6086956521739130821, 0.6159420289855072062, 0.6231884057971014412, 0.6304347826086956763, 0.6376811594202898004, 0.6449275362318841465, 0.6521739130434782705, 0.6594202898550725056, 0.6666666666666666297, 0.6739130434782608647, 0.6811594202898550998, 0.6884057971014492239, 0.6956521739130434590, 0.7028985507246376940, 0.7101449275362319291, 0.7173913043478260532, 0.7246376811594202882, 0.7318840579710145233, 0.7391304347826086474, 0.7463768115942028825, 0.7536231884057971175, 0.7608695652173913526, 0.7681159420289854767, 0.7753623188405797118, 0.7826086956521739468, 0.7898550724637680709, 0.7971014492753623060, 0.8043478260869565410, 0.8115942028985507761, 0.8188405797101449002, 0.8260869565217391353, 0.8333333333333333703, 0.8405797101449274944, 0.8478260869565217295, 0.8550724637681158535, 0.8623188405797101996, 0.8695652173913043237, 0.8768115942028985588, 0.8840579710144927938, 0.8913043478260869179, 0.8985507246376811530, 0.9057971014492753881, 0.9130434782608695121, 0.9202898550724637472, 0.9275362318840579823, 0.9347826086956523284, 0.9420289855072463414, 0.9470763321615516261 ),
 .UNSPECIFIED. ) 
 CURVE ( )  GEOMETRIC_REPRESENTATION_ITEM ( )  RATIONAL_B_SPLINE_CURVE ( ( 1.000000000000000000, 0.8660254037844387076, 1.000000000000000000, 0.8660254037844387076, 1.000000000000000000, 0.8660254037844387076, 1.000000000000000000, 0.8660254037844387076, 1.000000000000000000, 0.8660254037844387076, 1.000000000000000000, 0.8660254037844387076, 1.000000000000000000, 0.8660254037844387076, 1.000000000000000000, 0.8660254037844387076, 1.000000000000000000, 0.8660254037844387076, 1.000000000000000000, 0.8660254037844387076, 1.000000000000000000, 0.8660254037844387076, 1.000000000000000000, 0.8660254037844387076, 1.000000000000000000, 0.8660254037844387076, 1.000000000000000000, 0.8660254037844387076, 1.000000000000000000, 0.8660254037844387076, 1.000000000000000000, 0.8660254037844387076, 1.000000000000000000, 0.8660254037844387076, 1.000000000000000000, 0.8660254037844387076, 1.000000000000000000, 0.8660254037844387076, 1.000000000000000000, 0.8660254037844387076, 1.000000000000000000, 0.8660254037844387076, 1.000000000000000000, 0.8660254037844387076, 1.000000000000000000, 0.8660254037844387076, 1.000000000000000000, 0.8660254037844387076, 1.000000000000000000, 0.8660254037844387076, 1.000000000000000000, 0.8660254037844387076, 1.000000000000000000, 0.8660254037844387076, 1.000000000000000000, 0.8660254037844387076, 1.000000000000000000, 0.8660254037844387076, 1.000000000000000000, 0.8660254037844387076, 1.000000000000000000, 0.8660254037844387076, 1.000000000000000000, 0.8660254037844387076, 1.000000000000000000, 0.8660254037844387076, 1.000000000000000000, 0.8660254037844387076, 1.000000000000000000, 0.8660254037844387076, 1.000000000000000000, 0.8660254037844387076, 1.000000000000000000, 0.8660254037844387076, 1.000000000000000000, 0.8660254037844387076, 1.000000000000000000, 0.8660254037844387076, 1.000000000000000000, 0.8660254037844387076, 1.000000000000000000, 0.8660254037844387076, 1.000000000000000000, 0.8660254037844387076, 1.000000000000000000, 0.8660254037844387076, 1.000000000000000000, 0.8660254037844387076, 1.000000000000000000, 0.8660254037844387076, 1.000000000000000000, 0.8660254037844387076, 1.000000000000000000, 0.8660254037844387076, 1.000000000000000000, 0.8660254037844387076, 1.000000000000000000, 0.8660254037844387076, 1.000000000000000000, 0.8660254037844387076, 1.000000000000000000, 0.8660254037844387076, 1.000000000000000000, 0.8660254037844387076, 1.000000000000000000, 0.8660254037844387076, 1.000000000000000000, 0.8660254037844387076, 1.000000000000000000, 0.8660254037844387076, 1.000000000000000000, 0.8660254037844387076, 1.000000000000000000, 0.8660254037844387076, 1.000000000000000000, 0.8660254037844387076, 1.000000000000000000, 0.8660254037844387076, 1.000000000000000000, 0.8660254037844387076, 1.000000000000000000, 0.8660254037844387076, 1.000000000000000000, 0.8660254037844387076, 1.000000000000000000, 0.8660254037844387076, 1.000000000000000000, 0.8660254037844387076, 1.000000000000000000, 0.8660254037844387076, 1.000000000000000000, 0.8660254037844387076, 1.000000000000000000, 0.8660254037844387076, 1.000000000000000000, 0.8660254037844387076, 1.000000000000000000, 0.8660254037844387076, 1.000000000000000000, 0.8660254037844387076, 1.000000000000000000, 0.8660254037844387076, 1.000000000000000000, 0.8660254037844387076, 1.000000000000000000, 0.8660254037844387076, 1.000000000000000000, 0.8660254037844387076, 1.000000000000000000, 0.8660254037844387076, 1.000000000000000000, 0.8660254037844387076, 1.000000000000000000, 0.8660254037844387076, 1.000000000000000000, 0.8660254037844387076, 1.000000000000000000, 0.8660254037844387076, 1.000000000000000000, 0.8660254037844387076, 1.000000000000000000, 0.8660254037844387076, 1.000000000000000000, 0.8660254037844387076, 1.000000000000000000, 0.8660254037844387076, 1.000000000000000000, 0.8660254037844387076, 1.000000000000000000, 0.8660254037844387076, 1.000000000000000000, 0.8660254037844387076, 1.000000000000000000, 0.8660254037844387076, 1.000000000000000000, 0.8660254037844387076, 1.000000000000000000, 0.8660254037844387076, 1.000000000000000000, 0.8660254037844387076, 1.000000000000000000, 0.8660254037844387076, 1.000000000000000000, 0.8660254037844387076, 1.000000000000000000, 0.8660254037844387076, 1.000000000000000000, 0.8660254037844387076, 1.000000000000000000, 0.8660254037844387076, 1.000000000000000000, 0.8660254037844387076, 1.000000000000000000, 0.8660254037844387076, 1.000000000000000000, 0.8660254037844387076, 1.000000000000000000, 0.8660254037844387076, 1.000000000000000000, 0.8660254037844387076, 1.000000000000000000, 0.8660254037844387076, 1.000000000000000000, 0.8660254037844387076, 1.000000000000000000, 0.8660254037844387076, 1.000000000000000000, 0.8660254037844387076, 1.000000000000000000, 0.8660254037844387076, 1.000000000000000000, 0.8660254037844387076, 1.000000000000000000, 0.8660254037844387076, 1.000000000000000000, 0.8660254037844387076, 1.000000000000000000, 0.8660254037844387076, 1.000000000000000000, 0.8660254037844387076, 1.000000000000000000, 0.8660254037844387076, 1.000000000000000000, 0.8660254037844387076, 1.000000000000000000, 0.8660254037844387076, 1.000000000000000000, 0.8660254037844387076, 1.000000000000000000, 0.8660254037844387076, 1.000000000000000000, 0.8660254037844387076, 1.000000000000000000, 0.8660254037844387076, 1.000000000000000000, 0.8660254037844387076, 1.000000000000000000, 0.8660254037844387076, 1.000000000000000000, 0.8660254037844387076, 1.000000000000000000, 0.8660254037844387076, 1.000000000000000000, 0.8660254037844387076, 1.000000000000000000, 0.8660254037844387076, 1.000000000000000000, 0.8660254037844387076, 1.000000000000000000, 0.8660254037844387076, 1.000000000000000000, 0.8660254037844387076, 1.000000000000000000, 0.8660254037844387076, 1.000000000000000000, 0.8660254037844387076, 1.000000000000000000, 0.8660254037844387076, 1.000000000000000000, 0.8660254037844387076, 1.000000000000000000, 0.9066821602640693367, 0.9433623867133065222 ) ) 
 REPRESENTATION_ITEM ( '' )  );
#30095=EDGE_LOOP ( 'NONE', ( #36837, #17559, #1613, #25734 ) ) ;
#30106=ORIENTED_EDGE ( 'NONE', *, *, #12616, .F. ) ;
#30109=CARTESIAN_POINT ( 'NONE',  ( 22.56230152254257604, -3.464101615138639900, -9.149999998771018994 ) ) ;
#30118=CARTESIAN_POINT ( 'NONE',  ( 16.56230152254411436, -7.209453229046475009, -7.228124999385518556 ) ) ;
#30123=CARTESIAN_POINT ( 'NONE',  ( 19.56230152254411792, -5.196152422706629359, -6.937499998771023968 ) ) ;
#30126=CARTESIAN_POINT ( 'NONE',  ( 22.80587116629412137, 7.646167579472024665E-16, -3.121874999385543248 ) ) ;
#30150=( BOUNDED_CURVE ( )  B_SPLINE_CURVE ( 2, ( #945, #14610, #6265, #12520, #6642, #383, #26347 ),
 .UNSPECIFIED., .F., .F. ) 
 B_SPLINE_CURVE_WITH_KNOTS ( ( 3, 2, 2, 3 ),
 ( 0.7391304347826079812, 0.7463768115942022163, 0.7536231884057965624, 0.7608695652173907975 ),
 .UNSPECIFIED. ) 
 CURVE ( )  GEOMETRIC_REPRESENTATION_ITEM ( )  RATIONAL_B_SPLINE_CURVE ( ( 1.000000000000012212, 0.8660254037844263841, 1.000000000000000000, 0.8660254037844387076, 1.000000000000000000, 0.8660254037844489217, 0.9999999999999897859 ) ) 
 REPRESENTATION_ITEM ( '' )  );
#30157=CARTESIAN_POINT ( 'NONE',  ( 16.56230152254411436, 7.209453229046482114, -6.609374999385521754 ) ) ;
#30164=SURFACE_SIDE_STYLE ('',( #18622 ) ) ;
#30169=ORIENTED_EDGE ( 'NONE', *, *, #22645, .T. ) ;
#30176=CARTESIAN_POINT ( 'NONE',  ( 10.56230152254410548, 3.464101615137757051, -7.687500000000020428 ) ) ;
#30178=VECTOR ( 'NONE', #18401, 1000.000000000000227 ) ;
#30187=CARTESIAN_POINT ( 'NONE',  ( 22.56230152254411792, 7.347880794884125653E-16, -5.625000000000018652 ) ) ;
#30193=CARTESIAN_POINT ( 'NONE',  ( 10.31873187879410558, -3.604726614523244610, -4.209374999385490312 ) ) ;
#30201=EDGE_CURVE ( 'NONE', #21112, #3622, #35968, .T. ) ;
#30218=EDGE_CURVE ( 'NONE', #20931, #25619, #19504, .T. ) ;
#30228=ADVANCED_FACE ( 'NONE', ( #19597 ), #7653, .F. ) ;
#30236=CARTESIAN_POINT ( 'NONE',  ( 22.80587116629411071, -3.604726614523235284, -7.153124999385556571 ) ) ;
#30266=EDGE_CURVE ( 'NONE', #35280, #18752, #25557, .T. ) ;
#30274=CARTESIAN_POINT ( 'NONE',  ( 10.31873187879410914, 0.000000000000000000, -3.290624999385538541 ) ) ;
#30277=CARTESIAN_POINT ( 'NONE',  ( 19.68408634441911431, -5.407089921784861808, -9.946874999385540761 ) ) ;
#30295=ORIENTED_EDGE ( 'NONE', *, *, #35212, .T. ) ;
#30306=CARTESIAN_POINT ( 'NONE',  ( 19.68408634441910721, -5.407089921784855591, -8.540624999385542537 ) ) ;
#30312=CARTESIAN_POINT ( 'NONE',  ( 16.56230152254411436, -6.928203230275506996, -7.424999998770979381 ) ) ;
#30315=CARTESIAN_POINT ( 'NONE',  ( 16.56230152254411436, -7.209453229046482114, -3.234374999385536853 ) ) ;
#30324=VECTOR ( 'NONE', #35462, 1000.000000000000000 ) ;
#30325=ORIENTED_EDGE ( 'NONE', *, *, #35174, .F. ) ;
#30332=CARTESIAN_POINT ( 'NONE',  ( 10.31873187879411091, 0.000000000000000000, -2.840624999385532590 ) ) ;
#30333=( BOUNDED_CURVE ( )  B_SPLINE_CURVE ( 2, ( #12132, #1134, #15176, #23899, #20875, #756, #12326 ),
 .UNSPECIFIED., .F., .F. ) 
 B_SPLINE_CURVE_WITH_KNOTS ( ( 3, 2, 2, 3 ),
 ( 0.5217391304347842595, 0.5289855072463786057, 0.5362318840579728407, 0.5434782608695670758 ),
 .UNSPECIFIED. ) 
 CURVE ( )  GEOMETRIC_REPRESENTATION_ITEM ( )  RATIONAL_B_SPLINE_CURVE ( ( 0.9999999999999692468, 0.8660254037844694608, 1.000000000000000000, 0.8660254037844387076, 1.000000000000000000, 0.8660254037844038466, 1.000000000000034861 ) ) 
 REPRESENTATION_ITEM ( '' )  );
#30345=CARTESIAN_POINT ( 'NONE',  ( 22.80587116629411781, -3.604726614523238837, -6.759374999385540761 ) ) ;
#30358=CARTESIAN_POINT ( 'NONE',  ( 15.47812160658635428, 6.148716598298411107, -10.19635144101486368 ) ) ;
#30359=ORIENTED_EDGE ( 'NONE', *, *, #12928, .F. ) ;
#30366=CARTESIAN_POINT ( 'NONE',  ( 10.56230152254410548, 0.000000000000000000, -9.450000000000041922 ) ) ;
#30384=CARTESIAN_POINT ( 'NONE',  ( 10.31873187879411091, -3.604726614523244610, -5.109374999385544847 ) ) ;
#30401=DIRECTION ( 'NONE',  ( 0.000000000000000000, 0.000000000000000000, 1.000000000000000000 ) ) ;
#30414=( BOUNDED_CURVE ( )  B_SPLINE_CURVE ( 2, ( #14053, #3036, #16900, #3224, #8731, #19938, #19757 ),
 .UNSPECIFIED., .F., .F. ) 
 B_SPLINE_CURVE_WITH_KNOTS ( ( 3, 2, 2, 3 ),
 ( 0.4130434782608723432, 0.4202898550724666338, 0.4275362318840610354, 0.4347826086956553260 ),
 .UNSPECIFIED. ) 
 CURVE ( )  GEOMETRIC_REPRESENTATION_ITEM ( )  RATIONAL_B_SPLINE_CURVE ( ( 0.9999999999999487077, 0.8660254037844899999, 1.000000000000000000, 0.8660254037844387076, 1.000000000000000000, 0.8660254037843801989, 1.000000000000058620 ) ) 
 REPRESENTATION_ITEM ( '' )  );
#30423=EDGE_CURVE ( 'NONE', #24827, #28622, #3751, .T. ) ;
#30428=CARTESIAN_POINT ( 'NONE',  ( 22.80587116629410716, 7.646167579472015790E-16, -6.215624999385549465 ) ) ;
#30436=EDGE_LOOP ( 'NONE', ( #10280, #6280, #23242, #17964 ) ) ;
#30468=CARTESIAN_POINT ( 'NONE',  ( 16.56230152254411436, 7.209453229046475009, -3.853124999385534988 ) ) ;
#30477=CARTESIAN_POINT ( 'NONE',  ( 10.31873187879410736, 0.000000000000000000, -1.096874999385516469 ) ) ;
#30500=CARTESIAN_POINT ( 'NONE',  ( 22.80587116629411071, -3.604726614523235284, -8.503124999385544669 ) ) ;
#30506=CARTESIAN_POINT ( 'NONE',  ( 10.56230152254411436, 3.464101615137752166, -7.574999998771032139 ) ) ;
#30510=CARTESIAN_POINT ( 'NONE',  ( 10.31873187879411091, -3.604726614523244610, -6.009374999385537208 ) ) ;
#30521=EDGE_CURVE ( 'NONE', #34832, #18566, #18047, .T. ) ;
#30541=CARTESIAN_POINT ( 'NONE',  ( 22.80587116629411781, 3.604726614523243278, -5.334374999385495641 ) ) ;
#30553=CARTESIAN_POINT ( 'NONE',  ( 22.56230152254410370, 7.347880794884117764E-16, -1.912499998771022280 ) ) ;
#30556=CARTESIAN_POINT ( 'NONE',  ( 10.56230152254410548, 0.000000000000000000, -9.000000000000035527 ) ) ;
#30562=CARTESIAN_POINT ( 'NONE',  ( 13.56230152254411792, -5.196152422706638241, -8.925000000000071765 ) ) ;
#30579=CARTESIAN_POINT ( 'NONE',  ( 13.44051670066910731, 5.407089921784862696, -5.221874999385534011 ) ) ;
#30583=ORIENTED_EDGE ( 'NONE', *, *, #26822, .T. ) ;
#30589=DIRECTION ( 'NONE',  ( 0.08715574274765143514, 0.000000000000000000, -0.9961946980917461003 ) ) ;
#30597=( BOUNDED_CURVE ( )  B_SPLINE_CURVE ( 2, ( #11935, #23138, #20485, #25081, #28804, #34680, #8725 ),
 .UNSPECIFIED., .F., .F. ) 
 B_SPLINE_CURVE_WITH_KNOTS ( ( 3, 2, 2, 3 ),
 ( 0.7826086956521710603, 0.7898550724637652953, 0.7971014492753596414, 0.8043478260869539875 ),
 .UNSPECIFIED. ) 
 CURVE ( )  GEOMETRIC_REPRESENTATION_ITEM ( )  RATIONAL_B_SPLINE_CURVE ( ( 1.000000000000053291, 0.8660254037843853059, 1.000000000000000000, 0.8660254037844387076, 1.000000000000000000, 0.8660254037844858921, 0.9999999999999528155 ) ) 
 REPRESENTATION_ITEM ( '' )  );
#30601=CARTESIAN_POINT ( 'NONE',  ( 22.56230152254412857, -3.464101615137755275, -2.062499999999993339 ) ) ;
#30608=CARTESIAN_POINT ( 'NONE',  ( 22.56230152254410015, 7.347880794884117764E-16, -7.762499998770988618 ) ) ;
#30617=CARTESIAN_POINT ( 'NONE',  ( 13.44051670066911619, -5.407089921784859143, -9.065624999385569538 ) ) ;
#30626=CARTESIAN_POINT ( 'NONE',  ( 22.56230152254410370, 0.000000000000000000, -10.00000000000000000 ) ) ;
#30644=ORIENTED_EDGE ( 'NONE', *, *, #18712, .F. ) ;
#30654=CARTESIAN_POINT ( 'NONE',  ( 22.80587116629411781, 3.604726614523238837, -4.378124999385524241 ) ) ;
#30662=CARTESIAN_POINT ( 'NONE',  ( 10.31873187879410736, 3.604726614523240613, -1.584374999385509630 ) ) ;
#30674=ORIENTED_EDGE ( 'NONE', *, *, #24687, .T. ) ;
#30684=CARTESIAN_POINT ( 'NONE',  ( 22.80587116629410360, 3.604726614523238837, -8.428124999385516958 ) ) ;
#30690=CARTESIAN_POINT ( 'NONE',  ( 19.56230152254410370, 5.196152422706631135, -8.587499998771008336 ) ) ;
#30695=CARTESIAN_POINT ( 'NONE',  ( 19.68408634441912142, -5.407089921784861808, -7.246874999385532590 ) ) ;
#30706=EDGE_CURVE ( 'NONE', #11580, #28711, #29426, .T. ) ;
#30721=CARTESIAN_POINT ( 'NONE',  ( 19.56230152254412147, -5.196152422706635576, -0.3000000000000779821 ) ) ;
#30723=CARTESIAN_POINT ( 'NONE',  ( 16.56230152254411081, -7.209453229046482114, -8.184374999385489957 ) ) ;
#30727=CARTESIAN_POINT ( 'NONE',  ( 16.56230152254411436, 7.209453229046475009, -1.603124999385524108 ) ) ;
#30732=EDGE_CURVE ( 'NONE', #28398, #21699, #18297, .T. ) ;
#30735=CARTESIAN_POINT ( 'NONE',  ( 16.56230152254411081, -6.928203230275506996, -0.6749999987709800475 ) ) ;
#30736=ORIENTED_EDGE ( 'NONE', *, *, #33797, .F. ) ;
#30738=CARTESIAN_POINT ( 'NONE',  ( 10.56230152254491195, -3.464101615138220236, -8.962500000000034106 ) ) ;
#30743=CARTESIAN_POINT ( 'NONE',  ( 10.56230152254410903, -3.464101615137761048, -9.862500000000036238 ) ) ;
#30759=CARTESIAN_POINT ( 'NONE',  ( 13.44051670066910731, 5.407089921784862696, -7.471874999385508254 ) ) ;
#30764=CARTESIAN_POINT ( 'NONE',  ( 10.31873187879410914, 0.000000000000000000, -0.1968749993855323233 ) ) ;
#30766=CARTESIAN_POINT ( 'NONE',  ( 22.56230152254410726, 7.347880794884117764E-16, -9.562499998771039955 ) ) ;
#30768=FACE_OUTER_BOUND ( 'NONE', #24738, .T. ) ;
#30770=EDGE_CURVE ( 'NONE', #32942, #20931, #12952, .T. ) ;
#30780=CARTESIAN_POINT ( 'NONE',  ( 22.56230152254411436, 3.464101615137759271, -2.437500000000027534 ) ) ;
#30782=EDGE_LOOP ( 'NONE', ( #11427, #11885, #36804, #24136 ) ) ;
#30796=CARTESIAN_POINT ( 'NONE',  ( 16.56230152254411436, -7.209453229046475009, -9.928124999385525840 ) ) ;
#30820=ADVANCED_FACE ( 'NONE', ( #36924 ), #31618, .F. ) ;
#30834=CARTESIAN_POINT ( 'NONE',  ( 19.68408634441910365, -5.407089921784855591, -5.840624999385535254 ) ) ;
#30843=CARTESIAN_POINT ( 'NONE',  ( 13.44051670066911264, -5.407089921784865361, -1.471874999385502925 ) ) ;
#30864=CARTESIAN_POINT ( 'NONE',  ( 16.56230152254411436, 7.209453229046475009, -7.003124999385537564 ) ) ;
#30866=VECTOR ( 'NONE', #35472, 1000.000000000000000 ) ;
#30871=CARTESIAN_POINT ( 'NONE',  ( 13.56230152254410370, 5.196152422706630247, -9.412499998771028942 ) ) ;
#30875=CARTESIAN_POINT ( 'NONE',  ( 22.80587116629411781, 7.646167579472024665E-16, -5.821874999385522997 ) ) ;
#30878=DIRECTION ( 'NONE',  ( -1.000000000000000000, 0.000000000000000000, 0.000000000000000000 ) ) ;
#30881=CARTESIAN_POINT ( 'NONE',  ( 22.56230152254411792, 7.347880794884125653E-16, -4.725000000000035172 ) ) ;
#30902=CARTESIAN_POINT ( 'NONE',  ( 19.56230152254411792, 5.196152422706637353, -2.400000000000013234 ) ) ;
#30904=CARTESIAN_POINT ( 'NONE',  ( 22.80587116629412492, -3.604726614523238837, -9.009374999385519445 ) ) ;
#30909=CARTESIAN_POINT ( 'NONE',  ( 16.56230152254411436, 7.209453229046475009, -0.2531249993855048674 ) ) ;
#30913=CARTESIAN_POINT ( 'NONE',  ( 19.56230152254411792, -5.196152422706629359, -2.887499998771053455 ) ) ;
#30916=CARTESIAN_POINT ( 'NONE',  ( 19.56230152254410726, 5.196152422706631135, -0.4874999987710126881 ) ) ;
#30922=CARTESIAN_POINT ( 'NONE',  ( 13.56230152254411792, -5.196152422706638241, -8.925000000000071765 ) ) ;
#30926=CARTESIAN_POINT ( 'NONE',  ( 16.56230152254411436, 6.928203230275514990, -8.212500000000009237 ) ) ;
#30935=DIRECTION ( 'NONE',  ( 0.000000000000000000, 0.000000000000000000, 1.000000000000000000 ) ) ;
#30938=CARTESIAN_POINT ( 'NONE',  ( 22.56230152254410370, 7.347880794884117764E-16, -2.362499998771028231 ) ) ;
#30943=CARTESIAN_POINT ( 'NONE',  ( 22.80587116629411781, 3.604726614523243278, -5.334374999385495641 ) ) ;
#30950=CARTESIAN_POINT ( 'NONE',  ( 10.31873187879410736, -3.604726614523244610, -1.959374999385511185 ) ) ;
#30952=EDGE_CURVE ( 'NONE', #26216, #33455, #28428, .T. ) ;
#30965=AXIS2_PLACEMENT_3D ( 'NONE', #20408, #853, #26078 ) ;
#30968=CARTESIAN_POINT ( 'NONE',  ( 22.56230152254411792, 3.464101615137759271, -2.887500000000023270 ) ) ;
#30969=ADVANCED_FACE ( 'NONE', ( #14194 ), #11347, .F. ) ;
#30984=CARTESIAN_POINT ( 'NONE',  ( 22.56230152254411792, 7.347880794884125653E-16, -6.975000000000036948 ) ) ;
#30988=CARTESIAN_POINT ( 'NONE',  ( 10.31873187879411091, 3.604726614523236616, -8.278124999385530813 ) ) ;
#30995=ORIENTED_EDGE ( 'NONE', *, *, #23537, .F. ) ;
#31017=FACE_OUTER_BOUND ( 'NONE', #30436, .T. ) ;
#31021=EDGE_CURVE ( 'NONE', #36053, #19993, #4246, .T. ) ;
#31022=CARTESIAN_POINT ( 'NONE',  ( 19.68408634441910721, -5.407089921784855591, -7.640624999385531524 ) ) ;
#31031=CARTESIAN_POINT ( 'NONE',  ( 16.56230152254411436, -7.209453229046482114, -2.334374999385512961 ) ) ;
#31037=CARTESIAN_POINT ( 'NONE',  ( 22.80587116629410716, 7.646167579472015790E-16, -1.265624999385539518 ) ) ;
#31060=CARTESIAN_POINT ( 'NONE',  ( 22.56230152254410015, 7.347880794884117764E-16, -7.312499998771010645 ) ) ;
#31064=CARTESIAN_POINT ( 'NONE',  ( 10.31873187879410736, 3.604726614523240613, -7.434374999385486404 ) ) ;
#31066=LINE ( 'NONE', #36176, #27237 ) ;
#31069=CARTESIAN_POINT ( 'NONE',  ( 22.56230152254411792, 7.347880794884125653E-16, -6.075000000000052580 ) ) ;
#31071=LINE ( 'NONE', #22358, #21526 ) ;
#31084=ORIENTED_EDGE ( 'NONE', *, *, #33003, .F. ) ;
#31090=( BOUNDED_CURVE ( )  B_SPLINE_CURVE ( 2, ( #37183, #36812, #33795, #22797, #10854, #28467, #36996 ),
 .UNSPECIFIED., .F., .F. ) 
 B_SPLINE_CURVE_WITH_KNOTS ( ( 3, 2, 2, 3 ),
 ( 0.2608695652173921298, 0.2681159420289864204, 0.2753623188405807110, 0.2826086956521749460 ),
 .UNSPECIFIED. ) 
 CURVE ( )  GEOMETRIC_REPRESENTATION_ITEM ( )  RATIONAL_B_SPLINE_CURVE ( ( 0.9999999999999845679, 0.8660254037844541397, 1.000000000000000000, 0.8660254037844387076, 1.000000000000000000, 0.8660254037844191677, 1.000000000000019540 ) ) 
 REPRESENTATION_ITEM ( '' )  );
#31091=CARTESIAN_POINT ( 'NONE',  ( 19.56230152254412147, -5.196152422706635576, -9.750000000000063949 ) ) ;
#31094=CARTESIAN_POINT ( 'NONE',  ( 10.31873187879410736, -3.604726614523244610, -8.259374999385515892 ) ) ;
#31097=CARTESIAN_POINT ( 'NONE',  ( 10.31873187879411091, -3.604726614523240613, -2.353124999385527882 ) ) ;
#31101=CARTESIAN_POINT ( 'NONE',  ( 19.56230152254411792, -5.196152422706629359, -7.387499998771030363 ) ) ;
#31104=CARTESIAN_POINT ( 'NONE',  ( 16.56230152254411081, -6.928203230275506996, -1.124999998771007759 ) ) ;
#31105=( BOUNDED_CURVE ( )  B_SPLINE_CURVE ( 2, ( #21322, #29454, #18481, #32862, #32481, #12398, #32672 ),
 .UNSPECIFIED., .F., .F. ) 
 B_SPLINE_CURVE_WITH_KNOTS ( ( 3, 2, 2, 3 ),
 ( 0.6956521739130421267, 0.7028985507246364728, 0.7101449275362307079, 0.7173913043478249429 ),
 .UNSPECIFIED. ) 
 CURVE ( )  GEOMETRIC_REPRESENTATION_ITEM ( )  RATIONAL_B_SPLINE_CURVE ( ( 1.000000000000024647, 0.8660254037844140607, 1.000000000000000000, 0.8660254037844387076, 1.000000000000000000, 0.8660254037844592467, 0.9999999999999794609 ) ) 
 REPRESENTATION_ITEM ( '' )  );
#31112=CARTESIAN_POINT ( 'NONE',  ( 13.56230152254411614, -5.196152422706638241, -8.475000000000093792 ) ) ;
#31121=CARTESIAN_POINT ( 'NONE',  ( 22.56230152254410370, 0.000000000000000000, -10.00000000000000000 ) ) ;
#31123=LINE ( 'NONE', #4952, #3498 ) ;
#31125=CARTESIAN_POINT ( 'NONE',  ( 13.56230152254410726, 5.196152422706636465, -3.675000000000067324 ) ) ;
#31128=VERTEX_POINT ( 'NONE', #35201 ) ;
#31131=CARTESIAN_POINT ( 'NONE',  ( 16.56230152254411436, 7.209453229046482114, -6.159374999385525129 ) ) ;
#31135=CARTESIAN_POINT ( 'NONE',  ( 10.31873187879410381, 3.604726614523240613, -2.484374999385501326 ) ) ;
#31136=CARTESIAN_POINT ( 'NONE',  ( 22.56230152254410370, 0.000000000000000000, -10.00000000000000000 ) ) ;
#31146=CARTESIAN_POINT ( 'NONE',  ( 16.56230152254410726, 0.000000000000000000, -10.00000000000000000 ) ) ;
#31153=CARTESIAN_POINT ( 'NONE',  ( 16.56230152254411436, -6.928203230275514990, -3.037500000000043165 ) ) ;
#31168=CARTESIAN_POINT ( 'NONE',  ( 19.56230152254412502, -5.196152422706635576, -7.050000000000084199 ) ) ;
#31172=CARTESIAN_POINT ( 'NONE',  ( 22.80587116629411071, 3.604726614523238837, -9.778124999385537919 ) ) ;
#31204=CARTESIAN_POINT ( 'NONE',  ( 22.80587116629411071, -3.604726614523235284, -7.603124999385552307 ) ) ;
#31211=CARTESIAN_POINT ( 'NONE',  ( 10.31873187879410914, 0.000000000000000000, -0.1968749993855323233 ) ) ;
#31217=CARTESIAN_POINT ( 'NONE',  ( 10.31873187879410736, 3.604726614523236616, -1.978124999385525662 ) ) ;
#31241=CARTESIAN_POINT ( 'NONE',  ( 10.56230152254411259, -3.464101615137757051, -9.749999998770984888 ) ) ;
#31244=CARTESIAN_POINT ( 'NONE',  ( 19.83830452692372148, 6.917534487978463709, -10.24872752355802064 ) ) ;
#31245=CARTESIAN_POINT ( 'NONE',  ( 13.44051670066910908, 5.407089921784862696, -6.571874999385523886 ) ) ;
#31261=DIRECTION ( 'NONE',  ( 0.000000000000000000, 0.000000000000000000, 1.000000000000000000 ) ) ;
#31273=CARTESIAN_POINT ( 'NONE',  ( 22.56230152254432042, 3.464101615137637147, -2.437500000000029310 ) ) ;
#31275=CARTESIAN_POINT ( 'NONE',  ( 16.56230152254411436, -7.209453229046482114, -8.634374999385517668 ) ) ;
#31278=CARTESIAN_POINT ( 'NONE',  ( 16.56230152254411081, -7.209453229046475009, -2.728124999385529215 ) ) ;
#31284=CARTESIAN_POINT ( 'NONE',  ( 13.56230152254410726, 5.196152422706630247, -3.112499998771029119 ) ) ;
#31293=CARTESIAN_POINT ( 'NONE',  ( 22.80587116629410360, 7.646167579472015790E-16, -1.715624999385545468 ) ) ;
#31294=DIRECTION ( 'NONE',  ( 0.000000000000000000, 0.000000000000000000, 1.000000000000000000 ) ) ;
#31309=CARTESIAN_POINT ( 'NONE',  ( 22.80587116629411781, -3.604726614523238837, -7.209374999385536498 ) ) ;
#31313=CARTESIAN_POINT ( 'NONE',  ( 10.31873187879410558, 0.000000000000000000, -1.546874999385550176 ) ) ;
#31330=CARTESIAN_POINT ( 'NONE',  ( 10.56230152254410726, 0.000000000000000000, -3.150000000000041656 ) ) ;
#31348=CARTESIAN_POINT ( 'NONE',  ( 10.31873187879410381, 3.604726614523240613, -0.2343749993854903346 ) ) ;
#31353=ORIENTED_EDGE ( 'NONE', *, *, #35141, .T. ) ;
#31359=( BOUNDED_CURVE ( )  B_SPLINE_CURVE ( 2, ( #28351, #36320, #21755, #25143, #19665, #19105, #22128 ),
 .UNSPECIFIED., .F., .F. ) 
 B_SPLINE_CURVE_WITH_KNOTS ( ( 3, 2, 2, 3 ),
 ( 0.7173913043478249429, 0.7246376811594192890, 0.7318840579710137462, 0.7391304347826079812 ),
 .UNSPECIFIED. ) 
 CURVE ( )  GEOMETRIC_REPRESENTATION_ITEM ( )  RATIONAL_B_SPLINE_CURVE ( ( 1.000000000000020428, 0.8660254037844181685, 1.000000000000000000, 0.8660254037844387076, 1.000000000000000000, 0.8660254037844510311, 0.9999999999999876765 ) ) 
 REPRESENTATION_ITEM ( '' )  );
#31387=CARTESIAN_POINT ( 'NONE',  ( 19.68408634441910721, 5.407089921784857367, -6.140624999385558169 ) ) ;
#31397=CARTESIAN_POINT ( 'NONE',  ( 13.44051670066911086, -5.407089921784865361, -2.821874999385520777 ) ) ;
#31403=CARTESIAN_POINT ( 'NONE',  ( 22.80587116629410716, 3.604726614523238837, -2.578124999385541738 ) ) ;
#31408=ORIENTED_EDGE ( 'NONE', *, *, #20954, .T. ) ;
#31409=ORIENTED_EDGE ( 'NONE', *, *, #20778, .T. ) ;
#31417=CYLINDRICAL_SURFACE ( 'NONE', #17994, 5.999999999999998224 ) ;
#31431=CARTESIAN_POINT ( 'NONE',  ( 13.44051670066911441, -5.407089921784865361, -9.571874999385554972 ) ) ;
#31437=CARTESIAN_POINT ( 'NONE',  ( 16.56230152254410726, 6.928203230275506996, -3.599999998771000520 ) ) ;
#31444=CARTESIAN_POINT ( 'NONE',  ( 16.56230152254411081, 6.928203230275514990, -9.112500000000034461 ) ) ;
#31449=VERTEX_POINT ( 'NONE', #9995 ) ;
#31459=CARTESIAN_POINT ( 'NONE',  ( 16.56230152254410370, -7.209453229046475009, -4.078124999385484450 ) ) ;
#31465=CARTESIAN_POINT ( 'NONE',  ( 22.56230152254410015, 7.347880794884117764E-16, -2.812499998771006204 ) ) ;
#31472=CARTESIAN_POINT ( 'NONE',  ( 22.56230152254411792, 7.347880794884125653E-16, -2.475000000000060485 ) ) ;
#31474=CARTESIAN_POINT ( 'NONE',  ( 22.80587116629410716, -3.604726614523235284, -2.203124999385539962 ) ) ;
#31476=ORIENTED_EDGE ( 'NONE', *, *, #10112, .T. ) ;
#31492=CARTESIAN_POINT ( 'NONE',  ( 22.80587116629411071, 3.604726614523243278, -9.384374999385521221 ) ) ;
#31514=CARTESIAN_POINT ( 'NONE',  ( 22.56230152254412502, 7.347880794884125653E-16, -3.375000000000044409 ) ) ;
#31521=DIRECTION ( 'NONE',  ( 0.000000000000000000, 0.000000000000000000, 1.000000000000000000 ) ) ;
#31533=CARTESIAN_POINT ( 'NONE',  ( 16.56230152254411436, 7.209453229046482114, -1.209374999385475657 ) ) ;
#31559=ORIENTED_EDGE ( 'NONE', *, *, #19562, .F. ) ;
#31562=EDGE_CURVE ( 'NONE', #2980, #26922, #7641, .T. ) ;
#31564=CARTESIAN_POINT ( 'NONE',  ( 10.56230152254612520, 3.464101615138916568, -9.824999998771035692 ) ) ;
#31568=CARTESIAN_POINT ( 'NONE',  ( 10.31873187879411091, 3.604726614523236616, -5.578124999385555505 ) ) ;
#31569=CARTESIAN_POINT ( 'NONE',  ( 16.56230152254410726, 0.000000000000000000, -10.00000000000000000 ) ) ;
#31582=CARTESIAN_POINT ( 'NONE',  ( 22.80587116629410360, 7.646167579472015790E-16, -1.715624999385545468 ) ) ;
#31612=CARTESIAN_POINT ( 'NONE',  ( 13.44051670066910731, 5.407089921784862696, -7.921874999385513760 ) ) ;
#31618=CYLINDRICAL_SURFACE ( 'NONE', #34340, 5.999999999999998224 ) ;
#31630=VERTEX_POINT ( 'NONE', #33492 ) ;
#31642=CARTESIAN_POINT ( 'NONE',  ( 16.56230152254411081, 7.209453229046475009, -3.403124999385538807 ) ) ;
#31649=CARTESIAN_POINT ( 'NONE',  ( 22.56230152254409660, 3.464101615137755275, -2.774999998771003007 ) ) ;
#31675=CARTESIAN_POINT ( 'NONE',  ( 22.80587116629412137, 7.646167579472024665E-16, -9.421874999385515537 ) ) ;
#31679=CARTESIAN_POINT ( 'NONE',  ( 13.44051670066911441, -5.407089921784865361, -4.621874999385545024 ) ) ;
#31700=CARTESIAN_POINT ( 'NONE',  ( 10.56230152254410726, 3.464101615137757051, -4.987500000000046008 ) ) ;
#31703=CARTESIAN_POINT ( 'NONE',  ( 22.56230152254410370, 0.000000000000000000, -10.00000000000000000 ) ) ;
#31719=CARTESIAN_POINT ( 'NONE',  ( 22.80587116629411426, 3.604726614523243278, -2.184374999385525040 ) ) ;
#31724=ORIENTED_EDGE ( 'NONE', *, *, #6389, .T. ) ;
#31753=CARTESIAN_POINT ( 'NONE',  ( 16.56230152254411081, 7.209453229046475009, -8.803124999385520510 ) ) ;
#31762=VERTEX_POINT ( 'NONE', #2020 ) ;
#31765=CARTESIAN_POINT ( 'NONE',  ( 10.31873187879411091, 0.000000000000000000, -4.640624999385528859 ) ) ;
#31769=ORIENTED_EDGE ( 'NONE', *, *, #32048, .F. ) ;
#31778=CARTESIAN_POINT ( 'NONE',  ( 10.56230152254410548, 0.000000000000000000, -9.000000000000035527 ) ) ;
#31781=CARTESIAN_POINT ( 'NONE',  ( 10.31873187879411091, 0.000000000000000000, -9.140624999385559946 ) ) ;
#31782=AXIS2_PLACEMENT_3D ( 'NONE', #9105, #17645, #14793 ) ;
#31789=CARTESIAN_POINT ( 'NONE',  ( 22.56230152254410015, 7.347880794884117764E-16, -8.212499998771022547 ) ) ;
#31793=CARTESIAN_POINT ( 'NONE',  ( 16.56230152254411436, 7.209453229046482114, -7.959374999385476102 ) ) ;
#31801=ORIENTED_EDGE ( 'NONE', *, *, #6126, .T. ) ;
#31811=AXIS2_PLACEMENT_3D ( 'NONE', #32414, #9115, #35065 ) ;
#31814=ORIENTED_EDGE ( 'NONE', *, *, #26302, .F. ) ;
#31825=CARTESIAN_POINT ( 'NONE',  ( 13.44051670066911441, -5.407089921784859143, -2.315624999385534899 ) ) ;
#31831=CARTESIAN_POINT ( 'NONE',  ( 22.56230152254410370, 7.347880794884117764E-16, -4.162499998770996967 ) ) ;
#31857=VERTEX_POINT ( 'NONE', #8097 ) ;
#31860=CARTESIAN_POINT ( 'NONE',  ( 10.31873187879410736, -3.604726614523244610, -8.709374999385511629 ) ) ;
#31864=CARTESIAN_POINT ( 'NONE',  ( 13.44051670066910908, 5.407089921784862696, -4.771874999385556038 ) ) ;
#31874=EDGE_CURVE ( 'NONE', #31762, #11777, #23348, .T. ) ;
#31885=CARTESIAN_POINT ( 'NONE',  ( 19.56230152254412502, -5.196152422706635576, -3.900000000000070077 ) ) ;
#31888=CARTESIAN_POINT ( 'NONE',  ( 10.56230152254410726, 0.000000000000000000, -0.9000000000000396572 ) ) ;
#31905=CARTESIAN_POINT ( 'NONE',  ( 19.68408634441911076, 5.407089921784862696, -1.246874999385527705 ) ) ;
#31914=DIRECTION ( 'NONE',  ( 0.000000000000000000, 0.000000000000000000, 1.000000000000000000 ) ) ;
#31917=EDGE_CURVE ( 'NONE', #27522, #13344, #8459, .T. ) ;
#31926=CARTESIAN_POINT ( 'NONE',  ( 10.56230152254410726, 0.000000000000000000, -5.400000000000043876 ) ) ;
#31930=CARTESIAN_POINT ( 'NONE',  ( 13.56230152254410548, 5.196152422706636465, -9.975000000000012079 ) ) ;
#31936=LINE ( 'NONE', #5968, #9084 ) ;
#31937=CARTESIAN_POINT ( 'NONE',  ( 13.44051670066911264, 5.407089921784856479, -8.315624999385541116 ) ) ;
#31946=VERTEX_POINT ( 'NONE', #5975 ) ;
#31951=CARTESIAN_POINT ( 'NONE',  ( 10.31873187879411269, 3.604726614523236616, -3.778124999385508609 ) ) ;
#31959=PLANE ( 'NONE',  #16423 ) ;
#31981=CARTESIAN_POINT ( 'NONE',  ( 13.56230152254411614, -5.196152422706632912, -9.712499998771024323 ) ) ;
#31986=CARTESIAN_POINT ( 'NONE',  ( 19.68408634441911076, 5.407089921784862696, -8.446874999385538985 ) ) ;
#32012=CARTESIAN_POINT ( 'NONE',  ( 22.80587116629410716, 3.604726614523238837, -5.278124999385515714 ) ) ;
#32017=CARTESIAN_POINT ( 'NONE',  ( 16.56230152254411081, 6.928203230275506996, -4.499999998770991105 ) ) ;
#32030=ORIENTED_EDGE ( 'NONE', *, *, #32495, .T. ) ;
#32045=CARTESIAN_POINT ( 'NONE',  ( 13.44051670066911441, -5.407089921784865361, -9.121874999385520155 ) ) ;
#32048=EDGE_CURVE ( 'NONE', #35189, #31630, #7505, .T. ) ;
#32049=CARTESIAN_POINT ( 'NONE',  ( 10.56230152254410726, 0.000000000000000000, -1.350000000000045608 ) ) ;
#32051=CARTESIAN_POINT ( 'NONE',  ( 10.31873187879411091, -3.604726614523244610, -2.859374999385534633 ) ) ;
#32052=ORIENTED_EDGE ( 'NONE', *, *, #21473, .T. ) ;
#32071=CARTESIAN_POINT ( 'NONE',  ( 19.56230152254412502, 5.196152422706637353, -4.650000000000070521 ) ) ;
#32080=DIRECTION ( 'NONE',  ( 0.000000000000000000, 0.000000000000000000, 1.000000000000000000 ) ) ;
#32090=CARTESIAN_POINT ( 'NONE',  ( 16.56230152254411436, 7.209453229046482114, -2.559374999385494842 ) ) ;
#32095=CIRCLE ( 'NONE', #25440, 1.500000000000001332 ) ;
#32098=CARTESIAN_POINT ( 'NONE',  ( 10.56230152254339494, 3.464101615137343160, -0.9375000000000115463 ) ) ;
#32118=CIRCLE ( 'NONE', #28491, 5.999999999999998224 ) ;
#32122=CARTESIAN_POINT ( 'NONE',  ( 19.68408634441910721, 5.407089921784857367, -7.940624999385553551 ) ) ;
#32134=CARTESIAN_POINT ( 'NONE',  ( 13.44051670066911086, 5.407089921784856479, -5.165624999385554084 ) ) ;
#32146=CARTESIAN_POINT ( 'NONE',  ( 22.56230152254410370, 7.347880794884117764E-16, -5.512499998771014376 ) ) ;
#32148=VECTOR ( 'NONE', #13001, 1000.000000000000000 ) ;
#32151=FACE_OUTER_BOUND ( 'NONE', #1756, .T. ) ;
#32161=EDGE_CURVE ( 'NONE', #1340, #34717, #36091, .T. ) ;
#32169=CARTESIAN_POINT ( 'NONE',  ( 10.31873187879410736, 3.604726614523240613, -8.334374999385541827 ) ) ;
#32172=CARTESIAN_POINT ( 'NONE',  ( 16.56230152254411081, -7.209453229046475009, -1.828124999385505989 ) ) ;
#32182=AXIS2_PLACEMENT_3D ( 'NONE', #31569, #5591, #13962 ) ;
#32204=CARTESIAN_POINT ( 'NONE',  ( 10.31873187879411269, -3.604726614523240613, -5.503124999385529570 ) ) ;
#32209=CARTESIAN_POINT ( 'NONE',  ( 10.56230152254411259, 3.464101615137752166, -5.324999998771021481 ) ) ;
#32239=CARTESIAN_POINT ( 'NONE',  ( 22.80587116629411781, -3.604726614523238837, -2.709374999385514737 ) ) ;
#32249=ORIENTED_EDGE ( 'NONE', *, *, #23035, .F. ) ;
#32256=CARTESIAN_POINT ( 'NONE',  ( 19.56230152254412502, 5.196152422706637353, -5.550000000000054889 ) ) ;
#32274=CARTESIAN_POINT ( 'NONE',  ( 10.31873187879410736, -3.604726614523244610, -1.959374999385511407 ) ) ;
#32280=VECTOR ( 'NONE', #5882, 1000.000000000000000 ) ;
#32302=VERTEX_POINT ( 'NONE', #27570 ) ;
#32310=CARTESIAN_POINT ( 'NONE',  ( 10.31873187879411269, 3.604726614523236616, -9.178124999385520510 ) ) ;
#32313=CARTESIAN_POINT ( 'NONE',  ( 13.18934786828137362, 5.048416078761468917, -9.999999999999994671 ) ) ;
#32321=CARTESIAN_POINT ( 'NONE',  ( 13.56230152254411436, -5.196152422706632912, -3.412499998771051146 ) ) ;
#32322=CARTESIAN_POINT ( 'NONE',  ( 19.68408634441910721, -5.407089921784855591, -4.040624999385538985 ) ) ;
#32330=ORIENTED_EDGE ( 'NONE', *, *, #26378, .F. ) ;
#32337=CYLINDRICAL_SURFACE ( 'NONE', #4872, 5.999999999999998224 ) ;
#32359=CARTESIAN_POINT ( 'NONE',  ( 10.31873187879411091, 0.000000000000000000, -2.390624999385526639 ) ) ;
#32369=CARTESIAN_POINT ( 'NONE',  ( 19.56230152254412502, -5.196152422706635576, -6.600000000000050271 ) ) ;
#32380=ORIENTED_EDGE ( 'NONE', *, *, #10179, .F. ) ;
#32387=EDGE_CURVE ( 'NONE', #11777, #10703, #856, .T. ) ;
#32389=CARTESIAN_POINT ( 'NONE',  ( 13.44051670066911619, -5.407089921784859143, -4.565624999385536675 ) ) ;
#32394=CARTESIAN_POINT ( 'NONE',  ( 10.56230152254410903, 3.464101615137752166, -7.124999998771004428 ) ) ;
#32395=EDGE_CURVE ( 'NONE', #20367, #2209, #7856, .T. ) ;
#32400=CARTESIAN_POINT ( 'NONE',  ( 13.44051670066910908, 5.407089921784862696, -4.321874999385522109 ) ) ;
#32402=CARTESIAN_POINT ( 'NONE',  ( 16.56230152254411081, 6.928203230275506996, -7.199999998770998388 ) ) ;
#32414=CARTESIAN_POINT ( 'NONE',  ( 16.56230152254410726, 0.000000000000000000, -10.00000000000000000 ) ) ;
#32428=CARTESIAN_POINT ( 'NONE',  ( 19.68408634441911076, 5.407089921784862696, -3.496874999385557459 ) ) ;
#32446=CARTESIAN_POINT ( 'NONE',  ( 13.56230152254411792, -5.196152422706638241, -6.675000000000069988 ) ) ;
#32454=CARTESIAN_POINT ( 'NONE',  ( 17.75238460531252471, -6.096976528379499882, -10.00000000000000000 ) ) ;
#32463=CARTESIAN_POINT ( 'NONE',  ( 16.56230152254411436, -7.209453229046482114, -2.784374999385508698 ) ) ;
#32481=CARTESIAN_POINT ( 'NONE',  ( 19.56230152254412147, 5.196152422706637353, -7.350000000000022737 ) ) ;
#32484=CARTESIAN_POINT ( 'NONE',  ( 22.56230152254412147, 7.347880794884125653E-16, -9.225000000000010303 ) ) ;
#32487=FACE_OUTER_BOUND ( 'NONE', #28278, .T. ) ;
#32490=VECTOR ( 'NONE', #28893, 1000.000000000000000 ) ;
#32491=DIRECTION ( 'NONE',  ( 0.000000000000000000, 0.000000000000000000, 1.000000000000000000 ) ) ;
#32492=CARTESIAN_POINT ( 'NONE',  ( 22.80587116629410360, -3.604726614523235284, -8.953124999385540406 ) ) ;
#32495=EDGE_CURVE ( 'NONE', #29192, #25759, #18879, .T. ) ;
#32505=CARTESIAN_POINT ( 'NONE',  ( 10.31873187879411091, -3.604726614523240613, -3.253124999385518912 ) ) ;
#32514=CARTESIAN_POINT ( 'NONE',  ( 16.56230152254411436, -6.928203230275506996, -2.024999998770999454 ) ) ;
#32520=FACE_OUTER_BOUND ( 'NONE', #10289, .T. ) ;
#32533=DIRECTION ( 'NONE',  ( 0.000000000000000000, 0.000000000000000000, 1.000000000000000000 ) ) ;
#32539=CARTESIAN_POINT ( 'NONE',  ( 10.56230152254410903, 7.347880794884117764E-16, -10.00000000000000000 ) ) ;
#32543=CARTESIAN_POINT ( 'NONE',  ( 10.31873187879411091, 3.604726614523236616, -1.528124999385498173 ) ) ;
#32575=CARTESIAN_POINT ( 'NONE',  ( 13.44051670066911797, -5.407089921784859143, -6.365624999385560479 ) ) ;
#32581=CARTESIAN_POINT ( 'NONE',  ( 19.56230152254410726, 5.196152422706631135, -6.337499998771006560 ) ) ;
#32588=CARTESIAN_POINT ( 'NONE',  ( 22.80587116629411781, -3.604726614523238837, -3.609374999385538185 ) ) ;
#32597=ORIENTED_EDGE ( 'NONE', *, *, #10840, .T. ) ;
#32605=LINE ( 'NONE', #386, #24253 ) ;
#32618=CARTESIAN_POINT ( 'NONE',  ( 13.44051670066910908, 5.407089921784862696, -6.571874999385523886 ) ) ;
#32635=EDGE_CURVE ( 'NONE', #11078, #3622, #19067, .T. ) ;
#32637=CARTESIAN_POINT ( 'NONE',  ( 16.56230152254411436, -6.928203230275514990, -7.087500000000036771 ) ) ;
#32654=CARTESIAN_POINT ( 'NONE',  ( 13.44051670066910908, 5.407089921784862696, -4.771874999385556038 ) ) ;
#32665=CARTESIAN_POINT ( 'NONE',  ( 22.80587116629411071, 3.604726614523238837, -1.228124999385522331 ) ) ;
#32672=CARTESIAN_POINT ( 'NONE',  ( 22.56230152254411792, 7.347880794884125653E-16, -7.425000000000042455 ) ) ;
#32679=CARTESIAN_POINT ( 'NONE',  ( 19.56230152254412147, -5.196152422706635576, -0.3000000000000779821 ) ) ;
#32696=CARTESIAN_POINT ( 'NONE',  ( 10.31873187879411091, 3.604726614523236616, -6.478124999385515004 ) ) ;
#32705=CARTESIAN_POINT ( 'NONE',  ( 19.56230152254412502, -5.196152422706635576, -3.900000000000070077 ) ) ;
#32712=CARTESIAN_POINT ( 'NONE',  ( 13.56230152254411614, -5.196152422706638241, -5.775000000000085620 ) ) ;
#32727=VERTEX_POINT ( 'NONE', #16215 ) ;
#32734=CARTESIAN_POINT ( 'NONE',  ( 13.44051670066911086, 5.407089921784856479, -5.165624999385554084 ) ) ;
#32741=CARTESIAN_POINT ( 'NONE',  ( 19.56230152254412502, 5.196152422706637353, -5.100000000000049383 ) ) ;
#32747=CARTESIAN_POINT ( 'NONE',  ( 16.56230152254411081, -6.928203230275514990, -6.637500000000041034 ) ) ;
#32755=AXIS2_PLACEMENT_3D ( 'NONE', #23878, #18382, #29932 ) ;
#32766=CARTESIAN_POINT ( 'NONE',  ( 22.80587116629410360, 3.604726614523238837, -4.828124999385519978 ) ) ;
#32773=CARTESIAN_POINT ( 'NONE',  ( 22.56230152254410370, 7.347880794884117764E-16, -5.512499998771014376 ) ) ;
#32777=CARTESIAN_POINT ( 'NONE',  ( 22.80587116629412137, 7.646167579472024665E-16, -3.571874999385521221 ) ) ;
#32778=CARTESIAN_POINT ( 'NONE',  ( 16.56230152254411081, 6.928203230275506996, -3.149999998770972365 ) ) ;
#32794=CARTESIAN_POINT ( 'NONE',  ( 13.44051670066911086, 5.407089921784856479, -0.2156249993855441360 ) ) ;
#32806=CARTESIAN_POINT ( 'NONE',  ( 16.56230152254411436, -7.209453229046482114, -6.384374999385507010 ) ) ;
#32823=CARTESIAN_POINT ( 'NONE',  ( 16.56230152254411436, 6.928203230275514990, -7.762500000000014388 ) ) ;
#32831=CARTESIAN_POINT ( 'NONE',  ( 16.56230152254410726, 0.000000000000000000, 10.00000000000000000 ) ) ;
#32833=CARTESIAN_POINT ( 'NONE',  ( 15.26155779561005232, -6.106572496351636126, -10.00000000000000000 ) ) ;
#32841=CARTESIAN_POINT ( 'NONE',  ( 22.80587116629411781, -3.604726614523238837, -3.609374999385538185 ) ) ;
#32862=CARTESIAN_POINT ( 'NONE',  ( 16.56230152254411792, 6.928203230275514990, -7.312500000000050626 ) ) ;
#32875=CARTESIAN_POINT ( 'NONE',  ( 22.56230152254392252, -3.464101615137877843, -2.512500000000024158 ) ) ;
#32886=CARTESIAN_POINT ( 'NONE',  ( 16.56230152254411081, 7.209453229046475009, -5.653124999385517491 ) ) ;
#32913=ORIENTED_EDGE ( 'NONE', *, *, #33185, .F. ) ;
#32922=CARTESIAN_POINT ( 'NONE',  ( 16.56230152254411436, -7.209453229046475009, -4.978124999385539873 ) ) ;
#32929=CARTESIAN_POINT ( 'NONE',  ( 10.56230152254516952, -3.464101615138373003, -8.512500000000034817 ) ) ;
#32932=CARTESIAN_POINT ( 'NONE',  ( 10.56230152254395094, 3.464101615137665124, -1.837500000000042100 ) ) ;
#32942=VERTEX_POINT ( 'NONE', #3341 ) ;
#32954=CARTESIAN_POINT ( 'NONE',  ( 10.31873187879410736, 3.604726614523236616, -8.728124999385526550 ) ) ;
#32961=CARTESIAN_POINT ( 'NONE',  ( 19.56230152254411081, -5.196152422706629359, -6.487499998771045995 ) ) ;
#32964=CARTESIAN_POINT ( 'NONE',  ( 16.56230152254411436, 7.209453229046482114, -3.009374999385522553 ) ) ;
#32966=CARTESIAN_POINT ( 'NONE',  ( 10.56230152254411081, 0.000000000000000000, -2.587499998771031429 ) ) ;
#32978=FACE_OUTER_BOUND ( 'NONE', #6418, .T. ) ;
#32982=CARTESIAN_POINT ( 'NONE',  ( 10.31873187879411091, -3.604726614523240613, -0.5531249993855127389 ) ) ;
#32993=CARTESIAN_POINT ( 'NONE',  ( 10.56230152254500965, 3.464101615138273971, -8.024999998771040310 ) ) ;
#32995=CARTESIAN_POINT ( 'NONE',  ( 19.68408634441911431, -5.407089921784861808, -6.346874999385549110 ) ) ;
#33003=EDGE_CURVE ( 'NONE', #7808, #28808, #26996, .T. ) ;
#33006=CARTESIAN_POINT ( 'NONE',  ( 22.56230152254410370, 7.347880794884117764E-16, -8.662499998771028942 ) ) ;
#33016=CARTESIAN_POINT ( 'NONE',  ( 22.56230152254411792, 7.347880794884125653E-16, -7.875000000000048850 ) ) ;
#33021=CARTESIAN_POINT ( 'NONE',  ( 16.56230152254410726, -6.928203230275506996, -6.074999998771025034 ) ) ;
#33026=CARTESIAN_POINT ( 'NONE',  ( 13.56230152254410548, 5.196152422706630247, -1.312499998771005094 ) ) ;
#33030=ORIENTED_EDGE ( 'NONE', *, *, #30732, .F. ) ;
#33035=CARTESIAN_POINT ( 'NONE',  ( 10.31873187879410736, -3.604726614523244610, -3.309374999385498395 ) ) ;
#33062=CARTESIAN_POINT ( 'NONE',  ( 16.56230152254411436, 6.928203230275514990, -0.1125000000000229705 ) ) ;
#33080=CARTESIAN_POINT ( 'NONE',  ( 16.56230152254411081, -7.209453229046475009, -6.328124999385527083 ) ) ;
#33087=VERTEX_POINT ( 'NONE', #21826 ) ;
#33094=CARTESIAN_POINT ( 'NONE',  ( 22.56230152254337185, -3.464101615138180268, -3.749999998771029297 ) ) ;
#33095=CARTESIAN_POINT ( 'NONE',  ( 22.56230152254410370, 7.347880794884117764E-16, -5.062499998771007981 ) ) ;
#33107=EDGE_LOOP ( 'NONE', ( #30106, #1363, #19715, #30359 ) ) ;
#33114=CARTESIAN_POINT ( 'NONE',  ( 13.44051670066911264, 5.407089921784856479, -3.815624999385564209 ) ) ;
#33122=CARTESIAN_POINT ( 'NONE',  ( 13.56230152254411436, -5.196152422706632912, -7.912499998771055587 ) ) ;
#33133=CARTESIAN_POINT ( 'NONE',  ( 19.56230152254410370, 5.196152422706631135, -4.087499998771032317 ) ) ;
#33134=EDGE_CURVE ( 'NONE', #28841, #18251, #4929, .T. ) ;
#33149=CARTESIAN_POINT ( 'NONE',  ( 22.80587116629411426, -3.604726614523235284, -8.053124999385516958 ) ) ;
#33154=CARTESIAN_POINT ( 'NONE',  ( 16.56230152254411081, 6.928203230275506996, -8.549999998770985599 ) ) ;
#33157=CARTESIAN_POINT ( 'NONE',  ( 13.44051670066911441, -5.407089921784865361, -4.621874999385545024 ) ) ;
#33162=CYLINDRICAL_SURFACE ( 'NONE', #25547, 5.999999999999998224 ) ;
#33175=CARTESIAN_POINT ( 'NONE',  ( 13.44051670066911086, 5.407089921784856479, -2.015624999385540406 ) ) ;
#33185=EDGE_CURVE ( 'NONE', #36053, #21699, #2315, .T. ) ;
#33187=CARTESIAN_POINT ( 'NONE',  ( 13.44051670066911441, -5.407089921784865361, -5.071874999385522997 ) ) ;
#33200=CARTESIAN_POINT ( 'NONE',  ( 10.56230152254411614, -3.464101615137757051, -0.7499999987710380678 ) ) ;
#33201=ORIENTED_EDGE ( 'NONE', *, *, #30770, .T. ) ;
#33208=CARTESIAN_POINT ( 'NONE',  ( 10.56230152254410726, 0.000000000000000000, -8.100000000000024514 ) ) ;
#33217=CARTESIAN_POINT ( 'NONE',  ( 19.17052166273705538, -5.587842338165578404, -10.00000000000000355 ) ) ;
#33224=CARTESIAN_POINT ( 'NONE',  ( 13.44051670066911086, 5.407089921784862696, -2.971874999385532234 ) ) ;
#33240=CARTESIAN_POINT ( 'NONE',  ( 16.56230152254410726, 0.000000000000000000, -10.00000000000000000 ) ) ;
#33266=CARTESIAN_POINT ( 'NONE',  ( 22.80587116629410716, -3.604726614523235284, -6.703124999385561722 ) ) ;
#33268=DIRECTION ( 'NONE',  ( 0.000000000000000000, 0.000000000000000000, 1.000000000000000000 ) ) ;
#33273=ORIENTED_EDGE ( 'NONE', *, *, #19562, .T. ) ;
#33276=CARTESIAN_POINT ( 'NONE',  ( 13.56230152254411792, -5.196152422706638241, -9.375000000000078160 ) ) ;
#33304=CARTESIAN_POINT ( 'NONE',  ( 19.68408634441910721, -5.407089921784855591, -4.490624999385572913 ) ) ;
#33311=CARTESIAN_POINT ( 'NONE',  ( 10.56230152254321020, -3.464101615137235690, -7.949999998771044574 ) ) ;
#33313=CARTESIAN_POINT ( 'NONE',  ( 13.44051670066911086, -5.407089921784865361, -0.5718749993855187785 ) ) ;
#33315=ORIENTED_EDGE ( 'NONE', *, *, #25845, .T. ) ;
#33335=CARTESIAN_POINT ( 'NONE',  ( 16.56230152254411081, 7.209453229046475009, -7.453124999385500438 ) ) ;
#33342=CARTESIAN_POINT ( 'NONE',  ( 16.56230152254410726, 6.928203230275506996, -8.999999998771013310 ) ) ;
#33346=CARTESIAN_POINT ( 'NONE',  ( 19.68408634441912142, -5.407089921784861808, -6.796874999385527083 ) ) ;
#33351=DIRECTION ( 'NONE',  ( 0.000000000000000000, 0.000000000000000000, 1.000000000000000000 ) ) ;
#33366=ORIENTED_EDGE ( 'NONE', *, *, #27555, .F. ) ;
#33371=CARTESIAN_POINT ( 'NONE',  ( 14.45804369857214589, -5.892651062571511389, -9.999999999999991118 ) ) ;
#33374=CARTESIAN_POINT ( 'NONE',  ( 16.56230152254411081, -7.209453229046482114, -6.834374999385501859 ) ) ;
#33387=CARTESIAN_POINT ( 'NONE',  ( 10.56230152254411081, 0.000000000000000000, -2.137499998771025034 ) ) ;
#33395=CARTESIAN_POINT ( 'NONE',  ( 19.56230152254412147, -5.196152422706635576, -9.750000000000063949 ) ) ;
#33410=CARTESIAN_POINT ( 'NONE',  ( 22.80587116629412847, 3.604726614523243278, -6.234374999385518201 ) ) ;
#33424=CARTESIAN_POINT ( 'NONE',  ( 10.56230152254495103, 3.464101615138235335, -1.724999998771002074 ) ) ;
#33430=CARTESIAN_POINT ( 'NONE',  ( 16.56230152254411436, -6.928203230275514990, -1.237499999999996270 ) ) ;
#33435=CARTESIAN_POINT ( 'NONE',  ( 22.56230152254542887, 3.464101615136989665, -8.624999998771029297 ) ) ;
#33436=CYLINDRICAL_SURFACE ( 'NONE', #14139, 5.999999999999998224 ) ;
#33446=CARTESIAN_POINT ( 'NONE',  ( 16.56230152254410726, -7.209453229046475009, -8.578124999385506655 ) ) ;
#33454=ORIENTED_EDGE ( 'NONE', *, *, #16324, .T. ) ;
#33455=VERTEX_POINT ( 'NONE', #11988 ) ;
#33458=CARTESIAN_POINT ( 'NONE',  ( 10.56230152254410548, 0.000000000000000000, -9.450000000000041922 ) ) ;
#33485=CARTESIAN_POINT ( 'NONE',  ( 16.56230152254410015, -7.209453229046475009, -4.078124999385484450 ) ) ;
#33489=CARTESIAN_POINT ( 'NONE',  ( 22.80587116629412137, 7.646167579472024665E-16, -9.421874999385515537 ) ) ;
#33491=CARTESIAN_POINT ( 'NONE',  ( 22.56230152254412147, 7.347880794884125653E-16, -8.325000000000027711 ) ) ;
#33492=CARTESIAN_POINT ( 'NONE',  ( 24.56230152254410726, 0.000000000000000000, 2.535898384862258492 ) ) ;
#33494=CARTESIAN_POINT ( 'NONE',  ( 16.56230152254411436, -7.209453229046482114, -0.5343749993854981506 ) ) ;
#33517=CARTESIAN_POINT ( 'NONE',  ( 10.31873187879410736, -3.604726614523240613, -8.203124999385504879 ) ) ;
#33518=( BOUNDED_CURVE ( )  B_SPLINE_CURVE ( 2, ( #27531, #8000, #31125, #4590, #13128, #2303, #24682 ),
 .UNSPECIFIED., .F., .F. ) 
 B_SPLINE_CURVE_WITH_KNOTS ( ( 3, 2, 2, 3 ),
 ( 0.3478260869565210633, 0.3550724637681153539, 0.3623188405797096445, 0.3695652173913038796 ),
 .UNSPECIFIED. ) 
 CURVE ( )  GEOMETRIC_REPRESENTATION_ITEM ( )  RATIONAL_B_SPLINE_CURVE ( ( 1.000000000000012212, 0.8660254037844263841, 1.000000000000000000, 0.8660254037844387076, 1.000000000000000000, 0.8660254037844469233, 0.9999999999999917843 ) ) 
 REPRESENTATION_ITEM ( '' )  );
#33523=CARTESIAN_POINT ( 'NONE',  ( 13.56230152254411614, -5.196152422706632912, -9.262499998771044574 ) ) ;
#33528=CARTESIAN_POINT ( 'NONE',  ( 22.80587116629411781, 3.604726614523243278, -5.784374999385522464 ) ) ;
#33532=CARTESIAN_POINT ( 'NONE',  ( 19.56230152254412502, 5.196152422706637353, -6.000000000000060396 ) ) ;
#33536=CARTESIAN_POINT ( 'NONE',  ( 10.56230152254307519, 3.464101615137159751, -4.537500000000036948 ) ) ;
#33549=ORIENTED_EDGE ( 'NONE', *, *, #13312, .T. ) ;
#33559=CARTESIAN_POINT ( 'NONE',  ( 11.73492611592313573, -4.045813723653100880, -9.999999999999998224 ) ) ;
#33562=CARTESIAN_POINT ( 'NONE',  ( 19.68408634441911076, 5.407089921784862696, -7.546874999385555505 ) ) ;
#33566=CARTESIAN_POINT ( 'NONE',  ( 22.80587116629410716, 3.604726614523238837, -0.3281249993855308023 ) ) ;
#33570=( NAMED_UNIT ( * ) PLANE_ANGLE_UNIT ( ) SI_UNIT ( $, .RADIAN. ) );
#33571=CARTESIAN_POINT ( 'NONE',  ( 22.56230152254391896, -3.464101615137866741, -2.849999998770999632 ) ) ;
#33574=CARTESIAN_POINT ( 'NONE',  ( 19.56230152254411792, -5.196152422706629359, -1.537499998771035825 ) ) ;
#33579=CYLINDRICAL_SURFACE ( 'NONE', #35092, 1.500000000000001332 ) ;
#33581=CARTESIAN_POINT ( 'NONE',  ( 13.56230152254410548, 5.196152422706636465, -9.525000000000034106 ) ) ;
#33597=CARTESIAN_POINT ( 'NONE',  ( 13.44051670066911441, -5.407089921784865361, -6.871874999385546801 ) ) ;
#33613=CARTESIAN_POINT ( 'NONE',  ( 19.56230152254410370, 5.196152422706631135, -1.837499998771002785 ) ) ;
#33620=CARTESIAN_POINT ( 'NONE',  ( 19.56230152254412147, 5.196152422706637353, -1.500000000000029088 ) ) ;
#33638=CARTESIAN_POINT ( 'NONE',  ( 16.56230152254411081, -7.209453229046475009, -8.128124999385510918 ) ) ;
#33673=CARTESIAN_POINT ( 'NONE',  ( 13.44051670066911619, -5.407089921784859143, -7.265624999385544847 ) ) ;
#33682=CARTESIAN_POINT ( 'NONE',  ( 19.68408634441911431, -5.407089921784861808, -0.4968749993855270386 ) ) ;
#33700=EDGE_CURVE ( 'NONE', #26085, #16407, #34305, .T. ) ;
#33704=CARTESIAN_POINT ( 'NONE',  ( 13.44051670066911086, 5.407089921784856479, -7.415624999385555860 ) ) ;
#33709=CARTESIAN_POINT ( 'NONE',  ( 22.56230152254411436, -3.464101615137751278, -9.149999998771001231 ) ) ;
#33712=CARTESIAN_POINT ( 'NONE',  ( 19.68408634441910721, 5.407089921784862696, -9.796874999385529748 ) ) ;
#33713=CARTESIAN_POINT ( 'NONE',  ( 10.31873187879410736, 0.000000000000000000, -7.396874999385516958 ) ) ;
#33721=CARTESIAN_POINT ( 'NONE',  ( 10.56230152254349086, 3.464101615137404888, -3.187499999999991562 ) ) ;
#33722=DIRECTION ( 'NONE',  ( 1.000000000000000000, 0.000000000000000000, 0.000000000000000000 ) ) ;
#33743=( BOUNDED_SURFACE ( )  B_SPLINE_SURFACE ( 1, 2, ( 
 ( #6268, #24276, #32794, #29954, #3420, #15745, #29574, #27113, #12704, #9861, #18602, #32982, #11952, #9117, #17845, #14988, #26538, #568, #12135, #19860, #2029, #27485, #28365, #13606, #19678, #11124, #37263, #15937, #5246, #33875, #31037, #28182, #5059, #25156, #21624, #25710, #8104, #16823, #22323, #16641, #19491, #24460, #31582, #28544, #7219, #34429, #8287, #36009, #36711, #31217, #33175, #2213, #13795, #7917, #10048, #25342, #18791, #13975, #36891, #22511, #10937, #10750, #37078, #5422, #34058, #31403, #2400, #25525, #11310, #22701, #34245, #17003, #30332, #4356, #2586, #14156, #22878, #8466, #20036, #5605, #27296, #1327, #12896, #32505, #12233, #11858, #23061, #23427, #11492, #20409, #17376, #108, #35159, #8650, #14341, #14709, #6174, #31951, #28730, #35344, #5796, #9209, #20593, #17746, #32322, #9398, #6363, #5983, #20973, #292, #34979, #23804, #17563, #34607, #26632, #34793, #3141, #20219, #3326, #29098, #31765, #20780, #17190, #12045, #29287, #28919, #25895, #14897, #2953, #26445, #661, #478, #23615, #9021, #32134, #17934, #14523, #29478, #26257, #3515, #26079, #15082, #2768, #37443, #11672, #23247, #8837, #32886, #9584, #21898, #3890, #12612, #6936, #16028, #13175, #27016, #27199, #9953, #4079, #21347, #12425, #1041, #30428, #36099, #18313, #33080, #9769, #18124, #24730, #32696, #24548, #21534, #7123, #21715, #36280, #33266, #18506, #10328, #1225, #12797, #1606, #30045, #854, #27577, #24178, #15651, #35539, #30236, #24366, #21158, #10142, #6551, #1415, #18695, #6738, #3702, #29667, #15462, #4448, #15271, #26824, #23994, #35910, #29853, #4262, #35723, #15837, #27385, #12993, #7305, #18877, #4634, #22458, #33638, #25659, #28132, #7864, #30988, #27763, #16769, #1793, #33827, #19438, #28315, #11260, #33446, #5006, #16587, #7489, #22274, #25101, #16213, #19065, #7677, #34005, #27946, #36659, #10697, #30617, #37213, #34193, #13360, #2540, #13925, #24915, #19257, #36842, #36467, #2161, #13744, #1976, #10508, #25290, #22088, #19626, #10885, #8050, #31172, #4819, #5194, #11072, #30796, #25475, #2353, #16400, #16954, #37026, #22647, #8239, #13548, #19814 ),
 ( #28497, #31348, #14107, #5375, #28679, #29048, #17143, #26029, #23011, #5746, #3279, #14293, #19989, #20362, #22831, #6317, #616, #17889, #17514, #2717, #3092, #25846, #57, #34561, #17326, #14852, #37394, #31533, #31905, #11811, #11624, #34379, #3470, #11444, #26401, #26211, #23381, #434, #15039, #11999, #23199, #26587, #5934, #14660, #29434, #34747, #8600, #32274, #2904, #8790, #20171, #8975, #247, #31719, #23570, #8420, #17699, #34930, #28869, #5558, #14476, #20546, #20731, #32090, #6121, #29239, #35115, #9164, #996, #32463, #9910, #15421, #21494, #23949, #33224, #20924, #1184, #12379, #4405, #6886, #24139, #9733, #6506, #33035, #18081, #12572, #35681, #7084, #27536, #12186, #21305, #32841, #23758, #18462, #3844, #29622, #35297, #35491, #12758, #6695, #26967, #30004, #9353, #15988, #12948, #3657, #18838, #30193, #15228, #9541, #15605, #26778, #4033, #27161, #18266, #808, #24326, #21115, #35868, #18652, #4219, #15797, #32654, #27347, #1378, #29810, #24509, #36057, #10101, #7263, #21670, #30384, #5148, #21857, #30579, #2121, #36613, #30943, #36241, #25249, #28275, #22417, #33784, #13698, #1561, #16172, #36799, #22604, #10843, #33964, #7822, #22233, #8006, #7448, #19579, #27903, #19399, #27722, #36986, #31131, #13133, #33410, #25434, #4961, #1934, #4595, #16915, #36425, #7636, #13502, #11029, #8196, #22046, #16543, #28089, #10654, #16355, #19022, #33597, #34149, #16729, #13318, #1752, #2311, #24876, #13885, #19772, #31309, #10468, #5337, #19213, #4781, #25060, #24688, #30759, #10283, #34891, #14434, #37350, #11584, #23159, #11774, #29007, #37173, #20128, #28639, #25801, #26172, #34701, #8380, #5704, #2492, #29196, #14252, #11402, #11214, #2677, #17284, #34335, #14067, #28456, #28825, #8748, #3051, #22786, #20319, #8931, #31860, #5894, #6076, #14621, #208, #17472, #5515, #23340, #22973, #18, #20508, #32045, #17661, #3238, #34521, #25616, #8561, #19951, #31492, #31675, #17100, #2860, #25988, #25552, #2241, #25367, #2057, #10962, #10407, #33712, #5087, #13635, #37104, #36914, #33899, #28390, #25184, #10776, #19517, #36737, #27838, #22536, #31244, #2611 ) ),
 .UNSPECIFIED., .F., .F., .F. ) 
 B_SPLINE_SURFACE_WITH_KNOTS ( ( 2, 2 ),
 ( 3, 2, 2, 2, 2, 2, 2, 2, 2, 2, 2, 2, 2, 2, 2, 2, 2, 2, 2, 2, 2, 2, 2, 2, 2, 2, 2, 2, 2, 2, 2, 2, 2, 2, 2, 2, 2, 2, 2, 2, 2, 2, 2, 2, 2, 2, 2, 2, 2, 2, 2, 2, 2, 2, 2, 2, 2, 2, 2, 2, 2, 2, 2, 2, 2, 2, 2, 2, 2, 2, 2, 2, 2, 2, 2, 2, 2, 2, 2, 2, 2, 2, 2, 2, 2, 2, 2, 2, 2, 2, 2, 2, 2, 2, 2, 2, 2, 2, 2, 2, 2, 2, 2, 2, 2, 2, 2, 2, 2, 2, 2, 2, 2, 2, 2, 2, 2, 2, 2, 2, 2, 2, 2, 2, 2, 2, 2, 2, 2, 2, 2, 2, 2, 2, 2, 3 ),
 ( 0.000000000000000000, 1.000000000000000000 ),
 ( 0.000000000000000000, 0.007246376811594202987, 0.01449275362318840597, 0.02173913043478260809, 0.02898550724637681195, 0.03623188405797101580, 0.04347826086956521618, 0.05072463768115942351, 0.05797101449275362389, 0.06521739130434782428, 0.07246376811594203160, 0.07971014492753622505, 0.08695652173913043237, 0.09420289855072463969, 0.1014492753623188470, 0.1086956521739130405, 0.1159420289855072478, 0.1231884057971014551, 0.1304347826086956486, 0.1376811594202898559, 0.1449275362318840632, 0.1521739130434782705, 0.1594202898550724501, 0.1666666666666666574, 0.1739130434782608647, 0.1811594202898550721, 0.1884057971014492794, 0.1956521739130434867, 0.2028985507246376940, 0.2101449275362318736, 0.2173913043478260809, 0.2246376811594202882, 0.2318840579710144956, 0.2391304347826087029, 0.2463768115942029102, 0.2536231884057971175, 0.2608695652173912971, 0.2681159420289855322, 0.2753623188405797118, 0.2826086956521738913, 0.2898550724637681264, 0.2971014492753623060, 0.3043478260869565410, 0.3115942028985507206, 0.3188405797101449002, 0.3260869565217391353, 0.3333333333333333148, 0.3405797101449275499, 0.3478260869565217295, 0.3550724637681159646, 0.3623188405797101441, 0.3695652173913043237, 0.3768115942028985588, 0.3840579710144927383, 0.3913043478260869734, 0.3985507246376811530, 0.4057971014492753881, 0.4130434782608695676, 0.4202898550724637472, 0.4275362318840579823, 0.4347826086956521618, 0.4420289855072463969, 0.4492753623188405765, 0.4565217391304347561, 0.4637681159420289911, 0.4710144927536231707, 0.4782608695652174058, 0.4855072463768115854, 0.4927536231884058204, 0.5000000000000000000, 0.5072463768115942351, 0.5144927536231883591, 0.5217391304347825942, 0.5289855072463768293, 0.5362318840579710644, 0.5434782608695651884, 0.5507246376811594235, 0.5579710144927536586, 0.5652173913043477826, 0.5724637681159420177, 0.5797101449275362528, 0.5869565217391304879, 0.5942028985507246119, 0.6014492753623188470, 0.6086956521739130821, 0.6159420289855072062, 0.6231884057971014412, 0.6304347826086956763, 0.6376811594202898004, 0.6449275362318840354, 0.6521739130434782705, 0.6594202898550725056, 0.6666666666666666297, 0.6739130434782608647, 0.6811594202898550998, 0.6884057971014492239, 0.6956521739130434590, 0.7028985507246376940, 0.7101449275362319291, 0.7173913043478260532, 0.7246376811594202882, 0.7318840579710145233, 0.7391304347826086474, 0.7463768115942028825, 0.7536231884057971175, 0.7608695652173913526, 0.7681159420289854767, 0.7753623188405797118, 0.7826086956521739468, 0.7898550724637680709, 0.7971014492753623060, 0.8043478260869565410, 0.8115942028985507761, 0.8188405797101449002, 0.8260869565217391353, 0.8333333333333333703, 0.8405797101449274944, 0.8478260869565217295, 0.8550724637681159646, 0.8623188405797101996, 0.8695652173913043237, 0.8768115942028985588, 0.8840579710144927938, 0.8913043478260869179, 0.8985507246376811530, 0.9057971014492753881, 0.9130434782608695121, 0.9202898550724637472, 0.9275362318840579823, 0.9347826086956522174, 0.9420289855072463414, 0.9492753623188405765, 0.9565217391304348116, 0.9637681159420289356, 0.9662082893573751274, 0.9758703722509488587 ),
 .UNSPECIFIED. ) 
 GEOMETRIC_REPRESENTATION_ITEM ( )  RATIONAL_B_SPLINE_SURFACE ( (
 ( 1.000000000000000000, 0.8660254037844387076, 1.000000000000000000, 0.8660254037844387076, 1.000000000000000000, 0.8660254037844387076, 1.000000000000000000, 0.8660254037844387076, 1.000000000000000000, 0.8660254037844387076, 1.000000000000000000, 0.8660254037844387076, 1.000000000000000000, 0.8660254037844387076, 1.000000000000000000, 0.8660254037844387076, 1.000000000000000000, 0.8660254037844387076, 1.000000000000000000, 0.8660254037844387076, 1.000000000000000000, 0.8660254037844387076, 1.000000000000000000, 0.8660254037844387076, 1.000000000000000000, 0.8660254037844387076, 1.000000000000000000, 0.8660254037844387076, 1.000000000000000000, 0.8660254037844387076, 1.000000000000000000, 0.8660254037844387076, 1.000000000000000000, 0.8660254037844387076, 1.000000000000000000, 0.8660254037844387076, 1.000000000000000000, 0.8660254037844387076, 1.000000000000000000, 0.8660254037844387076, 1.000000000000000000, 0.8660254037844387076, 1.000000000000000000, 0.8660254037844387076, 1.000000000000000000, 0.8660254037844387076, 1.000000000000000000, 0.8660254037844387076, 1.000000000000000000, 0.8660254037844387076, 1.000000000000000000, 0.8660254037844387076, 1.000000000000000000, 0.8660254037844387076, 1.000000000000000000, 0.8660254037844387076, 1.000000000000000000, 0.8660254037844387076, 1.000000000000000000, 0.8660254037844387076, 1.000000000000000000, 0.8660254037844387076, 1.000000000000000000, 0.8660254037844387076, 1.000000000000000000, 0.8660254037844387076, 1.000000000000000000, 0.8660254037844387076, 1.000000000000000000, 0.8660254037844387076, 1.000000000000000000, 0.8660254037844387076, 1.000000000000000000, 0.8660254037844387076, 1.000000000000000000, 0.8660254037844387076, 1.000000000000000000, 0.8660254037844387076, 1.000000000000000000, 0.8660254037844387076, 1.000000000000000000, 0.8660254037844387076, 1.000000000000000000, 0.8660254037844387076, 1.000000000000000000, 0.8660254037844387076, 1.000000000000000000, 0.8660254037844387076, 1.000000000000000000, 0.8660254037844387076, 1.000000000000000000, 0.8660254037844387076, 1.000000000000000000, 0.8660254037844387076, 1.000000000000000000, 0.8660254037844387076, 1.000000000000000000, 0.8660254037844387076, 1.000000000000000000, 0.8660254037844387076, 1.000000000000000000, 0.8660254037844387076, 1.000000000000000000, 0.8660254037844387076, 1.000000000000000000, 0.8660254037844387076, 1.000000000000000000, 0.8660254037844387076, 1.000000000000000000, 0.8660254037844387076, 1.000000000000000000, 0.8660254037844387076, 1.000000000000000000, 0.8660254037844387076, 1.000000000000000000, 0.8660254037844387076, 1.000000000000000000, 0.8660254037844387076, 1.000000000000000000, 0.8660254037844387076, 1.000000000000000000, 0.8660254037844387076, 1.000000000000000000, 0.8660254037844387076, 1.000000000000000000, 0.8660254037844387076, 1.000000000000000000, 0.8660254037844387076, 1.000000000000000000, 0.8660254037844387076, 1.000000000000000000, 0.8660254037844387076, 1.000000000000000000, 0.8660254037844387076, 1.000000000000000000, 0.8660254037844387076, 1.000000000000000000, 0.8660254037844387076, 1.000000000000000000, 0.8660254037844387076, 1.000000000000000000, 0.8660254037844387076, 1.000000000000000000, 0.8660254037844387076, 1.000000000000000000, 0.8660254037844387076, 1.000000000000000000, 0.8660254037844387076, 1.000000000000000000, 0.8660254037844387076, 1.000000000000000000, 0.8660254037844387076, 1.000000000000000000, 0.8660254037844387076, 1.000000000000000000, 0.8660254037844387076, 1.000000000000000000, 0.8660254037844387076, 1.000000000000000000, 0.8660254037844387076, 1.000000000000000000, 0.8660254037844387076, 1.000000000000000000, 0.8660254037844387076, 1.000000000000000000, 0.8660254037844387076, 1.000000000000000000, 0.8660254037844387076, 1.000000000000000000, 0.8660254037844387076, 1.000000000000000000, 0.8660254037844387076, 1.000000000000000000, 0.8660254037844387076, 1.000000000000000000, 0.8660254037844387076, 1.000000000000000000, 0.8660254037844387076, 1.000000000000000000, 0.8660254037844387076, 1.000000000000000000, 0.8660254037844387076, 1.000000000000000000, 0.8660254037844387076, 1.000000000000000000, 0.8660254037844387076, 1.000000000000000000, 0.8660254037844387076, 1.000000000000000000, 0.8660254037844387076, 1.000000000000000000, 0.8660254037844387076, 1.000000000000000000, 0.8660254037844387076, 1.000000000000000000, 0.8660254037844387076, 1.000000000000000000, 0.8660254037844387076, 1.000000000000000000, 0.8660254037844387076, 1.000000000000000000, 0.8660254037844387076, 1.000000000000000000, 0.8660254037844387076, 1.000000000000000000, 0.8660254037844387076, 1.000000000000000000, 0.8660254037844387076, 1.000000000000000000, 0.8660254037844387076, 1.000000000000000000, 0.8660254037844387076, 1.000000000000000000, 0.8660254037844387076, 1.000000000000000000, 0.8660254037844387076, 1.000000000000000000, 0.8660254037844387076, 1.000000000000000000, 0.8660254037844387076, 1.000000000000000000, 0.8660254037844387076, 1.000000000000000000, 0.8660254037844387076, 1.000000000000000000, 0.8660254037844387076, 1.000000000000000000, 0.8660254037844387076, 1.000000000000000000, 0.8660254037844387076, 1.000000000000000000, 0.8660254037844387076, 1.000000000000000000, 0.8660254037844387076, 1.000000000000000000, 0.8660254037844387076, 1.000000000000000000, 0.8660254037844387076, 1.000000000000000000, 0.8660254037844387076, 1.000000000000000000, 0.8660254037844387076, 1.000000000000000000, 0.8660254037844387076, 1.000000000000000000, 0.8660254037844387076, 1.000000000000000000, 0.8660254037844387076, 1.000000000000000000, 0.8660254037844387076, 1.000000000000000000, 0.8660254037844387076, 1.000000000000000000, 0.8660254037844387076, 1.000000000000000000, 0.8660254037844387076, 1.000000000000000000, 0.8660254037844387076, 1.000000000000000000, 0.8660254037844387076, 1.000000000000000000, 0.8660254037844387076, 1.000000000000000000, 0.8660254037844387076, 1.000000000000000000, 0.8660254037844387076, 1.000000000000000000, 0.9548848677736607726, 0.9401542295229587953, 0.9401542295229587953, 0.9401542295229587953),
 ( 1.000000000000000000, 0.8660254037844387076, 1.000000000000000000, 0.8660254037844387076, 1.000000000000000000, 0.8660254037844387076, 1.000000000000000000, 0.8660254037844387076, 1.000000000000000000, 0.8660254037844387076, 1.000000000000000000, 0.8660254037844387076, 1.000000000000000000, 0.8660254037844387076, 1.000000000000000000, 0.8660254037844387076, 1.000000000000000000, 0.8660254037844387076, 1.000000000000000000, 0.8660254037844387076, 1.000000000000000000, 0.8660254037844387076, 1.000000000000000000, 0.8660254037844387076, 1.000000000000000000, 0.8660254037844387076, 1.000000000000000000, 0.8660254037844387076, 1.000000000000000000, 0.8660254037844387076, 1.000000000000000000, 0.8660254037844387076, 1.000000000000000000, 0.8660254037844387076, 1.000000000000000000, 0.8660254037844387076, 1.000000000000000000, 0.8660254037844387076, 1.000000000000000000, 0.8660254037844387076, 1.000000000000000000, 0.8660254037844387076, 1.000000000000000000, 0.8660254037844387076, 1.000000000000000000, 0.8660254037844387076, 1.000000000000000000, 0.8660254037844387076, 1.000000000000000000, 0.8660254037844387076, 1.000000000000000000, 0.8660254037844387076, 1.000000000000000000, 0.8660254037844387076, 1.000000000000000000, 0.8660254037844387076, 1.000000000000000000, 0.8660254037844387076, 1.000000000000000000, 0.8660254037844387076, 1.000000000000000000, 0.8660254037844387076, 1.000000000000000000, 0.8660254037844387076, 1.000000000000000000, 0.8660254037844387076, 1.000000000000000000, 0.8660254037844387076, 1.000000000000000000, 0.8660254037844387076, 1.000000000000000000, 0.8660254037844387076, 1.000000000000000000, 0.8660254037844387076, 1.000000000000000000, 0.8660254037844387076, 1.000000000000000000, 0.8660254037844387076, 1.000000000000000000, 0.8660254037844387076, 1.000000000000000000, 0.8660254037844387076, 1.000000000000000000, 0.8660254037844387076, 1.000000000000000000, 0.8660254037844387076, 1.000000000000000000, 0.8660254037844387076, 1.000000000000000000, 0.8660254037844387076, 1.000000000000000000, 0.8660254037844387076, 1.000000000000000000, 0.8660254037844387076, 1.000000000000000000, 0.8660254037844387076, 1.000000000000000000, 0.8660254037844387076, 1.000000000000000000, 0.8660254037844387076, 1.000000000000000000, 0.8660254037844387076, 1.000000000000000000, 0.8660254037844387076, 1.000000000000000000, 0.8660254037844387076, 1.000000000000000000, 0.8660254037844387076, 1.000000000000000000, 0.8660254037844387076, 1.000000000000000000, 0.8660254037844387076, 1.000000000000000000, 0.8660254037844387076, 1.000000000000000000, 0.8660254037844387076, 1.000000000000000000, 0.8660254037844387076, 1.000000000000000000, 0.8660254037844387076, 1.000000000000000000, 0.8660254037844387076, 1.000000000000000000, 0.8660254037844387076, 1.000000000000000000, 0.8660254037844387076, 1.000000000000000000, 0.8660254037844387076, 1.000000000000000000, 0.8660254037844387076, 1.000000000000000000, 0.8660254037844387076, 1.000000000000000000, 0.8660254037844387076, 1.000000000000000000, 0.8660254037844387076, 1.000000000000000000, 0.8660254037844387076, 1.000000000000000000, 0.8660254037844387076, 1.000000000000000000, 0.8660254037844387076, 1.000000000000000000, 0.8660254037844387076, 1.000000000000000000, 0.8660254037844387076, 1.000000000000000000, 0.8660254037844387076, 1.000000000000000000, 0.8660254037844387076, 1.000000000000000000, 0.8660254037844387076, 1.000000000000000000, 0.8660254037844387076, 1.000000000000000000, 0.8660254037844387076, 1.000000000000000000, 0.8660254037844387076, 1.000000000000000000, 0.8660254037844387076, 1.000000000000000000, 0.8660254037844387076, 1.000000000000000000, 0.8660254037844387076, 1.000000000000000000, 0.8660254037844387076, 1.000000000000000000, 0.8660254037844387076, 1.000000000000000000, 0.8660254037844387076, 1.000000000000000000, 0.8660254037844387076, 1.000000000000000000, 0.8660254037844387076, 1.000000000000000000, 0.8660254037844387076, 1.000000000000000000, 0.8660254037844387076, 1.000000000000000000, 0.8660254037844387076, 1.000000000000000000, 0.8660254037844387076, 1.000000000000000000, 0.8660254037844387076, 1.000000000000000000, 0.8660254037844387076, 1.000000000000000000, 0.8660254037844387076, 1.000000000000000000, 0.8660254037844387076, 1.000000000000000000, 0.8660254037844387076, 1.000000000000000000, 0.8660254037844387076, 1.000000000000000000, 0.8660254037844387076, 1.000000000000000000, 0.8660254037844387076, 1.000000000000000000, 0.8660254037844387076, 1.000000000000000000, 0.8660254037844387076, 1.000000000000000000, 0.8660254037844387076, 1.000000000000000000, 0.8660254037844387076, 1.000000000000000000, 0.8660254037844387076, 1.000000000000000000, 0.8660254037844387076, 1.000000000000000000, 0.8660254037844387076, 1.000000000000000000, 0.8660254037844387076, 1.000000000000000000, 0.8660254037844387076, 1.000000000000000000, 0.8660254037844387076, 1.000000000000000000, 0.8660254037844387076, 1.000000000000000000, 0.8660254037844387076, 1.000000000000000000, 0.8660254037844387076, 1.000000000000000000, 0.8660254037844387076, 1.000000000000000000, 0.8660254037844387076, 1.000000000000000000, 0.8660254037844387076, 1.000000000000000000, 0.8660254037844387076, 1.000000000000000000, 0.8660254037844387076, 1.000000000000000000, 0.8660254037844387076, 1.000000000000000000, 0.8660254037844387076, 1.000000000000000000, 0.8660254037844387076, 1.000000000000000000, 0.8660254037844387076, 1.000000000000000000, 0.8660254037844387076, 1.000000000000000000, 0.8660254037844387076, 1.000000000000000000, 0.8660254037844387076, 1.000000000000000000, 0.8660254037844387076, 1.000000000000000000, 0.8660254037844387076, 1.000000000000000000, 0.8660254037844387076, 1.000000000000000000, 0.8660254037844387076, 1.000000000000000000, 0.8660254037844387076, 1.000000000000000000, 0.8660254037844387076, 1.000000000000000000, 0.8660254037844387076, 1.000000000000000000, 0.8660254037844387076, 1.000000000000000000, 0.8660254037844387076, 1.000000000000000000, 0.9548848677736607726, 0.9401542295229587953, 0.9401542295229587953, 0.9401542295229587953) ) ) 
 REPRESENTATION_ITEM ( '' )  SURFACE ( )  );
#33746=CARTESIAN_POINT ( 'NONE',  ( 19.68408634441911786, -5.407089921784861808, -9.046874999385529748 ) ) ;
#33750=CARTESIAN_POINT ( 'NONE',  ( 22.80587116629410360, -3.604726614523235284, -0.4031249993855248182 ) ) ;
#33757=CARTESIAN_POINT ( 'NONE',  ( 10.56230152254411259, -3.464101615137757051, -1.199999998771033916 ) ) ;
#33763=UNCERTAINTY_MEASURE_WITH_UNIT (LENGTH_MEASURE( 1.000000000000000082E-05 ), #28256, 'distance_accuracy_value', 'NONE');
#33767=CARTESIAN_POINT ( 'NONE',  ( 13.56230152254410726, 5.196152422706636465, -8.625000000000021316 ) ) ;
#33780=ORIENTED_EDGE ( 'NONE', *, *, #34020, .F. ) ;
#33781=EDGE_CURVE ( 'NONE', #6483, #28398, #19769, .T. ) ;
#33784=CARTESIAN_POINT ( 'NONE',  ( 13.44051670066911264, -5.407089921784865361, -5.521874999385528504 ) ) ;
#33790=CARTESIAN_POINT ( 'NONE',  ( 16.56230152254411792, 7.209453229046482114, -0.7593749993855121172 ) ) ;
#33791=CARTESIAN_POINT ( 'NONE',  ( 10.56230152254411081, 0.000000000000000000, -9.337499998771036758 ) ) ;
#33795=CARTESIAN_POINT ( 'NONE',  ( 13.56230152254410903, 5.196152422706636465, -2.775000000000027445 ) ) ;
#33797=EDGE_CURVE ( 'NONE', #7868, #4455, #1866, .T. ) ;
#33800=AXIS2_PLACEMENT_3D ( 'NONE', #2568, #2009, #13583 ) ;
#33801=FACE_OUTER_BOUND ( 'NONE', #11728, .T. ) ;
#33809=CARTESIAN_POINT ( 'NONE',  ( 16.56230152254411436, 6.928203230275514990, -2.812500000000029754 ) ) ;
#33815=CARTESIAN_POINT ( 'NONE',  ( 16.56230152254410726, 0.000000000000000000, -10.00000000000000000 ) ) ;
#33822=ORIENTED_EDGE ( 'NONE', *, *, #13434, .F. ) ;
#33827=CARTESIAN_POINT ( 'NONE',  ( 22.80587116629410360, 3.604726614523238837, -8.428124999385516958 ) ) ;
#33860=CARTESIAN_POINT ( 'NONE',  ( 22.80587116629410360, 7.646167579472015790E-16, -7.565624999385539340 ) ) ;
#33869=CARTESIAN_POINT ( 'NONE',  ( 16.56230152254411436, 7.209453229046482114, -1.659374999385503591 ) ) ;
#33871=ORIENTED_EDGE ( 'NONE', *, *, #10195, .F. ) ;
#33875=CARTESIAN_POINT ( 'NONE',  ( 22.80587116629411071, 3.604726614523238837, -1.228124999385522331 ) ) ;
#33891=AXIS2_PLACEMENT_3D ( 'NONE', #28989, #11566, #3217 ) ;
#33896=CARTESIAN_POINT ( 'NONE',  ( 10.56230152254411081, 0.000000000000000000, -9.337499998771036758 ) ) ;
#33899=CARTESIAN_POINT ( 'NONE',  ( 16.56230152254411436, -7.209453229046482114, -9.984374999385536853 ) ) ;
#33900=CARTESIAN_POINT ( 'NONE',  ( 19.68408634441911076, 5.407089921784862696, -7.546874999385555505 ) ) ;
#33930=CARTESIAN_POINT ( 'NONE',  ( 16.56230152254411436, 7.209453229046482114, -7.509374999385479477 ) ) ;
#33934=CARTESIAN_POINT ( 'NONE',  ( 19.68408634441910721, 5.407089921784857367, -2.540624999385538096 ) ) ;
#33937=CARTESIAN_POINT ( 'NONE',  ( 13.56230152254411614, -5.196152422706632912, -7.462499998771049192 ) ) ;
#33940=CARTESIAN_POINT ( 'NONE',  ( 22.56230152254410370, -3.464101615137751278, -1.049999998770981602 ) ) ;
#33942=CARTESIAN_POINT ( 'NONE',  ( 10.56230152254411081, 0.000000000000000000, -9.337499998771036758 ) ) ;
#33948=CARTESIAN_POINT ( 'NONE',  ( 10.31873187879410736, 3.604726614523236616, -0.1781249993854788494 ) ) ;
#33951=CARTESIAN_POINT ( 'NONE',  ( 22.56230152254438437, -3.464101615137601176, -7.912500000000031619 ) ) ;
#33957=DIRECTION ( 'NONE',  ( 1.000000000000000000, 0.000000000000000000, 0.000000000000000000 ) ) ;
#33958=CARTESIAN_POINT ( 'NONE',  ( 16.56230152254410726, 6.928203230275506996, -6.749999998770969789 ) ) ;
#33964=CARTESIAN_POINT ( 'NONE',  ( 22.80587116629411781, 3.604726614523243278, -5.784374999385522464 ) ) ;
#33970=CARTESIAN_POINT ( 'NONE',  ( 16.56230152254411436, -7.209453229046482114, -2.334374999385513849 ) ) ;
#33975=CARTESIAN_POINT ( 'NONE',  ( 22.56230152254419252, 3.464101615137697987, -0.5249999987710254334 ) ) ;
#33984=AXIS2_PLACEMENT_3D ( 'NONE', #17314, #3271, #25833 ) ;
#33987=CARTESIAN_POINT ( 'NONE',  ( 19.56230152254412502, -5.196152422706635576, -3.000000000000058176 ) ) ;
#34005=CARTESIAN_POINT ( 'NONE',  ( 22.80587116629411071, 7.646167579472015790E-16, -8.915624999385585170 ) ) ;
#34020=EDGE_CURVE ( 'NONE', #32727, #36330, #10788, .T. ) ;
#34043=CARTESIAN_POINT ( 'NONE',  ( 16.56230152254411081, -7.209453229046475009, -6.328124999385527083 ) ) ;
#34052=CARTESIAN_POINT ( 'NONE',  ( 22.80587116629411426, 7.646167579472024665E-16, -2.221874999385531346 ) ) ;
#34058=CARTESIAN_POINT ( 'NONE',  ( 19.68408634441910721, 5.407089921784857367, -2.540624999385538096 ) ) ;
#34061=DIRECTION ( 'NONE',  ( 1.000000000000000000, 0.000000000000000000, 0.000000000000000000 ) ) ;
#34073=CARTESIAN_POINT ( 'NONE',  ( 22.80587116629411071, -3.604726614523235284, -9.853124999385530103 ) ) ;
#34084=CARTESIAN_POINT ( 'NONE',  ( 10.31873187879410558, 0.000000000000000000, -6.946874999385510563 ) ) ;
#34085=CARTESIAN_POINT ( 'NONE',  ( 10.56230152254410903, 0.000000000000000000, -5.551115123125782702E-14 ) ) ;
#34093=ORIENTED_EDGE ( 'NONE', *, *, #23960, .F. ) ;
#34099=CARTESIAN_POINT ( 'NONE',  ( 22.56230152254290644, 3.464101615138464041, -4.237500000000027356 ) ) ;
#34103=ORIENTED_EDGE ( 'NONE', *, *, #11433, .F. ) ;
#34109=CARTESIAN_POINT ( 'NONE',  ( 15.26155779561005232, -6.106572496351636126, -10.00000000000000000 ) ) ;
#34111=CARTESIAN_POINT ( 'NONE',  ( 19.68408634441911076, 5.407089921784862696, -8.446874999385538985 ) ) ;
#34115=CARTESIAN_POINT ( 'NONE',  ( 22.80587116629410716, 7.646167579472015790E-16, -3.515624999385541294 ) ) ;
#34122=CARTESIAN_POINT ( 'NONE',  ( 22.56230152254411436, 3.464101615137755275, -4.574999998771017928 ) ) ;
#34125=( NAMED_UNIT ( * ) SI_UNIT ( $, .STERADIAN. ) SOLID_ANGLE_UNIT ( ) );
#34128=FACE_OUTER_BOUND ( 'NONE', #25947, .T. ) ;
#34130=EDGE_CURVE ( 'NONE', #6556, #35189, #24681, .T. ) ;
#34131=CARTESIAN_POINT ( 'NONE',  ( 22.80587116629411071, 3.604726614523238837, -0.7781249993855585689 ) ) ;
#34132=CARTESIAN_POINT ( 'NONE',  ( 10.56230152254410726, 0.000000000000000000, -8.887499998771003717 ) ) ;
#34137=( GEOMETRIC_REPRESENTATION_CONTEXT ( 3 ) GLOBAL_UNCERTAINTY_ASSIGNED_CONTEXT ( ( #3567 ) ) GLOBAL_UNIT_ASSIGNED_CONTEXT ( ( #34263, #33570, #1346 ) ) REPRESENTATION_CONTEXT ( 'NONE', 'WORKASPACE' ) );
#34138=CARTESIAN_POINT ( 'NONE',  ( 22.56230152254531518, 3.464101615137058943, -2.324999998771022813 ) ) ;
#34143=CARTESIAN_POINT ( 'NONE',  ( 22.56230152254353527, -3.464101615138088786, -5.549999998771012244 ) ) ;
#34149=CARTESIAN_POINT ( 'NONE',  ( 10.31873187879410736, -3.604726614523244610, -6.909374999385495819 ) ) ;
#34152=EDGE_CURVE ( 'NONE', #33087, #11055, #31123, .T. ) ;
#34154=CARTESIAN_POINT ( 'NONE',  ( 22.80587116629412492, 3.604726614523243278, -1.284374999385501370 ) ) ;
#34155=EDGE_CURVE ( 'NONE', #20388, #23009, #21851, .T. ) ;
#34168=CARTESIAN_POINT ( 'NONE',  ( 16.56230152254411792, 6.928203230275514990, -1.462500000000010125 ) ) ;
#34175=CARTESIAN_POINT ( 'NONE',  ( 13.56230152254411436, -5.196152422706638241, -3.075000000000049916 ) ) ;
#34188=ORIENTED_EDGE ( 'NONE', *, *, #5656, .T. ) ;
#34193=CARTESIAN_POINT ( 'NONE',  ( 10.31873187879411091, 0.000000000000000000, -9.140624999385559946 ) ) ;
#34197=ORIENTED_EDGE ( 'NONE', *, *, #31562, .T. ) ;
#34198=EDGE_LOOP ( 'NONE', ( #33201, #36193, #7088, #29075, #24235 ) ) ;
#34199=( BOUNDED_CURVE ( )  B_SPLINE_CURVE ( 2, ( #2362, #32098, #6130, #26786, #23766, #12388, #29630 ),
 .UNSPECIFIED., .F., .F. ) 
 B_SPLINE_CURVE_WITH_KNOTS ( ( 3, 2, 2, 3 ),
 ( 0.08695652173912893357, 0.09420289855072321028, 0.1014492753623174870, 0.1086956521739117498 ),
 .UNSPECIFIED. ) 
 CURVE ( )  GEOMETRIC_REPRESENTATION_ITEM ( )  RATIONAL_B_SPLINE_CURVE ( ( 1.000000000000027534, 0.8660254037844109520, 1.000000000000000000, 0.8660254037844387076, 1.000000000000000000, 0.8660254037844625774, 0.9999999999999761302 ) ) 
 REPRESENTATION_ITEM ( '' )  );
#34229=CARTESIAN_POINT ( 'NONE',  ( 22.80587116629411071, 3.604726614523238837, -6.178124999385540050 ) ) ;
#34238=CARTESIAN_POINT ( 'NONE',  ( 19.68408634441912142, -5.407089921784861808, -2.746874999385529037 ) ) ;
#34242=( BOUNDED_CURVE ( )  B_SPLINE_CURVE ( 2, ( #13261, #7574, #24995, #36920, #33532, #10593, #31069 ),
 .UNSPECIFIED., .F., .F. ) 
 B_SPLINE_CURVE_WITH_KNOTS ( ( 3, 2, 2, 3 ),
 ( 0.5652173913043474496, 0.5724637681159416847, 0.5797101449275359197, 0.5869565217391301548 ),
 .UNSPECIFIED. ) 
 CURVE ( )  GEOMETRIC_REPRESENTATION_ITEM ( )  RATIONAL_B_SPLINE_CURVE ( ( 1.000000000000006217, 0.8660254037844326014, 1.000000000000000000, 0.8660254037844387076, 1.000000000000000000, 0.8660254037844448138, 0.9999999999999938938 ) ) 
 REPRESENTATION_ITEM ( '' )  );
#34245=CARTESIAN_POINT ( 'NONE',  ( 13.44051670066911264, -5.407089921784859143, -2.765624999385540850 ) ) ;
#34263=( LENGTH_UNIT ( ) NAMED_UNIT ( * ) SI_UNIT ( .MILLI., .METRE. ) );
#34269=CARTESIAN_POINT ( 'NONE',  ( 16.56230152254411436, -6.928203230275506996, -10.12499999877101864 ) ) ;
#34274=CARTESIAN_POINT ( 'NONE',  ( 16.56230152254411436, 7.209453229046482114, -8.409374999385503813 ) ) ;
#34277=FACE_BOUND ( 'NONE', #18885, .T. ) ;
#34282=CARTESIAN_POINT ( 'NONE',  ( 10.56230152254383903, -3.464101615137600287, -0.4125000000000343392 ) ) ;
#34290=CARTESIAN_POINT ( 'NONE',  ( 19.56230152254411792, 5.196152422706637353, -4.200000000000036593 ) ) ;
#34304=CARTESIAN_POINT ( 'NONE',  ( 19.68408634441910721, -5.407089921784855591, -4.040624999385538985 ) ) ;
#34305=( BOUNDED_CURVE ( )  B_SPLINE_CURVE ( 2, ( #24318, #27340, #21107, #26957, #21664, #15791, #30187 ),
 .UNSPECIFIED., .F., .F. ) 
 B_SPLINE_CURVE_WITH_KNOTS ( ( 3, 2, 2, 3 ),
 ( 0.5217391304347815950, 0.5289855072463750529, 0.5362318840579683998, 0.5434782608695617467 ),
 .UNSPECIFIED. ) 
 CURVE ( )  GEOMETRIC_REPRESENTATION_ITEM ( )  RATIONAL_B_SPLINE_CURVE ( ( 1.000000000000018430, 0.8660254037844202779, 1.000000000000000000, 0.8660254037844387076, 1.000000000000000000, 0.8660254037845023234, 0.9999999999999363842 ) ) 
 REPRESENTATION_ITEM ( '' )  );
#34307=CARTESIAN_POINT ( 'NONE',  ( 13.56230152254411436, -5.196152422706632912, -1.612499998771027565 ) ) ;
#34310=CARTESIAN_POINT ( 'NONE',  ( 19.56230152254410370, 5.196152422706631135, -2.737499998770986931 ) ) ;
#34318=CARTESIAN_POINT ( 'NONE',  ( 13.44051670066911441, -5.407089921784859143, -2.315624999385534899 ) ) ;
#34325=DIRECTION ( 'NONE',  ( 0.000000000000000000, 0.000000000000000000, 1.000000000000000000 ) ) ;
#34327=CARTESIAN_POINT ( 'NONE',  ( 13.56230152254411259, -5.196152422706632912, -8.812499998771039955 ) ) ;
#34335=CARTESIAN_POINT ( 'NONE',  ( 13.44051670066911086, 5.407089921784862696, -8.371874999385548577 ) ) ;
#34339=CARTESIAN_POINT ( 'NONE',  ( 19.68408634441912142, -5.407089921784861808, -1.396874999385538940 ) ) ;
#34340=AXIS2_PLACEMENT_3D ( 'NONE', #17041, #37112, #33722 ) ;
#34344=EDGE_CURVE ( 'NONE', #13979, #32302, #22474, .T. ) ;
#34346=CARTESIAN_POINT ( 'NONE',  ( 16.56230152254411436, 6.928203230275506996, -0.4499999987709982219 ) ) ;
#34358=CARTESIAN_POINT ( 'NONE',  ( 22.56230152254412147, -3.464101615137755275, -4.312500000000036415 ) ) ;
#34379=CARTESIAN_POINT ( 'NONE',  ( 22.80587116629411071, -3.604726614523238837, -1.359374999385495775 ) ) ;
#34415=CARTESIAN_POINT ( 'NONE',  ( 19.68408634441910721, -5.407089921784855591, -6.740624999385547156 ) ) ;
#34416=CYLINDRICAL_SURFACE ( 'NONE', #32182, 5.999999999999998224 ) ;
#34422=CARTESIAN_POINT ( 'NONE',  ( 15.06230152254410548, 0.000000000000000000, 10.00000000000000000 ) ) ;
#34429=CARTESIAN_POINT ( 'NONE',  ( 16.56230152254411081, -7.209453229046475009, -1.828124999385505989 ) ) ;
#34458=CARTESIAN_POINT ( 'NONE',  ( 10.31873187879410736, 0.000000000000000000, -7.846874999385494931 ) ) ;
#34476=ORIENTED_EDGE ( 'NONE', *, *, #6126, .F. ) ;
#34480=CARTESIAN_POINT ( 'NONE',  ( 16.56230152254411436, -6.928203230275514990, -2.137500000000051692 ) ) ;
#34486=EDGE_CURVE ( 'NONE', #28877, #32302, #12133, .T. ) ;
#34488=CARTESIAN_POINT ( 'NONE',  ( 19.68408634441910721, 5.407089921784857367, -2.090624999385559679 ) ) ;
#34493=CARTESIAN_POINT ( 'NONE',  ( 13.56230152254410548, 5.196152422706630247, -3.562499998771007093 ) ) ;
#34521=CARTESIAN_POINT ( 'NONE',  ( 10.31873187879411091, 3.604726614523240613, -9.234374999385533300 ) ) ;
#34526=CARTESIAN_POINT ( 'NONE',  ( 10.31873187879410914, 0.000000000000000000, -1.996874999385528371 ) ) ;
#34531=CARTESIAN_POINT ( 'NONE',  ( 22.56230152254412502, 7.347880794884125653E-16, -3.375000000000044409 ) ) ;
#34536=ORIENTED_EDGE ( 'NONE', *, *, #14801, .F. ) ;
#34543=CARTESIAN_POINT ( 'NONE',  ( 13.56230152254410548, 5.196152422706636465, -4.575000000000050804 ) ) ;
#34545=CARTESIAN_POINT ( 'NONE',  ( 22.56230152254410370, 7.347880794884117764E-16, -5.512499998771014376 ) ) ;
#34549=DIRECTION ( 'NONE',  ( 0.000000000000000000, 0.000000000000000000, 1.000000000000000000 ) ) ;
#34550=CYLINDRICAL_SURFACE ( 'NONE', #29923, 5.999999999999998224 ) ;
#34559=ORIENTED_EDGE ( 'NONE', *, *, #7804, .T. ) ;
#34561=CARTESIAN_POINT ( 'NONE',  ( 10.31873187879411091, -3.604726614523244610, -1.059374999385519933 ) ) ;
#34566=ORIENTED_EDGE ( 'NONE', *, *, #34344, .T. ) ;
#34567=ORIENTED_EDGE ( 'NONE', *, *, #7462, .T. ) ;
#34583=CARTESIAN_POINT ( 'NONE',  ( 19.56230152254412147, -5.196152422706635576, -5.250000000000060396 ) ) ;
#34593=CARTESIAN_POINT ( 'NONE',  ( 10.31873187879411091, 0.000000000000000000, -9.140624999385559946 ) ) ;
#34594=CARTESIAN_POINT ( 'NONE',  ( 22.56230152254412147, 7.347880794884125653E-16, -8.775000000000032330 ) ) ;
#34597=CARTESIAN_POINT ( 'NONE',  ( 10.83228649186779791, 2.189148559480569300, -9.999999999999998224 ) ) ;
#34607=CARTESIAN_POINT ( 'NONE',  ( 22.80587116629411781, 3.604726614523238837, -4.378124999385524241 ) ) ;
#34613=EDGE_LOOP ( 'NONE', ( #36452, #33030, #26286, #861 ) ) ;
#34625=CARTESIAN_POINT ( 'NONE',  ( 19.68408634441910365, 5.407089921784857367, -9.740624999385548932 ) ) ;
#34632=CARTESIAN_POINT ( 'NONE',  ( 22.56230152254410370, 7.347880794884117764E-16, -10.01249999877101793 ) ) ;
#34636=CARTESIAN_POINT ( 'NONE',  ( 10.31873187879410736, 3.604726614523240613, -7.884374999385513227 ) ) ;
#34668=CARTESIAN_POINT ( 'NONE',  ( 16.56230152254411081, 7.209453229046475009, -2.953124999385511096 ) ) ;
#34674=CARTESIAN_POINT ( 'NONE',  ( 22.56230152254410726, 7.347880794884117764E-16, -3.262499998771012599 ) ) ;
#34680=CARTESIAN_POINT ( 'NONE',  ( 22.56230152254289578, 3.464101615138464041, -8.287500000000052935 ) ) ;
#34697=ORIENTED_EDGE ( 'NONE', *, *, #1847, .T. ) ;
#34701=CARTESIAN_POINT ( 'NONE',  ( 19.68408634441911076, 5.407089921784862696, -7.996874999385533478 ) ) ;
#34705=CARTESIAN_POINT ( 'NONE',  ( 10.31873187879410914, 0.000000000000000000, -4.696874999385508787 ) ) ;
#34717=VERTEX_POINT ( 'NONE', #1696 ) ;
#34718=DIRECTION ( 'NONE',  ( 0.000000000000000000, 0.000000000000000000, 1.000000000000000000 ) ) ;
#34727=CARTESIAN_POINT ( 'NONE',  ( 10.56230152254410726, 0.000000000000000000, -5.400000000000043876 ) ) ;
#34747=CARTESIAN_POINT ( 'NONE',  ( 16.56230152254411436, -7.209453229046482114, -1.884374999385517446 ) ) ;
#34754=ORIENTED_EDGE ( 'NONE', *, *, #19779, .T. ) ;
#34780=CARTESIAN_POINT ( 'NONE',  ( 13.44051670066911086, 5.407089921784856479, -9.665624999385530103 ) ) ;
#34781=CARTESIAN_POINT ( 'NONE',  ( 22.56230152254321197, 3.464101615138280632, -8.737500000000023803 ) ) ;
#34783=CARTESIAN_POINT ( 'NONE',  ( 15.02202517871450738, 5.832799451530069845, -10.00000000000000000 ) ) ;
#34793=CARTESIAN_POINT ( 'NONE',  ( 22.80587116629411071, -3.604726614523235284, -4.453124999385550176 ) ) ;
#34799=ORIENTED_EDGE ( 'NONE', *, *, #17122, .T. ) ;
#34800=FACE_OUTER_BOUND ( 'NONE', #2959, .T. ) ;
#34807=LINE ( 'NONE', #29113, #14955 ) ;
#34819=CARTESIAN_POINT ( 'NONE',  ( 10.56230152254294552, -3.464101615137081591, -8.399999998771011889 ) ) ;
#34823=CARTESIAN_POINT ( 'NONE',  ( 22.80587116629411426, 7.646167579472024665E-16, -8.071874999385524774 ) ) ;
#34830=CARTESIAN_POINT ( 'NONE',  ( 13.56230152254410548, 5.196152422706636465, -5.025000000000029665 ) ) ;
#34832=VERTEX_POINT ( 'NONE', #2074 ) ;
#34855=CARTESIAN_POINT ( 'NONE',  ( 13.44051670066911441, -5.407089921784859143, -5.915624999385554972 ) ) ;
#34858=FACE_OUTER_BOUND ( 'NONE', #3412, .T. ) ;
#34861=CARTESIAN_POINT ( 'NONE',  ( 16.56230152254411081, -6.928203230275506996, -2.924999998770990928 ) ) ;
#34879=AXIS2_PLACEMENT_3D ( 'NONE', #16188, #30401, #8022 ) ;
#34891=CARTESIAN_POINT ( 'NONE',  ( 19.68408634441911076, 5.407089921784862696, -7.546874999385555505 ) ) ;
#34896=CARTESIAN_POINT ( 'NONE',  ( 19.68408634441911431, 5.407089921784862696, -4.846874999385547333 ) ) ;
#34913=CARTESIAN_POINT ( 'NONE',  ( 10.56230152254410903, 3.464101615137757051, -3.637500000000027267 ) ) ;
#34916=CARTESIAN_POINT ( 'NONE',  ( 16.56230152254411081, 6.928203230275506996, -5.399999998770983467 ) ) ;
#34930=CARTESIAN_POINT ( 'NONE',  ( 16.56230152254411436, -7.209453229046482114, -2.334374999385512961 ) ) ;
#34936=ORIENTED_EDGE ( 'NONE', *, *, #5307, .T. ) ;
#34941=ADVANCED_FACE ( 'NONE', ( #18789 ), #22367, .F. ) ;
#34942=( BOUNDED_CURVE ( )  B_SPLINE_CURVE ( 2, ( #16044, #36295, #15476, #21914, #32712, #4094, #868 ),
 .UNSPECIFIED., .F., .F. ) 
 B_SPLINE_CURVE_WITH_KNOTS ( ( 3, 2, 2, 3 ),
 ( 0.5434782608695617467, 0.5507246376811569810, 0.5579710144927523263, 0.5652173913043474496 ),
 .UNSPECIFIED. ) 
 CURVE ( )  GEOMETRIC_REPRESENTATION_ITEM ( )  RATIONAL_B_SPLINE_CURVE ( ( 1.000000000000063727, 0.8660254037843750918, 1.000000000000000000, 0.8660254037844387076, 1.000000000000000000, 0.8660254037844448138, 0.9999999999999938938 ) ) 
 REPRESENTATION_ITEM ( '' )  );
#34965=CARTESIAN_POINT ( 'NONE',  ( 10.31873187879411091, 3.604726614523236616, -8.278124999385530813 ) ) ;
#34979=CARTESIAN_POINT ( 'NONE',  ( 13.44051670066911086, 5.407089921784856479, -4.265624999385542182 ) ) ;
#34996=DIRECTION ( 'NONE',  ( 1.000000000000000000, 0.000000000000000000, 0.000000000000000000 ) ) ;
#35013=CARTESIAN_POINT ( 'NONE',  ( 13.44051670066911086, 5.407089921784862696, -8.371874999385548577 ) ) ;
#35015=CARTESIAN_POINT ( 'NONE',  ( 19.68408634441910721, 5.407089921784857367, -1.190624999385520022 ) ) ;
#35041=CARTESIAN_POINT ( 'NONE',  ( 13.44051670066911619, -5.407089921784859143, -5.015624999385570604 ) ) ;
#35044=CARTESIAN_POINT ( 'NONE',  ( 22.56230152254345356, -3.464101615138130530, -1.499999998770985554 ) ) ;
#35046=CARTESIAN_POINT ( 'NONE',  ( 22.56230152254410370, 3.464101615137755275, -5.924999998771004250 ) ) ;
#35065=DIRECTION ( 'NONE',  ( 1.000000000000000000, 0.000000000000000000, 0.000000000000000000 ) ) ;
#35078=CARTESIAN_POINT ( 'NONE',  ( 16.56230152254411792, -7.209453229046482114, -4.584374999385491201 ) ) ;
#35092=AXIS2_PLACEMENT_3D ( 'NONE', #7987, #10265, #7805 ) ;
#35097=CARTESIAN_POINT ( 'NONE',  ( 13.56230152254410726, 5.196152422706636465, -4.125000000000045297 ) ) ;
#35100=CARTESIAN_POINT ( 'NONE',  ( 19.56230152254411081, 5.196152422706631135, -5.437499998771022192 ) ) ;
#35115=CARTESIAN_POINT ( 'NONE',  ( 22.80587116629411426, 7.646167579472024665E-16, -2.671874999385509319 ) ) ;
#35120=EDGE_LOOP ( 'NONE', ( #34559, #12537, #15315, #22138 ) ) ;
#35141=EDGE_CURVE ( 'NONE', #28877, #1340, #13496, .T. ) ;
#35146=CARTESIAN_POINT ( 'NONE',  ( 19.68408634441910721, 5.407089921784857367, -8.840624999385537919 ) ) ;
#35149=CARTESIAN_POINT ( 'NONE',  ( 10.59851679596256702, -1.739360772546590050, -9.999999999999994671 ) ) ;
#35159=CARTESIAN_POINT ( 'NONE',  ( 19.68408634441910721, -5.407089921784855591, -3.590624999385533478 ) ) ;
#35174=EDGE_CURVE ( 'NONE', #29181, #15610, #21489, .T. ) ;
#35189=VERTEX_POINT ( 'NONE', #23107 ) ;
#35195=CARTESIAN_POINT ( 'NONE',  ( 22.80587116629410360, 7.646167579472015790E-16, -2.165624999385551419 ) ) ;
#35201=CARTESIAN_POINT ( 'NONE',  ( 10.56230152254410903, 0.000000000000000000, -4.950000000000037481 ) ) ;
#35212=EDGE_CURVE ( 'NONE', #16024, #26922, #155, .T. ) ;
#35218=CARTESIAN_POINT ( 'NONE',  ( 10.56230152254411081, 0.000000000000000000, -9.337499998771036758 ) ) ;
#35227=CARTESIAN_POINT ( 'NONE',  ( 19.68408634441911076, 5.407089921784857367, -5.240624999385545379 ) ) ;
#35230=CARTESIAN_POINT ( 'NONE',  ( 10.56230152254410903, 7.347880794884117764E-16, -10.00000000000000000 ) ) ;
#35232=CARTESIAN_POINT ( 'NONE',  ( 16.56230152254411081, -6.928203230275506996, -6.524999998771020771 ) ) ;
#35237=CARTESIAN_POINT ( 'NONE',  ( 19.68408634441911431, 5.407089921784862696, -4.846874999385547333 ) ) ;
#35241=CYLINDRICAL_SURFACE ( 'NONE', #20420, 5.999999999999998224 ) ;
#35262=CARTESIAN_POINT ( 'NONE',  ( 16.56230152254411436, -7.209453229046482114, -3.684374999385500171 ) ) ;
#35279=CARTESIAN_POINT ( 'NONE',  ( 10.56230152254411259, 3.464101615137757051, -6.337500000000034106 ) ) ;
#35280=VERTEX_POINT ( 'NONE', #14384 ) ;
#35287=CARTESIAN_POINT ( 'NONE',  ( 20.96920819138947323, -4.251017401976773691, -9.999999999999996447 ) ) ;
#35297=CARTESIAN_POINT ( 'NONE',  ( 10.31873187879410736, 0.000000000000000000, -3.796874999385524418 ) ) ;
#35307=CARTESIAN_POINT ( 'NONE',  ( 22.56230152254410370, 7.347880794884117764E-16, -6.412499998770998744 ) ) ;
#35319=FACE_OUTER_BOUND ( 'NONE', #13882, .T. ) ;
#35326=CARTESIAN_POINT ( 'NONE',  ( 13.56230152254411792, -5.196152422706638241, -0.8250000000000479172 ) ) ;
#35330=CARTESIAN_POINT ( 'NONE',  ( 19.68408634441910721, -5.407089921784855591, -8.990624999385548932 ) ) ;
#35344=CARTESIAN_POINT ( 'NONE',  ( 16.56230152254411436, 7.209453229046475009, -3.853124999385534988 ) ) ;
#35381=CARTESIAN_POINT ( 'NONE',  ( 16.56230152254411081, 7.209453229046475009, -0.7031249993855005487 ) ) ;
#35382=( BOUNDED_CURVE ( )  B_SPLINE_CURVE ( 2, ( #6559, #17942, #17059, #8706, #23117, #18133, #11364 ),
 .UNSPECIFIED., .F., .F. ) 
 B_SPLINE_CURVE_WITH_KNOTS ( ( 3, 2, 2, 3 ),
 ( 0.2826086956521749460, 0.2898550724637684040, 0.2971014492753618064, 0.3043478260869552643 ),
 .UNSPECIFIED. ) 
 CURVE ( )  GEOMETRIC_REPRESENTATION_ITEM ( )  RATIONAL_B_SPLINE_CURVE ( ( 0.9999999999999804601, 0.8660254037844582475, 1.000000000000000000, 0.8660254037844387076, 1.000000000000000000, 0.8660254037844623554, 0.9999999999999763522 ) ) 
 REPRESENTATION_ITEM ( '' )  );
#35387=CARTESIAN_POINT ( 'NONE',  ( 16.56230152254411792, 6.928203230275514990, -5.062500000000007994 ) ) ;
#35412=CARTESIAN_POINT ( 'NONE',  ( 16.56230152254410726, 7.209453229046475009, -5.203124999385489780 ) ) ;
#35414=CARTESIAN_POINT ( 'NONE',  ( 10.56230152254410903, 0.000000000000000000, -2.700000000000063238 ) ) ;
#35418=CARTESIAN_POINT ( 'NONE',  ( 13.56230152254411614, -5.196152422706632912, -7.012499998771043686 ) ) ;
#35426=CARTESIAN_POINT ( 'NONE',  ( 22.80587116629411781, 3.604726614523243278, -3.084374999385516514 ) ) ;
#35454=ORIENTED_EDGE ( 'NONE', *, *, #26449, .T. ) ;
#35455=CARTESIAN_POINT ( 'NONE',  ( 19.68408634441911786, -5.407089921784861808, -4.546874999385525307 ) ) ;
#35462=DIRECTION ( 'NONE',  ( 0.000000000000000000, 0.000000000000000000, 1.000000000000000000 ) ) ;
#35472=DIRECTION ( 'NONE',  ( -4.704570066849100051E-15, 0.000000000000000000, 1.000000000000000000 ) ) ;
#35474=CARTESIAN_POINT ( 'NONE',  ( 22.56230152254411792, 7.347880794884125653E-16, -6.525000000000058975 ) ) ;
#35491=CARTESIAN_POINT ( 'NONE',  ( 10.31873187879411091, 3.604726614523240613, -3.834374999385520066 ) ) ;
#35505=CARTESIAN_POINT ( 'NONE',  ( 16.56230152254411436, -7.209453229046475009, -0.9281249993855145153 ) ) ;
#35522=LINE ( 'NONE', #29650, #19886 ) ;
#35539=CARTESIAN_POINT ( 'NONE',  ( 22.80587116629410360, 7.646167579472015790E-16, -7.115624999385533833 ) ) ;
#35543=ADVANCED_FACE ( 'NONE', ( #524 ), #26874, .F. ) ;
#35548=CARTESIAN_POINT ( 'NONE',  ( 22.56230152254546439, -3.464101615136981227, -2.062499999999976463 ) ) ;
#35575=CARTESIAN_POINT ( 'NONE',  ( 22.80587116629410360, -3.604726614523235284, -4.003124999385554439 ) ) ;
#35582=DIRECTION ( 'NONE',  ( 0.000000000000000000, 0.000000000000000000, 1.000000000000000000 ) ) ;
#35604=CARTESIAN_POINT ( 'NONE',  ( 16.56230152254411436, -7.209453229046475009, -4.528124999385512162 ) ) ;
#35612=CARTESIAN_POINT ( 'NONE',  ( 16.56230152254411081, 6.928203230275506996, -5.399999998770982579 ) ) ;
#35616=CARTESIAN_POINT ( 'NONE',  ( 10.31873187879411091, 3.604726614523240613, -5.184374999385507721 ) ) ;
#35634=ORIENTED_EDGE ( 'NONE', *, *, #5307, .F. ) ;
#35635=VERTEX_POINT ( 'NONE', #36465 ) ;
#35645=CARTESIAN_POINT ( 'NONE',  ( 22.80587116629411781, -3.604726614523238837, -4.959374999385526728 ) ) ;
#35664=CARTESIAN_POINT ( 'NONE',  ( 13.56230152254410548, 5.196152422706636465, -7.275000000000058975 ) ) ;
#35671=CARTESIAN_POINT ( 'NONE',  ( 16.56230152254410726, 0.000000000000000000, -10.00000000000000000 ) ) ;
#35678=ORIENTED_EDGE ( 'NONE', *, *, #31917, .F. ) ;
#35681=CARTESIAN_POINT ( 'NONE',  ( 13.44051670066911086, 5.407089921784862696, -3.421874999385537741 ) ) ;
#35690=VECTOR ( 'NONE', #26153, 1000.000000000000000 ) ;
#35704=CARTESIAN_POINT ( 'NONE',  ( 22.56230152254411436, 3.464101615137759271, -0.1875000000000489608 ) ) ;
#35709=CARTESIAN_POINT ( 'NONE',  ( 13.56230152254410548, 5.196152422706630247, -8.512499998770989507 ) ) ;
#35719=ORIENTED_EDGE ( 'NONE', *, *, #33134, .F. ) ;
#35723=CARTESIAN_POINT ( 'NONE',  ( 10.31873187879411091, 3.604726614523236616, -7.828124999385535965 ) ) ;
#35725=CARTESIAN_POINT ( 'NONE',  ( 10.56230152254411081, 0.000000000000000000, -2.587499998771031429 ) ) ;
#35738=DIRECTION ( 'NONE',  ( 0.000000000000000000, 0.000000000000000000, 1.000000000000000000 ) ) ;
#35759=CARTESIAN_POINT ( 'NONE',  ( 19.68408634441910365, 5.407089921784857367, -3.440624999385522020 ) ) ;
#35763=CARTESIAN_POINT ( 'NONE',  ( 19.68408634441910721, 5.407089921784862696, -9.796874999385529748 ) ) ;
#35777=EDGE_CURVE ( 'NONE', #34717, #27686, #15155, .T. ) ;
#35790=DIRECTION ( 'NONE',  ( 0.000000000000000000, 0.000000000000000000, 1.000000000000000000 ) ) ;
#35792=CARTESIAN_POINT ( 'NONE',  ( 16.56230152254411081, 7.209453229046475009, -8.353124999385524774 ) ) ;
#35799=CARTESIAN_POINT ( 'NONE',  ( 22.56230152254410370, 7.347880794884117764E-16, -5.062499998771007981 ) ) ;
#35802=CARTESIAN_POINT ( 'NONE',  ( 10.31873187879410558, 0.000000000000000000, -4.246874999385502392 ) ) ;
#35804=CARTESIAN_POINT ( 'NONE',  ( 22.56230152254451937, 3.464101615137510137, -7.274999998771029652 ) ) ;
#35833=CARTESIAN_POINT ( 'NONE',  ( 16.56230152254411436, -7.209453229046482114, -7.284374999385498484 ) ) ;
#35840=CARTESIAN_POINT ( 'NONE',  ( 22.56230152254410726, 7.347880794884117764E-16, -9.562499998771039955 ) ) ;
#35852=CARTESIAN_POINT ( 'NONE',  ( 22.56230152254411792, 3.464101615137759271, -7.837500000000039435 ) ) ;
#35856=CARTESIAN_POINT ( 'NONE',  ( 10.56230152254305565, -3.464101615137144652, -6.149999998771001231 ) ) ;
#35863=DIRECTION ( 'NONE',  ( 0.000000000000000000, 0.000000000000000000, 1.000000000000000000 ) ) ;
#35868=CARTESIAN_POINT ( 'NONE',  ( 13.44051670066911441, -5.407089921784865361, -4.621874999385545024 ) ) ;
#35893=FACE_OUTER_BOUND ( 'NONE', #28754, .T. ) ;
#35910=CARTESIAN_POINT ( 'NONE',  ( 13.44051670066911619, -5.407089921784859143, -7.715624999385550353 ) ) ;
#35912=CARTESIAN_POINT ( 'NONE',  ( 22.56230152254410370, 0.000000000000000000, -10.00000000000000000 ) ) ;
#35916=ORIENTED_EDGE ( 'NONE', *, *, #20101, .T. ) ;
#35920=CARTESIAN_POINT ( 'NONE',  ( 10.56230152254410548, 0.000000000000000000, -9.450000000000041922 ) ) ;
#35936=CARTESIAN_POINT ( 'NONE',  ( 16.56230152254410726, 0.000000000000000000, 0.000000000000000000 ) ) ;
#35945=STYLED_ITEM('',(#37528),#7886);
#35949=CARTESIAN_POINT ( 'NONE',  ( 22.80587116629410716, 7.646167579472015790E-16, -4.865624999385531169 ) ) ;
#35951=CARTESIAN_POINT ( 'NONE',  ( 10.56230152254410903, 7.347880794884117764E-16, -10.00000000000000000 ) ) ;
#35968=( BOUNDED_CURVE ( )  B_SPLINE_CURVE ( 2, ( #18670, #18102, #24154, #831, #27177, #29829, #1201 ),
 .UNSPECIFIED., .F., .F. ) 
 B_SPLINE_CURVE_WITH_KNOTS ( ( 3, 2, 2, 3 ),
 ( 0.04347826086956579211, 0.05072463768116096394, 0.05797101449275612883, 0.06521739130435129372 ),
 .UNSPECIFIED. ) 
 CURVE ( )  GEOMETRIC_REPRESENTATION_ITEM ( )  RATIONAL_B_SPLINE_CURVE ( ( 0.9999999999999893419, 0.8660254037844493658, 1.000000000000000000, 0.8660254037844387076, 1.000000000000000000, 0.8660254037843745367, 1.000000000000064171 ) ) 
 REPRESENTATION_ITEM ( '' )  );
#35972=ORIENTED_EDGE ( 'NONE', *, *, #31917, .T. ) ;
#35974=CARTESIAN_POINT ( 'NONE',  ( 19.56230152254411436, -5.196152422706629359, -9.187499998771025744 ) ) ;
#35983=CARTESIAN_POINT ( 'NONE',  ( 22.80587116629410716, 7.646167579472015790E-16, -8.465624999385523708 ) ) ;
#35988=CARTESIAN_POINT ( 'NONE',  ( 19.56230152254411792, -5.196152422706629359, -7.387499998771030363 ) ) ;
#35990=CARTESIAN_POINT ( 'NONE',  ( 22.56230152254410370, 7.347880794884117764E-16, -6.412499998770998744 ) ) ;
#35992=CARTESIAN_POINT ( 'NONE',  ( 10.31873187879411091, -3.604726614523244610, -4.659374999385518024 ) ) ;
#35993=CARTESIAN_POINT ( 'NONE',  ( 10.56230152254426713, -3.464101615137852974, -1.762500000000048139 ) ) ;
#36001=VERTEX_POINT ( 'NONE', #26267 ) ;
#36009=CARTESIAN_POINT ( 'NONE',  ( 10.31873187879411091, -3.604726614523240613, -1.903124999385531924 ) ) ;
#36019=VERTEX_POINT ( 'NONE', #14720 ) ;
#36020=CARTESIAN_POINT ( 'NONE',  ( 10.31873187879410736, 0.000000000000000000, -5.146874999385541827 ) ) ;
#36041=CARTESIAN_POINT ( 'NONE',  ( 19.56230152254412502, -5.196152422706635576, -7.500000000000062172 ) ) ;
#36045=CARTESIAN_POINT ( 'NONE',  ( 10.31873187879410914, 0.000000000000000000, -0.1968749993855323233 ) ) ;
#36049=CARTESIAN_POINT ( 'NONE',  ( 22.46128102716605923, 1.096376214649937619, -10.00000000000000000 ) ) ;
#36053=VERTEX_POINT ( 'NONE', #23436 ) ;
#36057=CARTESIAN_POINT ( 'NONE',  ( 22.80587116629411781, -3.604726614523238837, -4.959374999385524951 ) ) ;
#36081=CARTESIAN_POINT ( 'NONE',  ( 10.56230152254410370, 3.464101615137757051, -0.03749999999999697325 ) ) ;
#36086=CARTESIAN_POINT ( 'NONE',  ( 18.06230152254410726, 1.836970198721030427E-16, 10.00000000000000000 ) ) ;
#36091=LINE ( 'NONE', #6732, #11128 ) ;
#36099=CARTESIAN_POINT ( 'NONE',  ( 22.80587116629410360, -3.604726614523235284, -6.253124999385533123 ) ) ;
#36106=ORIENTED_EDGE ( 'NONE', *, *, #30952, .F. ) ;
#36136=CARTESIAN_POINT ( 'NONE',  ( 10.31873187879411091, -3.604726614523240613, -3.253124999385518912 ) ) ;
#36140=CARTESIAN_POINT ( 'NONE',  ( 16.56230152254411792, 7.209453229046482114, -9.759374999385554972 ) ) ;
#36144=FACE_OUTER_BOUND ( 'NONE', #22883, .T. ) ;
#36151=CARTESIAN_POINT ( 'NONE',  ( 22.56230152254386923, 3.464101615137892942, -4.124999998771019527 ) ) ;
#36164=CARTESIAN_POINT ( 'NONE',  ( 22.80587116629411071, -3.604726614523235284, -7.153124999385557459 ) ) ;
#36170=CARTESIAN_POINT ( 'NONE',  ( 10.56230152254411436, -3.464101615137757051, -7.949999998771033916 ) ) ;
#36173=CARTESIAN_POINT ( 'NONE',  ( 10.31873187879410736, 0.000000000000000000, -5.596874999385520688 ) ) ;
#36176=CARTESIAN_POINT ( 'NONE',  ( 10.56230152254410903, 7.347880794884117764E-16, -10.00000000000000000 ) ) ;
#36181=CARTESIAN_POINT ( 'NONE',  ( 22.56230152254361698, 3.464101615138050150, -3.337500000000045208 ) ) ;
#36193=ORIENTED_EDGE ( 'NONE', *, *, #4615, .T. ) ;
#36200=VECTOR ( 'NONE', #24356, 1000.000000000000000 ) ;
#36202=CARTESIAN_POINT ( 'NONE',  ( 13.44051670066911086, 5.407089921784862696, -6.121874999385518379 ) ) ;
#36206=CARTESIAN_POINT ( 'NONE',  ( 10.31873187879410914, 0.000000000000000000, -0.5906249993855583469 ) ) ;
#36211=( LENGTH_UNIT ( ) NAMED_UNIT ( * ) SI_UNIT ( .MILLI., .METRE. ) );
#36212=CARTESIAN_POINT ( 'NONE',  ( 19.56230152254410370, 5.196152422706631135, -2.737499998770986931 ) ) ;
#36215=CARTESIAN_POINT ( 'NONE',  ( 14.39393461504979399, 5.957546011302761180, -10.18332779764974383 ) ) ;
#36225=CARTESIAN_POINT ( 'NONE',  ( 10.56230152254410548, 0.000000000000000000, -9.000000000000035527 ) ) ;
#36241=CARTESIAN_POINT ( 'NONE',  ( 22.80587116629411781, 7.646167579472024665E-16, -5.371874999385517491 ) ) ;
#36264=CARTESIAN_POINT ( 'NONE',  ( 22.56230152254412147, 3.464101615137759271, -3.337500000000051426 ) ) ;
#36269=CARTESIAN_POINT ( 'NONE',  ( 19.56230152254410370, 5.196152422706631135, -8.587499998771008336 ) ) ;
#36277=CARTESIAN_POINT ( 'NONE',  ( 10.56230152254474497, -3.464101615138128754, -7.162500000000022737 ) ) ;
#36278=DIRECTION ( 'NONE',  ( 1.000000000000000000, 0.000000000000000000, 0.000000000000000000 ) ) ;
#36280=CARTESIAN_POINT ( 'NONE',  ( 22.80587116629410360, 7.646167579472015790E-16, -6.665624999385527438 ) ) ;
#36295=CARTESIAN_POINT ( 'NONE',  ( 22.56230152254576993, -3.464101615136805368, -5.662500000000002309 ) ) ;
#36318=CARTESIAN_POINT ( 'NONE',  ( 13.44051670066911797, -5.407089921784859143, -3.665624999385552751 ) ) ;
#36320=CARTESIAN_POINT ( 'NONE',  ( 22.56230152254464727, -3.464101615137448409, -7.462500000000031442 ) ) ;
#36324=CARTESIAN_POINT ( 'NONE',  ( 16.56230152254411792, -6.928203230275514990, -8.437500000000024869 ) ) ;
#36327=CARTESIAN_POINT ( 'NONE',  ( 13.44051670066911441, -5.407089921784865361, -1.021874999385524729 ) ) ;
#36330=VERTEX_POINT ( 'NONE', #9218 ) ;
#36346=AXIS2_PLACEMENT_3D ( 'NONE', #4769, #36786, #22033 ) ;
#36350=CARTESIAN_POINT ( 'NONE',  ( 22.80587116629410716, 3.604726614523238837, -7.528124999385559235 ) ) ;
#36356=CARTESIAN_POINT ( 'NONE',  ( 22.56230152254411436, -3.464101615137751278, -8.699999998771005494 ) ) ;
#36360=CARTESIAN_POINT ( 'NONE',  ( 22.80587116629411781, 7.646167579472024665E-16, -5.371874999385517491 ) ) ;
#36367=CARTESIAN_POINT ( 'NONE',  ( 13.56230152254410903, 5.196152422706636465, -3.225000000000033396 ) ) ;
#36377=CARTESIAN_POINT ( 'NONE',  ( 13.56230152254411614, -5.196152422706632912, -7.012499998771043686 ) ) ;
#36389=CARTESIAN_POINT ( 'NONE',  ( 16.56230152254411081, -7.209453229046482114, -9.084374999385513405 ) ) ;
#36393=CARTESIAN_POINT ( 'NONE',  ( 22.80587116629411071, -3.604726614523235284, -1.303124999385484095 ) ) ;
#36397=CARTESIAN_POINT ( 'NONE',  ( 10.56230152254411081, 0.000000000000000000, -2.587499998771031429 ) ) ;
#36400=CARTESIAN_POINT ( 'NONE',  ( 13.56230152254410548, 5.196152422706630247, -2.212499998771017218 ) ) ;
#36408=CARTESIAN_POINT ( 'NONE',  ( 16.56230152254411436, -6.928203230275514990, -9.787500000000044054 ) ) ;
#36410=CARTESIAN_POINT ( 'NONE',  ( 10.56230152254410726, 0.000000000000000000, -8.100000000000024514 ) ) ;
#36418=CARTESIAN_POINT ( 'NONE',  ( 19.56230152254410726, 5.196152422706631135, -6.787499998771012955 ) ) ;
#36422=AXIS2_PLACEMENT_3D ( 'NONE', #1265, #20819, #3927 ) ;
#36425=CARTESIAN_POINT ( 'NONE',  ( 10.31873187879410736, -3.604726614523244610, -6.459374999385468996 ) ) ;
#36437=( BOUNDED_CURVE ( )  B_SPLINE_CURVE ( 2, ( #8825, #20579, #3128, #23050, #29086, #34781, #34594 ),
 .UNSPECIFIED., .F., .F. ) 
 B_SPLINE_CURVE_WITH_KNOTS ( ( 3, 2, 2, 3 ),
 ( 0.8260869565217369148, 0.8333333333333312609, 0.8405797101449254960, 0.8478260869565198421 ),
 .UNSPECIFIED. ) 
 CURVE ( )  GEOMETRIC_REPRESENTATION_ITEM ( )  RATIONAL_B_SPLINE_CURVE ( ( 1.000000000000041078, 0.8660254037843976294, 1.000000000000000000, 0.8660254037844387076, 1.000000000000000000, 0.8660254037844735686, 0.9999999999999651390 ) ) 
 REPRESENTATION_ITEM ( '' )  );
#36442=CARTESIAN_POINT ( 'NONE',  ( 10.56230152254410903, 0.000000000000000000, -1.687499998771019305 ) ) ;
#36450=CARTESIAN_POINT ( 'NONE',  ( 22.56230152254412147, -3.464101615137755275, -1.162500000000034284 ) ) ;
#36452=ORIENTED_EDGE ( 'NONE', *, *, #8477, .F. ) ;
#36465=CARTESIAN_POINT ( 'NONE',  ( 22.56230152254411792, 7.347880794884125653E-16, -2.025000000000027001 ) ) ;
#36467=CARTESIAN_POINT ( 'NONE',  ( 22.80587116629411071, -3.604726614523235284, -9.403124999385536142 ) ) ;
#36475=ORIENTED_EDGE ( 'NONE', *, *, #5656, .F. ) ;
#36506=CARTESIAN_POINT ( 'NONE',  ( 13.44051670066911086, 5.407089921784856479, -6.965624999385521932 ) ) ;
#36513=CARTESIAN_POINT ( 'NONE',  ( 16.56230152254411792, 6.928203230275514990, -6.862500000000054889 ) ) ;
#36515=CARTESIAN_POINT ( 'NONE',  ( 16.56230152254412147, -7.209453229046482114, -0.9843749993855260838 ) ) ;
#36538=CARTESIAN_POINT ( 'NONE',  ( 13.44051670066911086, 5.407089921784856479, -6.965624999385521932 ) ) ;
#36543=CARTESIAN_POINT ( 'NONE',  ( 22.56230152254411436, -3.464101615137751278, -7.799999998771014020 ) ) ;
#36548=CARTESIAN_POINT ( 'NONE',  ( 10.31873187879411091, -3.604726614523244610, -5.559374999385509497 ) ) ;
#36569=EDGE_CURVE ( 'NONE', #19865, #21112, #24749, .T. ) ;
#36578=CARTESIAN_POINT ( 'NONE',  ( 16.56230152254411792, 7.209453229046482114, -8.859374999385531524 ) ) ;
#36582=CARTESIAN_POINT ( 'NONE',  ( 16.56230152254411436, -7.209453229046475009, -0.4781249993855187230 ) ) ;
#36586=( NAMED_UNIT ( * ) SI_UNIT ( $, .STERADIAN. ) SOLID_ANGLE_UNIT ( ) );
#36590=CARTESIAN_POINT ( 'NONE',  ( 22.56230152254410370, -3.464101615137751278, -0.5999999987710181726 ) ) ;
#36592=CARTESIAN_POINT ( 'NONE',  ( 10.56230152254410903, 7.347880794884117764E-16, -10.00000000000000000 ) ) ;
#36597=CARTESIAN_POINT ( 'NONE',  ( 14.47852554861151830, 5.725134610794655465, -9.986452800325864132 ) ) ;
#36606=DIRECTION ( 'NONE',  ( -0.2588190451025212391, 0.000000000000000000, -0.9659258262890682012 ) ) ;
#36613=CARTESIAN_POINT ( 'NONE',  ( 19.68408634441911431, 5.407089921784862696, -5.296874999385526195 ) ) ;
#36619=CARTESIAN_POINT ( 'NONE',  ( 22.80587116629411781, 3.604726614523243278, -0.3843749993855423708 ) ) ;
#36622=CIRCLE ( 'NONE', #22743, 8.000000000000000000 ) ;
#36630=EDGE_CURVE ( 'NONE', #9264, #28127, #28142, .T. ) ;
#36639=CARTESIAN_POINT ( 'NONE',  ( 19.56230152254411792, 5.196152422706637353, -2.400000000000013234 ) ) ;
#36650=AXIS2_PLACEMENT_3D ( 'NONE', #25417, #31294, #22588 ) ;
#36659=CARTESIAN_POINT ( 'NONE',  ( 19.68408634441910721, -5.407089921784855591, -8.990624999385548932 ) ) ;
#36670=( BOUNDED_CURVE ( )  B_SPLINE_CURVE ( 2, ( #15508, #32932, #6984, #18553, #25336, #24593, #10930 ),
 .UNSPECIFIED., .F., .F. ) 
 B_SPLINE_CURVE_WITH_KNOTS ( ( 3, 2, 2, 3 ),
 ( 0.1739130434782605317, 0.1811594202898539063, 0.1884057971014473087, 0.1956521739130406834 ),
 .UNSPECIFIED. ) 
 CURVE ( )  GEOMETRIC_REPRESENTATION_ITEM ( )  RATIONAL_B_SPLINE_CURVE ( ( 1.000000000000006217, 0.8660254037844326014, 1.000000000000000000, 0.8660254037844387076, 1.000000000000000000, 0.8660254037844905550, 0.9999999999999481526 ) ) 
 REPRESENTATION_ITEM ( '' )  );
#36695=CARTESIAN_POINT ( 'NONE',  ( 10.31873187879410736, 0.000000000000000000, -6.440624999385525129 ) ) ;
#36705=CARTESIAN_POINT ( 'NONE',  ( 16.56230152254411436, 7.209453229046482114, -0.3093749993854842950 ) ) ;
#36711=CARTESIAN_POINT ( 'NONE',  ( 10.31873187879411091, 0.000000000000000000, -1.940624999385548444 ) ) ;
#36728=CARTESIAN_POINT ( 'NONE',  ( 16.56230152254410726, 7.209453229046475009, -9.253124999385514471 ) ) ;
#36733=CARTESIAN_POINT ( 'NONE',  ( 19.56230152254411081, -5.196152422706629359, -9.637499998771032139 ) ) ;
#36737=CARTESIAN_POINT ( 'NONE',  ( 13.44051670066910731, 5.407089921784862696, -10.17187499938551554 ) ) ;
#36738=CARTESIAN_POINT ( 'NONE',  ( 19.68408634441911431, 5.407089921784862696, -6.646874999385543603 ) ) ;
#36744=DIRECTION ( 'NONE',  ( 0.000000000000000000, 0.000000000000000000, 1.000000000000000000 ) ) ;
#36766=CARTESIAN_POINT ( 'NONE',  ( 13.44051670066911264, -5.407089921784865361, -8.671874999385515537 ) ) ;
#36774=CARTESIAN_POINT ( 'NONE',  ( 22.56230152254410370, 7.347880794884117764E-16, -1.012499998771038134 ) ) ;
#36782=CARTESIAN_POINT ( 'NONE',  ( 19.56230152254411792, 5.196152422706637353, -9.150000000000046541 ) ) ;
#36786=DIRECTION ( 'NONE',  ( 0.000000000000000000, 0.000000000000000000, 1.000000000000000000 ) ) ;
#36793=CARTESIAN_POINT ( 'NONE',  ( 10.56230152254410726, 0.000000000000000000, -6.637499998771001941 ) ) ;
#36799=CARTESIAN_POINT ( 'NONE',  ( 13.44051670066911086, 5.407089921784862696, -5.671874999385540406 ) ) ;
#36804=ORIENTED_EDGE ( 'NONE', *, *, #6243, .T. ) ;
#36806=CARTESIAN_POINT ( 'NONE',  ( 22.80587116629411426, -3.604726614523238837, -1.809374999385491511 ) ) ;
#36812=CARTESIAN_POINT ( 'NONE',  ( 10.56230152254450161, 3.464101615137985757, -2.737500000000008260 ) ) ;
#36817=FACE_OUTER_BOUND ( 'NONE', #11239, .T. ) ;
#36822=( BOUNDED_CURVE ( )  B_SPLINE_CURVE ( 2, ( #12241, #12622, #32705, #1049, #3899, #9593, #24002 ),
 .UNSPECIFIED., .F., .F. ) 
 B_SPLINE_CURVE_WITH_KNOTS ( ( 3, 2, 2, 3 ),
 ( 0.3695652173913038796, 0.3768115942028982257, 0.3840579710144925163, 0.3913043478260868624 ),
 .UNSPECIFIED. ) 
 CURVE ( )  GEOMETRIC_REPRESENTATION_ITEM ( )  RATIONAL_B_SPLINE_CURVE ( ( 1.000000000000008216, 0.8660254037844304920, 1.000000000000000000, 0.8660254037844387076, 1.000000000000000000, 0.8660254037844407060, 0.9999999999999980016 ) ) 
 REPRESENTATION_ITEM ( '' )  );
#36825=CARTESIAN_POINT ( 'NONE',  ( 10.56230152254410726, -3.464101615137761048, -1.762500000000049916 ) ) ;
#36837=ORIENTED_EDGE ( 'NONE', *, *, #30706, .T. ) ;
#36842=CARTESIAN_POINT ( 'NONE',  ( 22.80587116629410716, 7.646167579472015790E-16, -9.365624999385563143 ) ) ;
#36847=EDGE_LOOP ( 'NONE', ( #34476, #37157, #32030, #5108 ) ) ;
#36875=CARTESIAN_POINT ( 'NONE',  ( 10.31873187879411269, -3.604726614523240613, -6.403124999385521043 ) ) ;
#36884=CARTESIAN_POINT ( 'NONE',  ( 22.80587116629412847, 3.604726614523243278, -1.734374999385497551 ) ) ;
#36891=CARTESIAN_POINT ( 'NONE',  ( 13.44051670066911441, -5.407089921784859143, -2.315624999385534899 ) ) ;
#36904=CARTESIAN_POINT ( 'NONE',  ( 11.28998163430637725, -3.344369132205555317, -9.999999999999998224 ) ) ;
#36906=VECTOR ( 'NONE', #9717, 1000.000000000000000 ) ;
#36911=EDGE_CURVE ( 'NONE', #11078, #24827, #12502, .T. ) ;
#36914=CARTESIAN_POINT ( 'NONE',  ( 19.68408634441911431, -5.407089921784861808, -9.946874999385540761 ) ) ;
#36915=CARTESIAN_POINT ( 'NONE',  ( 22.80587116629411426, 7.646167579472024665E-16, -6.721874999385535787 ) ) ;
#36916=DIRECTION ( 'NONE',  ( 0.000000000000000000, 0.000000000000000000, 1.000000000000000000 ) ) ;
#36920=CARTESIAN_POINT ( 'NONE',  ( 16.56230152254411792, 6.928203230275514990, -5.962500000000031442 ) ) ;
#36924=FACE_OUTER_BOUND ( 'NONE', #30095, .T. ) ;
#36940=ORIENTED_EDGE ( 'NONE', *, *, #29389, .F. ) ;
#36945=CARTESIAN_POINT ( 'NONE',  ( 10.56230152254410726, 0.000000000000000000, -9.900000000000048317 ) ) ;
#36947=CARTESIAN_POINT ( 'NONE',  ( 19.68408634441910721, 5.407089921784862696, -8.896874999385516958 ) ) ;
#36950=CARTESIAN_POINT ( 'NONE',  ( 22.80587116629411071, 3.604726614523238837, -2.128124999385546001 ) ) ;
#36958=CARTESIAN_POINT ( 'NONE',  ( 22.56230152254410370, 3.464101615137755275, -1.424999998770983600 ) ) ;
#36969=CARTESIAN_POINT ( 'NONE',  ( 22.80587116629410360, -3.604726614523235284, -0.4031249993855248182 ) ) ;
#36970=CARTESIAN_POINT ( 'NONE',  ( 22.56230152254410726, 7.347880794884117764E-16, -9.112499998771033560 ) ) ;
#36974=CARTESIAN_POINT ( 'NONE',  ( 10.56230152254521037, 3.464101615138387658, -2.174999998771001142 ) ) ;
#36979=DIRECTION ( 'NONE',  ( 0.000000000000000000, 0.000000000000000000, 1.000000000000000000 ) ) ;
#36986=CARTESIAN_POINT ( 'NONE',  ( 13.44051670066911086, 5.407089921784862696, -6.121874999385518379 ) ) ;
#36991=CARTESIAN_POINT ( 'NONE',  ( 22.80587116629411781, 7.646167579472024665E-16, -0.8718749993855412495 ) ) ;
#36996=CARTESIAN_POINT ( 'NONE',  ( 22.56230152254412502, 7.347880794884125653E-16, -2.925000000000066436 ) ) ;
#37009=CARTESIAN_POINT ( 'NONE',  ( 13.56230152254411436, -5.196152422706638241, -2.625000000000043965 ) ) ;
#37026=CARTESIAN_POINT ( 'NONE',  ( 13.44051670066910908, 5.407089921784856479, -10.11562499938553650 ) ) ;
#37062=CARTESIAN_POINT ( 'NONE',  ( 22.80587116629411071, -3.604726614523235284, -5.803124999385537386 ) ) ;
#37071=CARTESIAN_POINT ( 'NONE',  ( 16.56230152254411436, 7.209453229046482114, -2.559374999385494842 ) ) ;
#37072=LINE ( 'NONE', #25889, #22117 ) ;
#37076=CARTESIAN_POINT ( 'NONE',  ( 10.56230152254410903, 0.000000000000000000, -3.937499998770993770 ) ) ;
#37078=CARTESIAN_POINT ( 'NONE',  ( 13.44051670066911441, 5.407089921784856479, -2.465624999385545912 ) ) ;
#37081=DIRECTION ( 'NONE',  ( 0.000000000000000000, 0.000000000000000000, 1.000000000000000000 ) ) ;
#37094=CARTESIAN_POINT ( 'NONE',  ( 13.44051670066911619, -5.407089921784859143, -9.515624999385547511 ) ) ;
#37100=CARTESIAN_POINT ( 'NONE',  ( 22.56230152254411436, -3.464101615137751278, -10.04999999877099270 ) ) ;
#37102=CYLINDRICAL_SURFACE ( 'NONE', #13250, 5.999999999999998224 ) ;
#37104=CARTESIAN_POINT ( 'NONE',  ( 22.80587116629411781, -3.604726614523238837, -9.909374999385510918 ) ) ;
#37105=( BOUNDED_CURVE ( )  B_SPLINE_CURVE ( 2, ( #9476, #12508, #15352, #32402, #23694, #35804, #742 ),
 .UNSPECIFIED., .F., .F. ) 
 B_SPLINE_CURVE_WITH_KNOTS ( ( 3, 2, 2, 3 ),
 ( 0.6521739130434789367, 0.6594202898550732828, 0.6666666666666674068, 0.6739130434782617529 ),
 .UNSPECIFIED. ) 
 CURVE ( )  GEOMETRIC_REPRESENTATION_ITEM ( )  RATIONAL_B_SPLINE_CURVE ( ( 0.9999999999999876765, 0.8660254037844510311, 1.000000000000000000, 0.8660254037844387076, 1.000000000000000000, 0.8660254037844222763, 1.000000000000016431 ) ) 
 REPRESENTATION_ITEM ( '' )  );
#37106=CARTESIAN_POINT ( 'NONE',  ( 22.80587116629412137, 7.646167579472024665E-16, -9.421874999385515537 ) ) ;
#37112=DIRECTION ( 'NONE',  ( 0.000000000000000000, 0.000000000000000000, 1.000000000000000000 ) ) ;
#37122=EDGE_CURVE ( 'NONE', #26922, #23387, #20259, .T. ) ;
#37131=CARTESIAN_POINT ( 'NONE',  ( 10.56230152254423693, 3.464101615137833434, -2.287500000000041389 ) ) ;
#37134=CARTESIAN_POINT ( 'NONE',  ( 19.68408634441911786, -5.407089921784861808, -8.596874999385523353 ) ) ;
#37137=CARTESIAN_POINT ( 'NONE',  ( 22.80587116629411426, -3.604726614523235284, -3.103124999385562521 ) ) ;
#37142=DIRECTION ( 'NONE',  ( 1.000000000000000000, 0.000000000000000000, 0.000000000000000000 ) ) ;
#37145=CARTESIAN_POINT ( 'NONE',  ( 16.56230152254411081, 6.928203230275506996, -4.049999998770996257 ) ) ;
#37155=CARTESIAN_POINT ( 'NONE',  ( 13.44051670066911264, 5.407089921784856479, -1.115624999385556038 ) ) ;
#37157=ORIENTED_EDGE ( 'NONE', *, *, #23535, .T. ) ;
#37161=COLOUR_RGB ( '',0.8941176470588234615, 0.8941176470588234615, 0.8941176470588234615 ) ;
#37166=CARTESIAN_POINT ( 'NONE',  ( 22.56230152254278920, -3.464101615138517332, -8.699999998771023257 ) ) ;
#37170=ORIENTED_EDGE ( 'NONE', *, *, #9417, .F. ) ;
#37173=CARTESIAN_POINT ( 'NONE',  ( 10.31873187879410381, -3.604726614523244610, -7.809374999385488181 ) ) ;
#37178=CARTESIAN_POINT ( 'NONE',  ( 22.80587116629411781, 3.604726614523243278, -0.8343749993855380520 ) ) ;
#37183=CARTESIAN_POINT ( 'NONE',  ( 10.56230152254410903, 0.000000000000000000, -2.700000000000063238 ) ) ;
#37194=CARTESIAN_POINT ( 'NONE',  ( 10.56230152254410903, -3.464101615137761048, -4.912500000000052047 ) ) ;
#37213=CARTESIAN_POINT ( 'NONE',  ( 10.31873187879411091, -3.604726614523240613, -9.103124999385528326 ) ) ;
#37218=ORIENTED_EDGE ( 'NONE', *, *, #15285, .T. ) ;
#37236=CARTESIAN_POINT ( 'NONE',  ( 10.56230152254458865, -3.464101615138036827, -5.362500000000041567 ) ) ;
#37244=CARTESIAN_POINT ( 'NONE',  ( 19.56230152254412147, -5.196152422706635576, -0.7500000000000839329 ) ) ;
#37248=CARTESIAN_POINT ( 'NONE',  ( 16.56230152254410726, -7.209453229046475009, -6.778124999385522820 ) ) ;
#37258=EDGE_LOOP ( 'NONE', ( #11161, #31353, #27858, #27371 ) ) ;
#37263=CARTESIAN_POINT ( 'NONE',  ( 13.44051670066911264, 5.407089921784856479, -1.115624999385556038 ) ) ;
#37269=ORIENTED_EDGE ( 'NONE', *, *, #15863, .F. ) ;
#37275=VECTOR ( 'NONE', #14734, 1000.000000000000000 ) ;
#37281=CARTESIAN_POINT ( 'NONE',  ( 10.31873187879410736, -3.604726614523240613, -9.553124999385522287 ) ) ;
#37285=CIRCLE ( 'NONE', #28812, 1.500000000000001332 ) ;
#37292=CARTESIAN_POINT ( 'NONE',  ( 22.80587116629411781, -3.604726614523238837, -9.909374999385510918 ) ) ;
#37298=CARTESIAN_POINT ( 'NONE',  ( 22.56230152254484977, 3.464101615137326728, -3.674999998771035781 ) ) ;
#37311=VERTEX_POINT ( 'NONE', #12274 ) ;
#37313=VECTOR ( 'NONE', #13891, 1000.000000000000000 ) ;
#37314=CARTESIAN_POINT ( 'NONE',  ( 10.56230152254397758, -3.464101615137684664, -2.212500000000047429 ) ) ;
#37320=CARTESIAN_POINT ( 'NONE',  ( 22.80587116629410716, 3.604726614523238837, -2.578124999385541738 ) ) ;
#37325=CARTESIAN_POINT ( 'NONE',  ( 13.56230152254411792, -5.196152422706632912, -3.862499998771057541 ) ) ;
#37334=CARTESIAN_POINT ( 'NONE',  ( 19.56230152254410370, 5.196152422706631135, -9.037499998771014731 ) ) ;
#37339=CARTESIAN_POINT ( 'NONE',  ( 22.56230152254410370, 0.000000000000000000, -10.00000000000000000 ) ) ;
#37350=CARTESIAN_POINT ( 'NONE',  ( 22.80587116629411426, 7.646167579472024665E-16, -7.621874999385519267 ) ) ;
#37354=CARTESIAN_POINT ( 'NONE',  ( 22.80587116629411426, 7.646167579472024665E-16, -1.771874999385525395 ) ) ;
#37362=( BOUNDED_CURVE ( )  B_SPLINE_CURVE ( 2, ( #8741, #34143, #19945, #28818, #8553, #23333, #20312 ),
 .UNSPECIFIED., .F., .F. ) 
 B_SPLINE_CURVE_WITH_KNOTS ( ( 3, 2, 2, 3 ),
 ( 0.5000000000000012212, 0.5072463768115955673, 0.5144927536231899134, 0.5217391304347842595 ),
 .UNSPECIFIED. ) 
 CURVE ( )  GEOMETRIC_REPRESENTATION_ITEM ( )  RATIONAL_B_SPLINE_CURVE ( ( 0.9999999999999774625, 0.8660254037844612451, 1.000000000000000000, 0.8660254037844387076, 1.000000000000000000, 0.8660254037844079544, 1.000000000000030864 ) ) 
 REPRESENTATION_ITEM ( '' )  );
#37364=ADVANCED_FACE ( 'NONE', ( #6212, #8685 ), #14935, .F. ) ;
#37374=CARTESIAN_POINT ( 'NONE',  ( 22.56230152254412147, 3.464101615137759271, -4.237500000000042455 ) ) ;
#37378=CARTESIAN_POINT ( 'NONE',  ( 10.56230152254411259, -3.464101615137757051, -6.599999998771014731 ) ) ;
#37394=CARTESIAN_POINT ( 'NONE',  ( 13.44051670066911086, 5.407089921784862696, -1.171874999385535965 ) ) ;
#37417=CARTESIAN_POINT ( 'NONE',  ( 22.56230152254410370, 0.000000000000000000, -10.00000000000000000 ) ) ;
#37429=CARTESIAN_POINT ( 'NONE',  ( 13.44051670066911441, -5.407089921784859143, -8.165624999385528326 ) ) ;
#37430=CARTESIAN_POINT ( 'NONE',  ( 22.56230152254410370, 7.347880794884117764E-16, -1.462499998771016330 ) ) ;
#37432=CARTESIAN_POINT ( 'NONE',  ( 10.56230152254410726, 0.000000000000000000, -3.600000000000047606 ) ) ;
#37443=CARTESIAN_POINT ( 'NONE',  ( 10.31873187879411269, -3.604726614523240613, -5.503124999385529570 ) ) ;
#37472=CARTESIAN_POINT ( 'NONE',  ( 10.31873187879410558, 0.000000000000000000, -9.196874999385512339 ) ) ;
#37499=CARTESIAN_POINT ( 'NONE',  ( 10.31873187879410736, 3.604726614523236616, -1.978124999385525662 ) ) ;
#37522=COLOUR_RGB('Light Blue',0.38,0.62,0.78);
#37523=FILL_AREA_STYLE_COLOUR('',#37522);
#37524=FILL_AREA_STYLE('',(#37523));
#37525=SURFACE_STYLE_FILL_AREA(#37524);
#37526=SURFACE_SIDE_STYLE('',(#37525));
#37527=SURFACE_STYLE_USAGE(.BOTH.,#37526);
#37528=PRESENTATION_STYLE_ASSIGNMENT((#37527));
ENDSEC;
END-ISO-10303-21;
